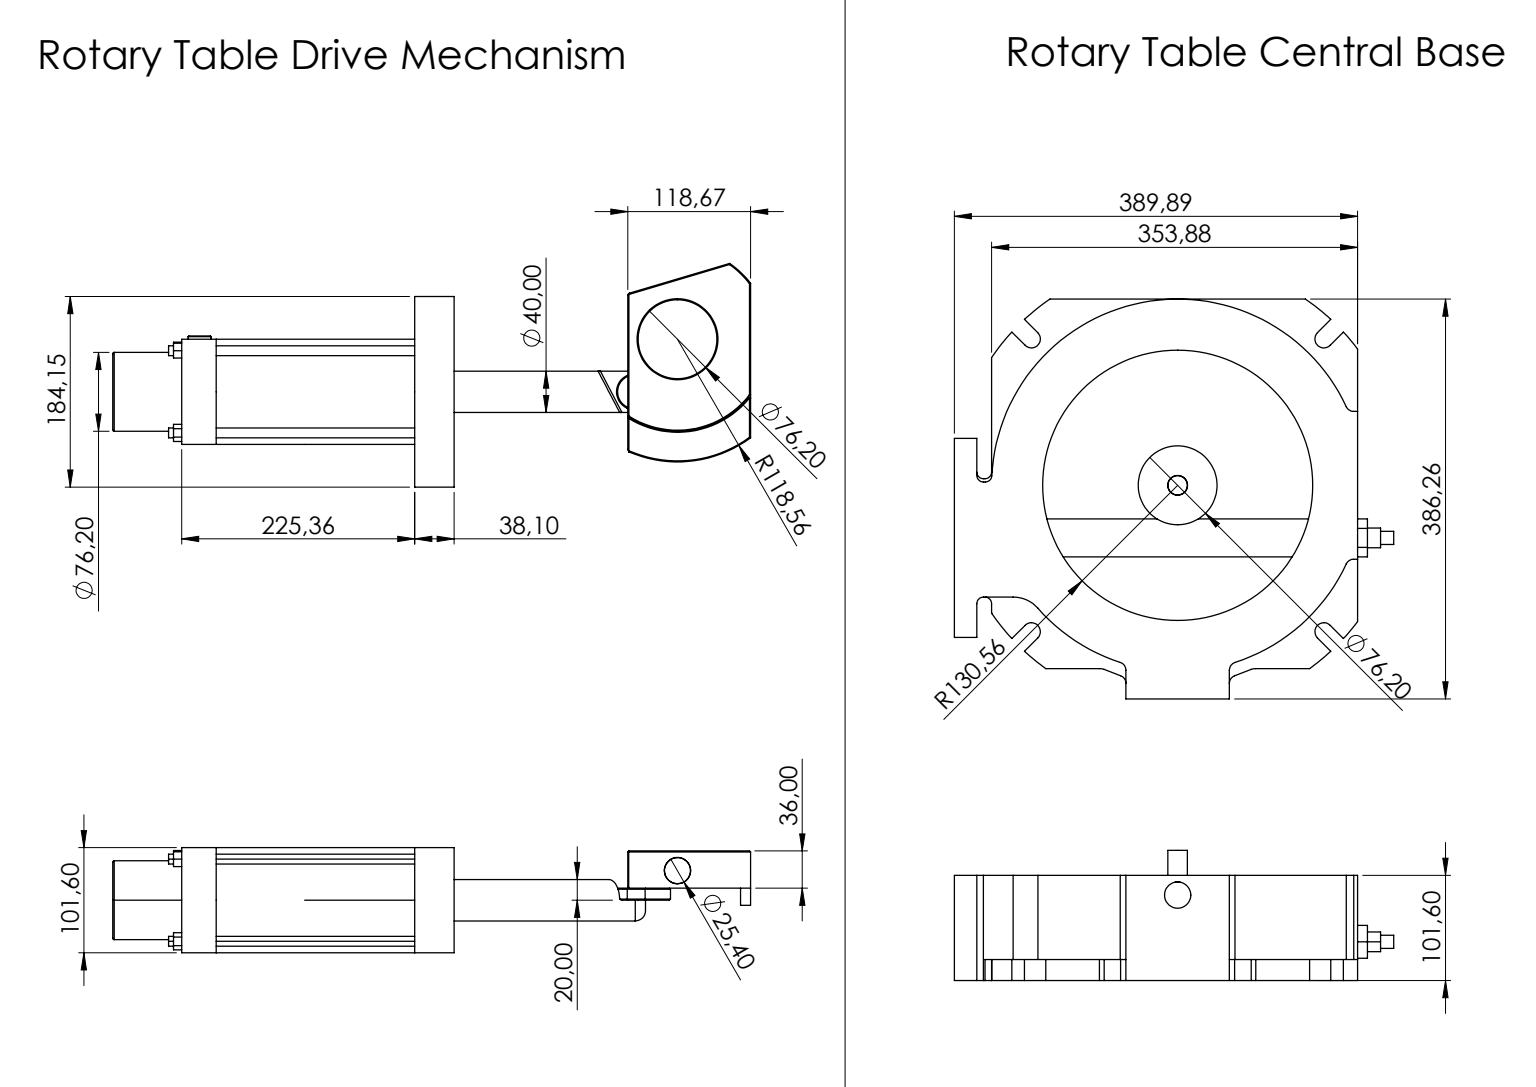
ISO-10303-21;
HEADER;
FILE_DESCRIPTION (('STEP AP214'),
    '1' );
FILE_NAME ('Rotary Table Central Base.step',
    '2026-10-07T11:37:37',
    ( '' ),
    ( '' ),
    'SwSTEP 2.0',
    'SolidWorks 2020',
    '' );
FILE_SCHEMA (( 'AUTOMOTIVE_DESIGN' ));
ENDSEC;

DATA;
#6=CARTESIAN_POINT ( 'NONE',  ( 55.11501535284990183, 101.5999999999999943, 183.9403141659174992 ) ) ;
#9=CARTESIAN_POINT ( 'NONE',  ( 9.168977498726896158, 73.76155057898466794, 130.2336791939843295 ) ) ;
#14=CARTESIAN_POINT ( 'NONE',  ( -194.1576000000000022, 0.000000000000000000, -12.69999999999999929 ) ) ;
#21=ORIENTED_EDGE ( 'NONE', *, *, #73612, .F. ) ;
#33=ORIENTED_EDGE ( 'NONE', *, *, #1736, .F. ) ;
#55=ORIENTED_EDGE ( 'NONE', *, *, #81296, .T. ) ;
#58=DIRECTION ( 'NONE',  ( 0.000000000000000000, -1.000000000000000000, 0.000000000000000000 ) ) ;
#67=DIRECTION ( 'NONE',  ( 0.000000000000000000, -1.000000000000000000, 0.000000000000000000 ) ) ;
#73=FACE_OUTER_BOUND ( 'NONE', #27829, .T. ) ;
#85=DIRECTION ( 'NONE',  ( 0.000000000000000000, 0.000000000000000000, -1.000000000000000000 ) ) ;
#88=CARTESIAN_POINT ( 'NONE',  ( 57.91199999999999903, 20.32000000000000028, 178.6098374884404905 ) ) ;
#95=ORIENTED_EDGE ( 'NONE', *, *, #27973, .F. ) ;
#121=VERTEX_POINT ( 'NONE', #20268 ) ;
#132=VECTOR ( 'NONE', #74907, 1000.000000000000000 ) ;
#135=DIRECTION ( 'NONE',  ( 0.000000000000000000, -1.000000000000000000, 0.000000000000000000 ) ) ;
#144=CARTESIAN_POINT ( 'NONE',  ( 1.925672578516905147E-22, 69.84999999999999432, 130.5560000000000116 ) ) ;
#191=EDGE_CURVE ( 'NONE', #23949, #76533, #47936, .T. ) ;
#205=FACE_OUTER_BOUND ( 'NONE', #10836, .T. ) ;
#234=CARTESIAN_POINT ( 'NONE',  ( -118.6305646578576045, 74.28520294732120988, 54.51736277023807986 ) ) ;
#242=EDGE_CURVE ( 'NONE', #42621, #19042, #11659, .T. ) ;
#255=EDGE_LOOP ( 'NONE', ( #36658, #16819, #37232, #21617 ) ) ;
#262=CARTESIAN_POINT ( 'NONE',  ( 50.03799999999999670, 101.5999999999999943, 206.3750000000000000 ) ) ;
#265=CARTESIAN_POINT ( 'NONE',  ( -6.586072245893089594, 71.69064597417980167, 130.3897833686264676 ) ) ;
#267=DIRECTION ( 'NONE',  ( 0.000000000000000000, 0.000000000000000000, 1.000000000000000000 ) ) ;
#269=LINE ( 'NONE', #28879, #27362 ) ;
#284=FACE_OUTER_BOUND ( 'NONE', #2553, .T. ) ;
#309=ORIENTED_EDGE ( 'NONE', *, *, #18028, .F. ) ;
#321=LINE ( 'NONE', #15311, #8132 ) ;
#341=CARTESIAN_POINT ( 'NONE',  ( -179.8898777604655095, 101.5999999999999943, 114.2999999999999972 ) ) ;
#345=ORIENTED_EDGE ( 'NONE', *, *, #9906, .F. ) ;
#365=EDGE_CURVE ( 'NONE', #79893, #74303, #7526, .T. ) ;
#369=DIRECTION ( 'NONE',  ( 0.000000000000000000, 0.000000000000000000, 1.000000000000000000 ) ) ;
#371=FACE_OUTER_BOUND ( 'NONE', #73680, .T. ) ;
#378=VERTEX_POINT ( 'NONE', #7971 ) ;
#402=CARTESIAN_POINT ( 'NONE',  ( 0.000000000000000000, 8.255000000000000782, 0.000000000000000000 ) ) ;
#409=ADVANCED_FACE ( 'NONE', ( #6043 ), #47786, .F. ) ;
#412=ORIENTED_EDGE ( 'NONE', *, *, #13605, .T. ) ;
#418=LINE ( 'NONE', #69017, #71892 ) ;
#419=VECTOR ( 'NONE', #36946, 1000.000000000000000 ) ;
#424=EDGE_CURVE ( 'NONE', #58432, #84394, #41641, .T. ) ;
#436=ORIENTED_EDGE ( 'NONE', *, *, #26526, .T. ) ;
#447=DIRECTION ( 'NONE',  ( 0.000000000000000000, 1.000000000000000000, 0.000000000000000000 ) ) ;
#456=CARTESIAN_POINT ( 'NONE',  ( 120.0602177517065314, 48.67389603571125178, -51.28856941560783866 ) ) ;
#459=ORIENTED_EDGE ( 'NONE', *, *, #13256, .F. ) ;
#461=EDGE_CURVE ( 'NONE', #89089, #79893, #19649, .T. ) ;
#493=ORIENTED_EDGE ( 'NONE', *, *, #28288, .T. ) ;
#509=PLANE ( 'NONE',  #44376 ) ;
#523=FACE_OUTER_BOUND ( 'NONE', #41384, .T. ) ;
#534=AXIS2_PLACEMENT_3D ( 'NONE', #54365, #54819, #13078 ) ;
#537=AXIS2_PLACEMENT_3D ( 'NONE', #14393, #82553, #62968 ) ;
#572=CARTESIAN_POINT ( 'NONE',  ( -187.8075999999999794, 20.32000000000000028, -12.69999999999999929 ) ) ;
#599=CARTESIAN_POINT ( 'NONE',  ( 11.42157353567683842, 76.98139724742750900, 130.0556313956597592 ) ) ;
#635=DIRECTION ( 'NONE',  ( 1.000000000000000000, 0.000000000000000000, 0.000000000000000000 ) ) ;
#639=ORIENTED_EDGE ( 'NONE', *, *, #3250, .F. ) ;
#656=LINE ( 'NONE', #28362, #8199 ) ;
#675=LINE ( 'NONE', #22483, #55023 ) ;
#679=ORIENTED_EDGE ( 'NONE', *, *, #28156, .T. ) ;
#681=CARTESIAN_POINT ( 'NONE',  ( -114.0590328520549832, 70.22562679785821160, 63.52550556333007137 ) ) ;
#684=CARTESIAN_POINT ( 'NONE',  ( -127.5252020268932114, 20.32000000000000028, 177.0380000000000109 ) ) ;
#710=DIRECTION ( 'NONE',  ( 0.000000000000000000, -1.000000000000000000, 0.000000000000000000 ) ) ;
#723=CARTESIAN_POINT ( 'NONE',  ( 0.000000000000000000, 101.5999999999999943, 0.000000000000000000 ) ) ;
#730=CARTESIAN_POINT ( 'NONE',  ( 0.000000000000000000, 0.000000000000000000, 0.000000000000000000 ) ) ;
#754=ORIENTED_EDGE ( 'NONE', *, *, #13256, .T. ) ;
#766=CARTESIAN_POINT ( 'NONE',  ( -11.74378193249606106, 87.38464304823123996, 130.0267385514075329 ) ) ;
#820=CARTESIAN_POINT ( 'NONE',  ( 23.04101804865160119, 56.72370184857491182, 30.34351131950213798 ) ) ;
#849=VERTEX_POINT ( 'NONE', #62748 ) ;
#879=VECTOR ( 'NONE', #87402, 1000.000000000000000 ) ;
#903=LINE ( 'NONE', #51260, #75514 ) ;
#910=CARTESIAN_POINT ( 'NONE',  ( 121.8078998857219375, 45.20015392834827850, -46.98888152329894297 ) ) ;
#924=DIRECTION ( 'NONE',  ( 1.000000000000000000, 0.000000000000000000, -7.340987889507870014E-14 ) ) ;
#940=CARTESIAN_POINT ( 'NONE',  ( 122.6197261538189593, 73.74150706513661646, 44.83011014023653473 ) ) ;
#969=EDGE_CURVE ( 'NONE', #72419, #64336, #76549, .T. ) ;
#991=EDGE_CURVE ( 'NONE', #50564, #38934, #59391, .T. ) ;
#1000=FACE_OUTER_BOUND ( 'NONE', #74644, .T. ) ;
#1051=CIRCLE ( 'NONE', #41678, 218.1859999999999786 ) ;
#1054=AXIS2_PLACEMENT_3D ( 'NONE', #30838, #23597, #85383 ) ;
#1058=PLANE ( 'NONE',  #80794 ) ;
#1080=ORIENTED_EDGE ( 'NONE', *, *, #12504, .T. ) ;
#1099=EDGE_LOOP ( 'NONE', ( #50497, #23649, #64387, #74455 ) ) ;
#1137=CIRCLE ( 'NONE', #51867, 218.1859999999999786 ) ;
#1144=CARTESIAN_POINT ( 'NONE',  ( -125.2622172144571522, 69.13895712999180887, 36.80031982249843026 ) ) ;
#1162=VERTEX_POINT ( 'NONE', #12156 ) ;
#1196=CARTESIAN_POINT ( 'NONE',  ( 0.000000000000000000, 0.000000000000000000, 0.000000000000000000 ) ) ;
#1214=AXIS2_PLACEMENT_3D ( 'NONE', #4908, #60752, #6253 ) ;
#1273=FACE_OUTER_BOUND ( 'NONE', #73997, .T. ) ;
#1274=CARTESIAN_POINT ( 'NONE',  ( 173.9900000000000091, 20.32000000000000028, 71.37400000000000944 ) ) ;
#1291=CYLINDRICAL_SURFACE ( 'NONE', #89725, 25.39999999999999858 ) ;
#1300=CARTESIAN_POINT ( 'NONE',  ( 141.3509999999999991, 0.000000000000000000, -141.3509999999999991 ) ) ;
#1331=ORIENTED_EDGE ( 'NONE', *, *, #52309, .T. ) ;
#1354=CARTESIAN_POINT ( 'NONE',  ( 131.3179999999999836, 53.97500000000000142, 50.79999999999999716 ) ) ;
#1365=CARTESIAN_POINT ( 'NONE',  ( 122.3663862029045504, 44.85577228901693303, -45.51497792402615516 ) ) ;
#1372=CARTESIAN_POINT ( 'NONE',  ( -186.2398777604655038, 20.32000000000000028, -6.349999999999999645 ) ) ;
#1374=DIRECTION ( 'NONE',  ( 0.000000000000000000, 1.000000000000000000, 0.000000000000000000 ) ) ;
#1384=VECTOR ( 'NONE', #24697, 1000.000000000000000 ) ;
#1393=CARTESIAN_POINT ( 'NONE',  ( 124.9987061611030299, 69.92834781287285750, 37.68974897191494478 ) ) ;
#1408=CIRCLE ( 'NONE', #11581, 7.937500000000000000 ) ;
#1428=LINE ( 'NONE', #77732, #37903 ) ;
#1476=ORIENTED_EDGE ( 'NONE', *, *, #57990, .F. ) ;
#1508=VECTOR ( 'NONE', #40924, 1000.000000000000000 ) ;
#1538=EDGE_CURVE ( 'NONE', #50564, #46362, #46531, .T. ) ;
#1547=DIRECTION ( 'NONE',  ( 0.000000000000000000, -1.000000000000000000, 0.000000000000000000 ) ) ;
#1579=VECTOR ( 'NONE', #24525, 1000.000000000000000 ) ;
#1593=LINE ( 'NONE', #33068, #83246 ) ;
#1603=EDGE_LOOP ( 'NONE', ( #84238, #42439, #85968, #88448, #51749, #46852, #88301, #60459, #68291, #59099, #73730, #61079, #86150, #31030, #81684, #69215, #63173, #39550, #87001, #53196, #28094, #73403, #88949, #30386 ) ) ;
#1625=TOROIDAL_SURFACE ( 'NONE', #36441, 154.1697486074984909, 6.349999999999999645 ) ;
#1662=ORIENTED_EDGE ( 'NONE', *, *, #34458, .T. ) ;
#1664=DIRECTION ( 'NONE',  ( 0.000000000000000000, -1.000000000000000000, 0.000000000000000000 ) ) ;
#1665=AXIS2_PLACEMENT_3D ( 'NONE', #30439, #29996, #84972 ) ;
#1728=CARTESIAN_POINT ( 'NONE',  ( 5.483693934069210130, 69.93014865207605624, 37.70952975325106848 ) ) ;
#1730=DIRECTION ( 'NONE',  ( 0.000000000000000000, -1.000000000000000000, 0.000000000000000000 ) ) ;
#1732=DIRECTION ( 'NONE',  ( -0.000000000000000000, 1.000000000000000000, -0.000000000000000000 ) ) ;
#1736=EDGE_CURVE ( 'NONE', #19136, #23399, #48323, .T. ) ;
#1772=AXIS2_PLACEMENT_3D ( 'NONE', #8531, #21718, #42565 ) ;
#1777=VECTOR ( 'NONE', #19377, 1000.000000000000000 ) ;
#1806=DIRECTION ( 'NONE',  ( 1.000000000000000000, 0.000000000000000000, 0.000000000000000000 ) ) ;
#1839=DIRECTION ( 'NONE',  ( 0.000000000000000000, 0.000000000000000000, 1.000000000000000000 ) ) ;
#1842=AXIS2_PLACEMENT_3D ( 'NONE', #41040, #67400, #66965 ) ;
#1844=CARTESIAN_POINT ( 'NONE',  ( 123.4547429832808945, 72.86362559908033631, 42.47335031276299588 ) ) ;
#1855=ORIENTED_EDGE ( 'NONE', *, *, #32760, .T. ) ;
#1900=CARTESIAN_POINT ( 'NONE',  ( 135.2444258376725941, 20.32000000000000028, 147.4575741623265799 ) ) ;
#1925=CARTESIAN_POINT ( 'NONE',  ( 50.03799999999999670, 20.32000000000000028, 178.6098374884404905 ) ) ;
#1957=CYLINDRICAL_SURFACE ( 'NONE', #84880, 6.349999999999994316 ) ;
#1960=CARTESIAN_POINT ( 'NONE',  ( 11.75171833347117811, 77.73468025497935230, 130.0260221836642813 ) ) ;
#1984=EDGE_LOOP ( 'NONE', ( #10043, #68745, #95, #71951, #82324, #55575 ) ) ;
#2041=CARTESIAN_POINT ( 'NONE',  ( -126.8825202696031198, 58.88652527941982129, 30.75229511181026609 ) ) ;
#2056=CYLINDRICAL_SURFACE ( 'NONE', #89128, 12.69999999999999929 ) ;
#2074=DIRECTION ( 'NONE',  ( 0.000000000000000000, -1.000000000000000000, 0.000000000000000000 ) ) ;
#2092=AXIS2_PLACEMENT_3D ( 'NONE', #19499, #34808, #8462 ) ;
#2178=CARTESIAN_POINT ( 'NONE',  ( 0.000000000000000000, 2.269999999999994245, 0.000000000000000000 ) ) ;
#2186=CARTESIAN_POINT ( 'NONE',  ( 173.9900000000000091, 21.46300000000000097, 41.63456447661474868 ) ) ;
#2198=DIRECTION ( 'NONE',  ( 0.000000000000000000, 0.000000000000000000, 1.000000000000000000 ) ) ;
#2213=VERTEX_POINT ( 'NONE', #41413 ) ;
#2238=DIRECTION ( 'NONE',  ( 0.000000000000000000, -1.000000000000000000, 0.000000000000000000 ) ) ;
#2241=VECTOR ( 'NONE', #42500, 1000.000000000000000 ) ;
#2242=EDGE_LOOP ( 'NONE', ( #82053, #59237, #69794, #15889 ) ) ;
#2281=CARTESIAN_POINT ( 'NONE',  ( -12.69999999999999929, 82.54999999999999716, 129.9368274816650057 ) ) ;
#2286=EDGE_CURVE ( 'NONE', #58230, #18059, #63217, .T. ) ;
#2292=CARTESIAN_POINT ( 'NONE',  ( 126.3208227659863638, 64.39779484612361671, 32.98409395337385064 ) ) ;
#2307=ORIENTED_EDGE ( 'NONE', *, *, #46424, .T. ) ;
#2310=AXIS2_PLACEMENT_3D ( 'NONE', #35040, #41840, #85017 ) ;
#2313=CIRCLE ( 'NONE', #50193, 8.636000000000004562 ) ;
#2395=ORIENTED_EDGE ( 'NONE', *, *, #26112, .F. ) ;
#2400=AXIS2_PLACEMENT_3D ( 'NONE', #64029, #1806, #29505 ) ;
#2401=DIRECTION ( 'NONE',  ( 0.000000000000000000, -1.000000000000000000, 0.000000000000000000 ) ) ;
#2458=DIRECTION ( 'NONE',  ( 0.000000000000000000, 1.000000000000000000, 0.000000000000000000 ) ) ;
#2468=EDGE_CURVE ( 'NONE', #11178, #18383, #21790, .T. ) ;
#2473=DIRECTION ( 'NONE',  ( -0.000000000000000000, 1.000000000000000000, 0.000000000000000000 ) ) ;
#2506=CARTESIAN_POINT ( 'NONE',  ( 71.09939861440099662, 20.32000000000000028, 177.8662485265279827 ) ) ;
#2508=ORIENTED_EDGE ( 'NONE', *, *, #15756, .F. ) ;
#2533=EDGE_CURVE ( 'NONE', #69150, #57574, #33384, .T. ) ;
#2541=LINE ( 'NONE', #8919, #2241 ) ;
#2550=ORIENTED_EDGE ( 'NONE', *, *, #83461, .F. ) ;
#2553=EDGE_LOOP ( 'NONE', ( #85925, #24242, #36675, #80564 ) ) ;
#2573=CARTESIAN_POINT ( 'NONE',  ( -6.676094946653681639, 93.36325093810603448, 130.3857439148796686 ) ) ;
#2617=CIRCLE ( 'NONE', #35929, 25.39999999999999858 ) ;
#2625=FACE_OUTER_BOUND ( 'NONE', #55968, .T. ) ;
#2688=CARTESIAN_POINT ( 'NONE',  ( 0.000000000000000000, 44.45000000000000284, 0.000000000000000000 ) ) ;
#2714=AXIS2_PLACEMENT_3D ( 'NONE', #31294, #58989, #11763 ) ;
#2739=CARTESIAN_POINT ( 'NONE',  ( 126.5345833325615104, 62.85051826981599987, 32.15513509386430258 ) ) ;
#2756=VERTEX_POINT ( 'NONE', #38518 ) ;
#2765=AXIS2_PLACEMENT_3D ( 'NONE', #7711, #28138, #27706 ) ;
#2785=CARTESIAN_POINT ( 'NONE',  ( 196.2150000000000034, 43.68799999999999528, 44.45000000000000284 ) ) ;
#2805=LINE ( 'NONE', #73162, #20065 ) ;
#2809=AXIS2_PLACEMENT_3D ( 'NONE', #64440, #50346, #78085 ) ;
#2810=FACE_OUTER_BOUND ( 'NONE', #61011, .T. ) ;
#2850=CARTESIAN_POINT ( 'NONE',  ( -135.2444258376732193, 101.5999999999999943, -147.4575741623275746 ) ) ;
#2904=LINE ( 'NONE', #44660, #11603 ) ;
#2914=AXIS2_PLACEMENT_3D ( 'NONE', #18645, #74054, #60409 ) ;
#2916=CARTESIAN_POINT ( 'NONE',  ( 3.174999999999879918, 17.78000000000000114, -33.98325472291465132 ) ) ;
#2945=DIRECTION ( 'NONE',  ( 0.000000000000000000, -1.000000000000000000, 0.000000000000000000 ) ) ;
#2957=LINE ( 'NONE', #11095, #63039 ) ;
#2965=ADVANCED_FACE ( 'NONE', ( #4242 ), #69374, .F. ) ;
#2975=PLANE ( 'NONE',  #30037 ) ;
#3011=EDGE_LOOP ( 'NONE', ( #54618, #26924, #77400, #78953 ) ) ;
#3013=CARTESIAN_POINT ( 'NONE',  ( 126.6062568295380260, 45.75147977268651545, 31.87055648571903532 ) ) ;
#3014=DIRECTION ( 'NONE',  ( 0.000000000000000000, 0.000000000000000000, 1.000000000000000000 ) ) ;
#3028=EDGE_CURVE ( 'NONE', #64725, #32634, #70806, .T. ) ;
#3039=AXIS2_PLACEMENT_3D ( 'NONE', #66814, #19562, #39106 ) ;
#3040=ORIENTED_EDGE ( 'NONE', *, *, #50901, .T. ) ;
#3070=LINE ( 'NONE', #30333, #46669 ) ;
#3088=FACE_OUTER_BOUND ( 'NONE', #30243, .T. ) ;
#3102=CARTESIAN_POINT ( 'NONE',  ( 173.9900000000000091, 20.32000000000000028, 71.37400000000000944 ) ) ;
#3105=ORIENTED_EDGE ( 'NONE', *, *, #42203, .F. ) ;
#3156=DIRECTION ( 'NONE',  ( 0.000000000000000000, -1.000000000000000000, 0.000000000000000000 ) ) ;
#3168=CIRCLE ( 'NONE', #78661, 12.69999999999999929 ) ;
#3173=DIRECTION ( 'NONE',  ( 0.000000000000000000, 0.000000000000000000, 1.000000000000000000 ) ) ;
#3181=CARTESIAN_POINT ( 'NONE',  ( 111.1294417335836044, 64.57244353077730636, 68.52200795564769464 ) ) ;
#3190=AXIS2_PLACEMENT_3D ( 'NONE', #44429, #24903, #23581 ) ;
#3191=EDGE_CURVE ( 'NONE', #23399, #67629, #41787, .T. ) ;
#3204=CARTESIAN_POINT ( 'NONE',  ( -55.48342271751670296, 20.32000000000000028, 171.1197181046785261 ) ) ;
#3209=LINE ( 'NONE', #30019, #61414 ) ;
#3210=VECTOR ( 'NONE', #26083, 1000.000000000000000 ) ;
#3216=EDGE_CURVE ( 'NONE', #74303, #21031, #48681, .T. ) ;
#3250=EDGE_CURVE ( 'NONE', #25538, #23113, #65902, .T. ) ;
#3256=DIRECTION ( 'NONE',  ( 0.000000000000000000, 1.000000000000000000, 0.000000000000000000 ) ) ;
#3265=CIRCLE ( 'NONE', #72887, 9.425000000000000711 ) ;
#3274=EDGE_LOOP ( 'NONE', ( #29356, #25141, #17679, #23241 ) ) ;
#3276=CARTESIAN_POINT ( 'NONE',  ( 0.000000000000000000, 114.2999999999999972, 0.000000000000000000 ) ) ;
#3279=ORIENTED_EDGE ( 'NONE', *, *, #89079, .T. ) ;
#3323=CARTESIAN_POINT ( 'NONE',  ( 6.966821914208871647, 93.16860575031896019, 130.3699860581843382 ) ) ;
#3393=EDGE_CURVE ( 'NONE', #60724, #64884, #18658, .T. ) ;
#3398=AXIS2_PLACEMENT_3D ( 'NONE', #24982, #52649, #18157 ) ;
#3424=DIRECTION ( 'NONE',  ( 0.000000000000000000, -1.000000000000000000, 0.000000000000000000 ) ) ;
#3442=AXIS2_PLACEMENT_3D ( 'NONE', #11677, #66625, #40255 ) ;
#3445=CARTESIAN_POINT ( 'NONE',  ( 196.2150000000000034, 37.33800000000000097, 50.79999999999999716 ) ) ;
#3446=AXIS2_PLACEMENT_3D ( 'NONE', #51287, #18570, #3173 ) ;
#3452=CARTESIAN_POINT ( 'NONE',  ( -7.303152832728717847, 92.94038696238578723, 130.3515497892399821 ) ) ;
#3454=ORIENTED_EDGE ( 'NONE', *, *, #53244, .F. ) ;
#3458=CARTESIAN_POINT ( 'NONE',  ( -158.9822249764580135, 20.32000000000000028, 107.9500000000000028 ) ) ;
#3493=AXIS2_PLACEMENT_3D ( 'NONE', #36604, #29780, #57471 ) ;
#3517=LINE ( 'NONE', #31217, #34566 ) ;
#3523=EDGE_CURVE ( 'NONE', #55364, #65449, #59232, .T. ) ;
#3534=DIRECTION ( 'NONE',  ( 0.000000000000000000, 1.000000000000000000, 0.000000000000000000 ) ) ;
#3554=CARTESIAN_POINT ( 'NONE',  ( 173.9900000000000091, 37.33800000000000097, 32.46912895322940074 ) ) ;
#3576=DIRECTION ( 'NONE',  ( 0.000000000000000000, -1.000000000000000000, 0.000000000000000000 ) ) ;
#3583=AXIS2_PLACEMENT_3D ( 'NONE', #26369, #33633, #89501 ) ;
#3603=FACE_OUTER_BOUND ( 'NONE', #9763, .T. ) ;
#3613=CARTESIAN_POINT ( 'NONE',  ( 117.1417030460440003, 73.45442465866868531, 57.64679522113551968 ) ) ;
#3636=EDGE_CURVE ( 'NONE', #45956, #11616, #5573, .T. ) ;
#3666=VERTEX_POINT ( 'NONE', #43106 ) ;
#3675=CARTESIAN_POINT ( 'NONE',  ( 183.5150000000000148, 21.46300000000000097, 59.96543552338529537 ) ) ;
#3676=CARTESIAN_POINT ( 'NONE',  ( 0.000000000000000000, 8.255000000000000782, 0.000000000000000000 ) ) ;
#3685=FILL_AREA_STYLE ('',( #37767 ) ) ;
#3686=DIRECTION ( 'NONE',  ( -1.000000000000000000, 0.000000000000000000, 0.000000000000000000 ) ) ;
#3692=LINE ( 'NONE', #31384, #19527 ) ;
#3707=EDGE_LOOP ( 'NONE', ( #12509, #31854, #37787, #38344 ) ) ;
#3714=ORIENTED_EDGE ( 'NONE', *, *, #48510, .F. ) ;
#3723=ORIENTED_EDGE ( 'NONE', *, *, #17531, .F. ) ;
#3743=CARTESIAN_POINT ( 'NONE',  ( -50.03799999999999670, 101.5999999999999943, 206.3750000000000000 ) ) ;
#3756=EDGE_CURVE ( 'NONE', #84589, #44354, #49476, .T. ) ;
#3763=CARTESIAN_POINT ( 'NONE',  ( 4.048368076483533251, 94.58941606601858609, 130.4932642680670654 ) ) ;
#3798=EDGE_CURVE ( 'NONE', #74769, #67371, #6811, .T. ) ;
#3841=CARTESIAN_POINT ( 'NONE',  ( -8.813809904571851206, 69.38616896394334788, 37.07268381226281662 ) ) ;
#3851=CARTESIAN_POINT ( 'NONE',  ( 0.000000000000000000, 17.78000000000000114, 0.000000000000000000 ) ) ;
#3859=EDGE_CURVE ( 'NONE', #24397, #60648, #74883, .T. ) ;
#3869=DIRECTION ( 'NONE',  ( 0.000000000000000000, 0.000000000000000000, 1.000000000000000000 ) ) ;
#3893=CARTESIAN_POINT ( 'NONE',  ( -10.40475206047886836, 89.83749360592842947, 130.1408237963791805 ) ) ;
#3902=EDGE_CURVE ( 'NONE', #43122, #1162, #15882, .T. ) ;
#3911=DIRECTION ( 'NONE',  ( 0.000000000000000000, 0.000000000000000000, 1.000000000000000000 ) ) ;
#3923=ADVANCED_FACE ( 'NONE', ( #86704 ), #10832, .F. ) ;
#3992=VECTOR ( 'NONE', #27514, 1000.000000000000000 ) ;
#4013=CARTESIAN_POINT ( 'NONE',  ( 119.5843592605237120, 53.27973259447988141, -52.38750000000000995 ) ) ;
#4030=AXIS2_PLACEMENT_3D ( 'NONE', #44635, #64216, #64650 ) ;
#4034=ORIENTED_EDGE ( 'NONE', *, *, #12569, .F. ) ;
#4035=CARTESIAN_POINT ( 'NONE',  ( -3.175000000000120171, 17.78000000000000114, -33.98325472291465132 ) ) ;
#4046=VECTOR ( 'NONE', #67580, 1000.000000000000000 ) ;
#4048=CYLINDRICAL_SURFACE ( 'NONE', #52014, 31.75000000000000000 ) ;
#4053=LINE ( 'NONE', #12215, #21138 ) ;
#4060=CARTESIAN_POINT ( 'NONE',  ( 112.1769819967410768, 67.02335788169725106, 66.79262069672253688 ) ) ;
#4065=DIRECTION ( 'NONE',  ( 1.000000000000000000, -0.000000000000000000, 2.108231265501709878E-16 ) ) ;
#4085=DIRECTION ( 'NONE',  ( 0.000000000000000000, 0.000000000000000000, 1.000000000000000000 ) ) ;
#4096=VECTOR ( 'NONE', #56793, 1000.000000000000000 ) ;
#4120=ORIENTED_EDGE ( 'NONE', *, *, #22845, .F. ) ;
#4151=EDGE_LOOP ( 'NONE', ( #9354, #88619 ) ) ;
#4177=VERTEX_POINT ( 'NONE', #89392 ) ;
#4196=DIRECTION ( 'NONE',  ( -1.000000000000000000, 0.000000000000000000, -1.840813417405305102E-14 ) ) ;
#4209=CARTESIAN_POINT ( 'NONE',  ( 7.283224538747764321, 92.95786475339244248, 130.3529002834609969 ) ) ;
#4239=DIRECTION ( 'NONE',  ( 0.7071067811865604513, 0.000000000000000000, -0.7071067811865344721 ) ) ;
#4242=FACE_OUTER_BOUND ( 'NONE', #42519, .T. ) ;
#4249=LINE ( 'NONE', #18318, #38584 ) ;
#4261=EDGE_LOOP ( 'NONE', ( #57389, #30712 ) ) ;
#4286=AXIS2_PLACEMENT_3D ( 'NONE', #3445, #51574, #78876 ) ;
#4293=CARTESIAN_POINT ( 'NONE',  ( -6.832456821293724225, 69.76561602091111070, 37.50674678103825244 ) ) ;
#4300=LINE ( 'NONE', #30664, #24978 ) ;
#4301=FACE_OUTER_BOUND ( 'NONE', #13829, .T. ) ;
#4318=DIRECTION ( 'NONE',  ( -1.514143847546114723E-15, -0.8660254037844387076, 0.4999999999999998890 ) ) ;
#4330=DIRECTION ( 'NONE',  ( -2.108231265501709878E-16, 0.000000000000000000, 1.000000000000000000 ) ) ;
#4338=ORIENTED_EDGE ( 'NONE', *, *, #33616, .F. ) ;
#4340=ADVANCED_FACE ( 'NONE', ( #64368 ), #37554, .F. ) ;
#4348=CARTESIAN_POINT ( 'NONE',  ( 173.9900000000000091, 0.000000000000000000, -131.6533725204182019 ) ) ;
#4360=ADVANCED_FACE ( 'NONE', ( #16659 ), #51160, .F. ) ;
#4368=ORIENTED_EDGE ( 'NONE', *, *, #69515, .F. ) ;
#4376=CARTESIAN_POINT ( 'NONE',  ( -109.3711719371063822, 56.43282072966933072, 71.29388279269264217 ) ) ;
#4442=ORIENTED_EDGE ( 'NONE', *, *, #82573, .T. ) ;
#4491=CARTESIAN_POINT ( 'NONE',  ( 173.9900000000000091, 101.5999999999999943, 71.37400000000000944 ) ) ;
#4513=CARTESIAN_POINT ( 'NONE',  ( 122.0810025972884034, 74.11507855671040090, 46.27428068823228813 ) ) ;
#4547=FACE_OUTER_BOUND ( 'NONE', #43550, .T. ) ;
#4549=ORIENTED_EDGE ( 'NONE', *, *, #3250, .T. ) ;
#4573=VERTEX_POINT ( 'NONE', #38874 ) ;
#4578=ORIENTED_EDGE ( 'NONE', *, *, #49606, .F. ) ;
#4634=FACE_OUTER_BOUND ( 'NONE', #56633, .T. ) ;
#4656=CARTESIAN_POINT ( 'NONE',  ( 7.043515244065597258, 93.11782407023925145, 130.3658622353028136 ) ) ;
#4664=AXIS2_PLACEMENT_3D ( 'NONE', #75186, #6153, #39312 ) ;
#4711=CARTESIAN_POINT ( 'NONE',  ( 147.4575741623270062, 101.5999999999999943, -135.2444258376734183 ) ) ;
#4719=CARTESIAN_POINT ( 'NONE',  ( -57.91199999999999903, 20.32000000000000028, 178.6098374884404905 ) ) ;
#4728=DIRECTION ( 'NONE',  ( 0.000000000000000000, -1.000000000000000000, 0.000000000000000000 ) ) ;
#4769=CARTESIAN_POINT ( 'NONE',  ( 21.73093249848547259, 47.21781368078172392, 31.29576654108570111 ) ) ;
#4778=CYLINDRICAL_SURFACE ( 'NONE', #24444, 9.524999999999998579 ) ;
#4786=PLANE ( 'NONE',  #18166 ) ;
#4800=CARTESIAN_POINT ( 'NONE',  ( 126.6659102797931808, 46.32248961978775981, 31.63262298343003920 ) ) ;
#4818=CARTESIAN_POINT ( 'NONE',  ( -109.4150722537221867, 56.95621006804009312, 71.22652974919590463 ) ) ;
#4822=ORIENTED_EDGE ( 'NONE', *, *, #21901, .F. ) ;
#4846=PLANE ( 'NONE',  #69282 ) ;
#4849=FACE_OUTER_BOUND ( 'NONE', #37716, .T. ) ;
#4853=EDGE_LOOP ( 'NONE', ( #37804, #41543, #10759, #75209 ) ) ;
#4875=ADVANCED_FACE ( 'NONE', ( #88308 ), #54626, .F. ) ;
#4888=CIRCLE ( 'NONE', #534, 24.63800000000000168 ) ;
#4898=PLANE ( 'NONE',  #8627 ) ;
#4908=CARTESIAN_POINT ( 'NONE',  ( 0.000000000000000000, 44.45000000000000284, 0.000000000000000000 ) ) ;
#4912=CARTESIAN_POINT ( 'NONE',  ( 125.2832873508473455, 54.59514987206014069, -36.72832927292047600 ) ) ;
#4938=DIRECTION ( 'NONE',  ( -1.000000000000000000, 0.000000000000000000, 3.491483361109380094E-15 ) ) ;
#4943=VERTEX_POINT ( 'NONE', #5171 ) ;
#4950=VECTOR ( 'NONE', #1730, 1000.000000000000000 ) ;
#4956=CARTESIAN_POINT ( 'NONE',  ( 120.5244058523157662, 74.60816462893807000, 50.18922276370457780 ) ) ;
#4962=AXIS2_PLACEMENT_3D ( 'NONE', #65180, #44719, #65621 ) ;
#4965=EDGE_LOOP ( 'NONE', ( #19056, #80784, #40633, #54726, #43123 ) ) ;
#4968=ORIENTED_EDGE ( 'NONE', *, *, #80762, .F. ) ;
#4980=EDGE_CURVE ( 'NONE', #64268, #63182, #88670, .T. ) ;
#4997=CARTESIAN_POINT ( 'NONE',  ( -71.09939861440099662, 101.5999999999999943, 177.8662485265279827 ) ) ;
#5009=CARTESIAN_POINT ( 'NONE',  ( 173.9900000000000091, 20.32000000000000028, 71.37400000000000944 ) ) ;
#5010=AXIS2_PLACEMENT_3D ( 'NONE', #56810, #14607, #41387 ) ;
#5042=CARTESIAN_POINT ( 'NONE',  ( -123.4696824136392053, 20.32000000000000028, -179.8898777604655095 ) ) ;
#5053=EDGE_CURVE ( 'NONE', #31466, #21936, #69233, .T. ) ;
#5058=VECTOR ( 'NONE', #74347, 1000.000000000000000 ) ;
#5070=CARTESIAN_POINT ( 'NONE',  ( 108.8673596973266058, 37.33800000000000097, 58.73749999999999716 ) ) ;
#5081=DIRECTION ( 'NONE',  ( -1.000000000000000000, 0.000000000000000000, 0.000000000000000000 ) ) ;
#5104=CARTESIAN_POINT ( 'NONE',  ( 11.71028986373773861, 87.46520591134841993, 130.0297596498208463 ) ) ;
#5105=ORIENTED_EDGE ( 'NONE', *, *, #8074, .T. ) ;
#5113=DIRECTION ( 'NONE',  ( 0.000000000000000000, -1.000000000000000000, 0.000000000000000000 ) ) ;
#5121=AXIS2_PLACEMENT_3D ( 'NONE', #8792, #57356, #48736 ) ;
#5126=CYLINDRICAL_SURFACE ( 'NONE', #69075, 9.425000000000000711 ) ;
#5154=EDGE_LOOP ( 'NONE', ( #63827, #17226, #55272, #36192 ) ) ;
#5171=CARTESIAN_POINT ( 'NONE',  ( -127.0239848601435995, 53.97500000000000142, 30.16249999999999787 ) ) ;
#5176=ADVANCED_FACE ( 'NONE', ( #41690 ), #53967, .F. ) ;
#5181=ORIENTED_EDGE ( 'NONE', *, *, #52435, .F. ) ;
#5185=CARTESIAN_POINT ( 'NONE',  ( -21.51128027773100015, 61.17290208904554305, 31.44902489669063073 ) ) ;
#5186=EDGE_CURVE ( 'NONE', #48446, #25704, #67627, .T. ) ;
#5209=CIRCLE ( 'NONE', #44293, 9.425000000000000711 ) ;
#5216=EDGE_CURVE ( 'NONE', #38814, #71713, #42213, .T. ) ;
#5232=VERTEX_POINT ( 'NONE', #48058 ) ;
#5236=VECTOR ( 'NONE', #48189, 1000.000000000000000 ) ;
#5268=ORIENTED_EDGE ( 'NONE', *, *, #31343, .F. ) ;
#5295=CARTESIAN_POINT ( 'NONE',  ( -10.54933103719152143, 75.47881567405516989, 130.1290928247797751 ) ) ;
#5300=DIRECTION ( 'NONE',  ( 0.000000000000000000, -1.000000000000000000, 0.000000000000000000 ) ) ;
#5303=CARTESIAN_POINT ( 'NONE',  ( -160.2664750769294812, 101.5999999999999943, -148.0533267522755807 ) ) ;
#5352=LINE ( 'NONE', #62548, #62068 ) ;
#5360=EDGE_LOOP ( 'NONE', ( #8884, #6285 ) ) ;
#5363=VERTEX_POINT ( 'NONE', #11673 ) ;
#5381=EDGE_CURVE ( 'NONE', #67371, #54555, #46157, .T. ) ;
#5395=DIRECTION ( 'NONE',  ( 0.000000000000000000, 1.000000000000000000, 0.000000000000000000 ) ) ;
#5414=LINE ( 'NONE', #89428, #45186 ) ;
#5450=LINE ( 'NONE', #4997, #48643 ) ;
#5454=FACE_OUTER_BOUND ( 'NONE', #53926, .T. ) ;
#5474=VERTEX_POINT ( 'NONE', #59793 ) ;
#5482=DIRECTION ( 'NONE',  ( 0.7071067811865344721, 0.000000000000000000, 0.7071067811865604513 ) ) ;
#5487=CARTESIAN_POINT ( 'NONE',  ( 10.40652293068787237, 75.26502159733162500, 130.1406823708988156 ) ) ;
#5514=ADVANCED_FACE ( 'NONE', ( #53410 ), #18923, .F. ) ;
#5534=DIRECTION ( 'NONE',  ( 1.000000000000000000, 0.000000000000000000, 2.108231265501709878E-16 ) ) ;
#5558=EDGE_CURVE ( 'NONE', #41931, #57180, #39366, .T. ) ;
#5573=CIRCLE ( 'NONE', #27343, 20.63750000000000284 ) ;
#5585=LINE ( 'NONE', #17859, #13035 ) ;
#5604=CIRCLE ( 'NONE', #2765, 31.75000000000000000 ) ;
#5642=DIRECTION ( 'NONE',  ( 1.000000000000000000, 0.000000000000000000, 0.000000000000000000 ) ) ;
#5648=DIRECTION ( 'NONE',  ( -1.000000000000000000, 0.000000000000000000, 4.277118011829300531E-15 ) ) ;
#5668=AXIS2_PLACEMENT_3D ( 'NONE', #25024, #11395, #24581 ) ;
#5702=DIRECTION ( 'NONE',  ( 0.000000000000000000, 0.000000000000000000, 1.000000000000000000 ) ) ;
#5715=CARTESIAN_POINT ( 'NONE',  ( 141.3509999999999991, 0.000000000000000000, 141.3509999999999991 ) ) ;
#5720=CARTESIAN_POINT ( 'NONE',  ( -109.4815320936060061, 57.56471201436704632, 71.12429803595952649 ) ) ;
#5721=AXIS2_PLACEMENT_3D ( 'NONE', #64400, #57570, #63953 ) ;
#5738=DIRECTION ( 'NONE',  ( 0.000000000000000000, 0.8660254037844387076, 0.4999999999999998890 ) ) ;
#5749=CARTESIAN_POINT ( 'NONE',  ( -10.52353995119061381, 75.44045292000316749, 130.1311838323437371 ) ) ;
#5810=DIRECTION ( 'NONE',  ( 0.000000000000000000, -1.000000000000000000, 0.000000000000000000 ) ) ;
#5834=VERTEX_POINT ( 'NONE', #50200 ) ;
#5837=ORIENTED_EDGE ( 'NONE', *, *, #86155, .T. ) ;
#5839=LINE ( 'NONE', #88950, #86209 ) ;
#5847=FACE_OUTER_BOUND ( 'NONE', #7286, .T. ) ;
#5960=VERTEX_POINT ( 'NONE', #45594 ) ;
#5984=DIRECTION ( 'NONE',  ( -0.7071067811865345831, 0.000000000000000000, -0.7071067811865604513 ) ) ;
#6014=CARTESIAN_POINT ( 'NONE',  ( 12.06576689403630454, 86.60966479152391173, 129.9976963971240025 ) ) ;
#6019=DIRECTION ( 'NONE',  ( 0.000000000000000000, 0.000000000000000000, 1.000000000000000000 ) ) ;
#6030=EDGE_CURVE ( 'NONE', #26732, #33670, #35078, .T. ) ;
#6039=DIRECTION ( 'NONE',  ( 0.000000000000000000, -1.000000000000000000, 0.000000000000000000 ) ) ;
#6043=FACE_OUTER_BOUND ( 'NONE', #3274, .T. ) ;
#6045=ORIENTED_EDGE ( 'NONE', *, *, #75444, .T. ) ;
#6085=EDGE_CURVE ( 'NONE', #30833, #66460, #68313, .T. ) ;
#6088=ORIENTED_EDGE ( 'NONE', *, *, #85066, .T. ) ;
#6119=CIRCLE ( 'NONE', #26402, 25.39999999999999858 ) ;
#6147=VERTEX_POINT ( 'NONE', #67399 ) ;
#6153=DIRECTION ( 'NONE',  ( 0.000000000000000000, -1.000000000000000000, 0.000000000000000000 ) ) ;
#6165=AXIS2_PLACEMENT_3D ( 'NONE', #29279, #27475, #76071 ) ;
#6169=CARTESIAN_POINT ( 'NONE',  ( -112.4269219824620478, 67.52370228190351042, 66.37105824381433195 ) ) ;
#6196=CARTESIAN_POINT ( 'NONE',  ( -7.057195792612153795, 71.99130726259811297, 130.3651223555374941 ) ) ;
#6197=CARTESIAN_POINT ( 'NONE',  ( -50.03799999999999670, 0.000000000000000000, 206.3750000000000000 ) ) ;
#6246=ADVANCED_FACE ( 'NONE', ( #69655 ), #43271, .F. ) ;
#6253=DIRECTION ( 'NONE',  ( 0.000000000000000000, 0.000000000000000000, 1.000000000000000000 ) ) ;
#6277=CARTESIAN_POINT ( 'NONE',  ( -123.4696824136392053, 20.32000000000000028, -179.8898777604655095 ) ) ;
#6285=ORIENTED_EDGE ( 'NONE', *, *, #3191, .F. ) ;
#6315=ORIENTED_EDGE ( 'NONE', *, *, #17305, .T. ) ;
#6334=LINE ( 'NONE', #83106, #44742 ) ;
#6339=CYLINDRICAL_SURFACE ( 'NONE', #73404, 12.69999999999999929 ) ;
#6343=VERTEX_POINT ( 'NONE', #86428 ) ;
#6370=VERTEX_POINT ( 'NONE', #71462 ) ;
#6374=CARTESIAN_POINT ( 'NONE',  ( 122.5505378705195909, 44.80423684447521993, -45.01691195935249112 ) ) ;
#6397=LINE ( 'NONE', #48160, #38253 ) ;
#6417=AXIS2_PLACEMENT_3D ( 'NONE', #81310, #67196, #73567 ) ;
#6423=CARTESIAN_POINT ( 'NONE',  ( 1.166476076187854022E-15, 114.2999999999999972, 9.525000000000000355 ) ) ;
#6428=CARTESIAN_POINT ( 'NONE',  ( 0.000000000000000000, 20.32000000000000028, 0.000000000000000000 ) ) ;
#6440=AXIS2_PLACEMENT_3D ( 'NONE', #77470, #710, #7979 ) ;
#6445=ORIENTED_EDGE ( 'NONE', *, *, #85042, .F. ) ;
#6465=CARTESIAN_POINT ( 'NONE',  ( 135.2444258376730204, 0.000000000000000000, -147.4575741623271767 ) ) ;
#6500=EDGE_LOOP ( 'NONE', ( #74205, #67199, #86606, #69951, #18273, #76747 ) ) ;
#6501=LINE ( 'NONE', #34200, #17892 ) ;
#6531=EDGE_CURVE ( 'NONE', #26221, #51337, #54095, .T. ) ;
#6554=CARTESIAN_POINT ( 'NONE',  ( 22.25283182517284075, 48.39572325881615456, 30.92657878646921432 ) ) ;
#6569=CARTESIAN_POINT ( 'NONE',  ( 31.75000000000000000, 24.56180297284579694, -3.174999999999999822 ) ) ;
#6605=CARTESIAN_POINT ( 'NONE',  ( -121.9014056762777329, 74.22174993621874250, 46.74836492626587159 ) ) ;
#6611=ORIENTED_EDGE ( 'NONE', *, *, #47315, .T. ) ;
#6630=AXIS2_PLACEMENT_3D ( 'NONE', #82779, #20540, #67779 ) ;
#6632=CARTESIAN_POINT ( 'NONE',  ( -12.69999999999999751, 81.76470274209911793, 129.9368274816649773 ) ) ;
#6657=DIRECTION ( 'NONE',  ( 3.491483361109380094E-15, 0.000000000000000000, 1.000000000000000000 ) ) ;
#6717=LINE ( 'NONE', #20361, #64420 ) ;
#6726=CYLINDRICAL_SURFACE ( 'NONE', #60956, 218.1859999999999786 ) ;
#6727=ORIENTED_EDGE ( 'NONE', *, *, #19121, .T. ) ;
#6737=DIRECTION ( 'NONE',  ( 2.505701470911820065E-15, 0.000000000000000000, 1.000000000000000000 ) ) ;
#6746=ORIENTED_EDGE ( 'NONE', *, *, #89384, .T. ) ;
#6787=ORIENTED_EDGE ( 'NONE', *, *, #71437, .T. ) ;
#6811=LINE ( 'NONE', #6, #53048 ) ;
#6814=CARTESIAN_POINT ( 'NONE',  ( 1.594823438788931513, 69.92315182778645521, 130.5484606227018958 ) ) ;
#6824=EDGE_CURVE ( 'NONE', #83969, #22713, #52381, .T. ) ;
#6845=VERTEX_POINT ( 'NONE', #3204 ) ;
#6943=VECTOR ( 'NONE', #50867, 1000.000000000000000 ) ;
#6945=VERTEX_POINT ( 'NONE', #26647 ) ;
#6965=AXIS2_PLACEMENT_3D ( 'NONE', #25339, #11726, #73948 ) ;
#6993=VECTOR ( 'NONE', #76413, 1000.000000000000000 ) ;
#7010=CARTESIAN_POINT ( 'NONE',  ( 148.0533267522749838, 20.32000000000000028, -160.2664750769289697 ) ) ;
#7033=ORIENTED_EDGE ( 'NONE', *, *, #68027, .T. ) ;
#7061=CARTESIAN_POINT ( 'NONE',  ( -114.5280640324896808, 70.85472008698103252, 62.67561285116475744 ) ) ;
#7087=CARTESIAN_POINT ( 'NONE',  ( -9.371942588247355488, 73.96144982415154345, 130.2197749970455050 ) ) ;
#7094=CARTESIAN_POINT ( 'NONE',  ( 0.000000000000000000, 12.27000000000000313, 0.000000000000000000 ) ) ;
#7095=VERTEX_POINT ( 'NONE', #14384 ) ;
#7104=VERTEX_POINT ( 'NONE', #56122 ) ;
#7110=VECTOR ( 'NONE', #49412, 1000.000000000000000 ) ;
#7143=CARTESIAN_POINT ( 'NONE',  ( -12.04016146640379148, 86.59615096602188089, 129.9997639365609245 ) ) ;
#7169=AXIS2_PLACEMENT_3D ( 'NONE', #46950, #81965, #75588 ) ;
#7187=DIRECTION ( 'NONE',  ( 0.000000000000000000, 0.000000000000000000, 1.000000000000000000 ) ) ;
#7192=PLANE ( 'NONE',  #14544 ) ;
#7221=EDGE_CURVE ( 'NONE', #43788, #6945, #30241, .T. ) ;
#7226=DIRECTION ( 'NONE',  ( 0.000000000000000000, 1.000000000000000000, 0.000000000000000000 ) ) ;
#7237=ORIENTED_EDGE ( 'NONE', *, *, #47452, .T. ) ;
#7263=CARTESIAN_POINT ( 'NONE',  ( -123.4696824136392053, 101.5999999999999943, -179.8898777604655095 ) ) ;
#7283=CARTESIAN_POINT ( 'NONE',  ( 119.5843592605237262, 52.19558960403061576, -52.38750000000002416 ) ) ;
#7286=EDGE_LOOP ( 'NONE', ( #82988, #76591, #25242, #57925 ) ) ;
#7306=ADVANCED_FACE ( 'NONE', ( #66074 ), #51548, .F. ) ;
#7348=FACE_OUTER_BOUND ( 'NONE', #61786, .T. ) ;
#7362=AXIS2_PLACEMENT_3D ( 'NONE', #20241, #35647, #69286 ) ;
#7387=LINE ( 'NONE', #27376, #23358 ) ;
#7407=CARTESIAN_POINT ( 'NONE',  ( -148.0533267522752112, 101.5999999999999943, 160.2664750769289697 ) ) ;
#7409=ORIENTED_EDGE ( 'NONE', *, *, #86155, .F. ) ;
#7420=CARTESIAN_POINT ( 'NONE',  ( 10.58784659601187350, 75.53659449424580430, 130.1259651751956312 ) ) ;
#7424=CARTESIAN_POINT ( 'NONE',  ( 170.2205283966864897, 20.32000000000000028, 79.24800000000000466 ) ) ;
#7446=CARTESIAN_POINT ( 'NONE',  ( -3.175000000000109956, 17.78000000000000114, -31.75000000000000000 ) ) ;
#7461=CARTESIAN_POINT ( 'NONE',  ( 196.2150000000000034, 43.68799999999999528, 57.14999999999999858 ) ) ;
#7465=ORIENTED_EDGE ( 'NONE', *, *, #78125, .F. ) ;
#7484=ORIENTED_EDGE ( 'NONE', *, *, #10397, .T. ) ;
#7501=DIRECTION ( 'NONE',  ( 0.000000000000000000, 1.000000000000000000, 0.000000000000000000 ) ) ;
#7507=CARTESIAN_POINT ( 'NONE',  ( -115.9581729443846143, 72.46394936478256454, 59.99146676500703990 ) ) ;
#7523=ORIENTED_EDGE ( 'NONE', *, *, #85177, .F. ) ;
#7526=LINE ( 'NONE', #34778, #3992 ) ;
#7543=CIRCLE ( 'NONE', #68429, 7.937500000000000000 ) ;
#7552=VERTEX_POINT ( 'NONE', #55111 ) ;
#7553=ADVANCED_FACE ( 'NONE', ( #88342 ), #75601, .T. ) ;
#7688=VERTEX_POINT ( 'NONE', #45070 ) ;
#7701=ORIENTED_EDGE ( 'NONE', *, *, #61457, .F. ) ;
#7711=CARTESIAN_POINT ( 'NONE',  ( -158.9822249764575020, 101.5999999999999943, 139.6999999999999886 ) ) ;
#7733=CARTESIAN_POINT ( 'NONE',  ( 33.98325472291465132, 24.56180297284579694, -3.174999999999999822 ) ) ;
#7737=ORIENTED_EDGE ( 'NONE', *, *, #34405, .F. ) ;
#7751=CARTESIAN_POINT ( 'NONE',  ( 126.0950369046984747, 65.73012104574902992, 33.83669062937374861 ) ) ;
#7756=AXIS2_PLACEMENT_3D ( 'NONE', #36514, #22891, #50567 ) ;
#7770=FILL_AREA_STYLE ('',( #49530 ) ) ;
#7779=CARTESIAN_POINT ( 'NONE',  ( -127.5252020268932114, 101.5999999999999943, 177.0380000000000109 ) ) ;
#7799=ORIENTED_EDGE ( 'NONE', *, *, #61457, .T. ) ;
#7811=CARTESIAN_POINT ( 'NONE',  ( 0.000000000000000000, 2.269999999999994245, -9.425000000000000711 ) ) ;
#7842=ORIENTED_EDGE ( 'NONE', *, *, #59061, .F. ) ;
#7873=CARTESIAN_POINT ( 'NONE',  ( 0.000000000000000000, 0.000000000000000000, 0.000000000000000000 ) ) ;
#7937=VERTEX_POINT ( 'NONE', #25533 ) ;
#7950=CARTESIAN_POINT ( 'NONE',  ( -112.9545031557597099, 68.49197848692702451, 65.46872494430569134 ) ) ;
#7971=CARTESIAN_POINT ( 'NONE',  ( 19.89663890320305839, 44.45000000000000284, 32.49205688096009936 ) ) ;
#7977=VECTOR ( 'NONE', #8445, 1000.000000000000000 ) ;
#7978=FACE_OUTER_BOUND ( 'NONE', #85148, .T. ) ;
#7979=DIRECTION ( 'NONE',  ( 0.000000000000000000, 0.000000000000000000, 1.000000000000000000 ) ) ;
#8014=ORIENTED_EDGE ( 'NONE', *, *, #64355, .T. ) ;
#8022=EDGE_LOOP ( 'NONE', ( #54716, #83488, #2307, #18096 ) ) ;
#8033=CARTESIAN_POINT ( 'NONE',  ( -11.02761275263880592, 88.85312730307458651, 130.0895250074965475 ) ) ;
#8043=ADVANCED_FACE ( 'NONE', ( #27774 ), #43180, .F. ) ;
#8067=ORIENTED_EDGE ( 'NONE', *, *, #57062, .T. ) ;
#8074=EDGE_CURVE ( 'NONE', #77506, #66460, #1428, .T. ) ;
#8077=AXIS2_PLACEMENT_3D ( 'NONE', #86892, #38283, #51019 ) ;
#8111=CARTESIAN_POINT ( 'NONE',  ( 196.2150000000000034, 37.33800000000000097, 50.79999999999999716 ) ) ;
#8116=ORIENTED_EDGE ( 'NONE', *, *, #43016, .F. ) ;
#8132=VECTOR ( 'NONE', #24237, 1000.000000000000000 ) ;
#8176=CARTESIAN_POINT ( 'NONE',  ( 119.9517054789250210, 49.13249813668914356, -51.54132924209260835 ) ) ;
#8199=VECTOR ( 'NONE', #4239, 1000.000000000000114 ) ;
#8212=DIRECTION ( 'NONE',  ( 0.000000000000000000, -1.000000000000000000, 0.000000000000000000 ) ) ;
#8256=PLANE ( 'NONE',  #64668 ) ;
#8289=LINE ( 'NONE', #22367, #55813 ) ;
#8321=VECTOR ( 'NONE', #21803, 1000.000000000000000 ) ;
#8337=CARTESIAN_POINT ( 'NONE',  ( 57.91199999999999903, 0.000000000000000000, 191.3008000794699797 ) ) ;
#8347=B_SPLINE_CURVE_WITH_KNOTS ( 'NONE', 3,
 ( #80272, #18015, #80712, #45698, #18461, #73880, #32528, #60234, #81620, #88868, #13010, #41137, #20713, #61579, #62486, #55198, #13896, #40697, #265, #68419, #27519, #67963, #67504, #76116, #89316, #41579, #6196, #27080, #82513, #54749, #21166, #75234, #69313, #7087, #47941, #75682, #33883, #62035, #20275, #13450, #48382, #5749, #82956, #5295, #83390, #76576, #47044, #55641, #68860, #88421, #89769, #12557, #47497, #19817, #27963, #32986, #34781, #60684, #26183, #26624, #48836, #6632, #53851 ),
 .UNSPECIFIED., .F., .F.,
 ( 4, 2, 2, 2, 1, 1, 1, 2, 2, 2, 2, 1, 1, 1, 1, 1, 2, 2, 2, 2, 2, 2, 2, 2, 1, 1, 1, 1, 2, 2, 2, 2, 1, 1, 1, 2, 2, 2, 4 ),
 ( 0.000000000000000000, 0.1249999999995831390, 0.1874999999993746669, 0.2187499999992704169, 0.2343749999992183475, 0.2421874999991923960, 0.2460937499991793231, 0.2480468749991724398, 0.2499999999991655286, 0.3124999999989367949, 0.3437499999988225530, 0.3593749999987653765, 0.3671874999987362886, 0.3710937499987211896, 0.3730468749987142507, 0.3740234374987106980, 0.3745117187487095323, 0.3749999999987083665, 0.4374999999987584376, 0.4687499999987840282, 0.4999999999988096189, 0.5624999999988609112, 0.5937499999988865573, 0.6093749999988995469, 0.6171874999989048760, 0.6210937499989086508, 0.6230468749989095389, 0.6240234374989099830, 0.6245117187489113153, 0.6249999999989126476, 0.6874999999990776267, 0.7187499999991611155, 0.7343749999992028599, 0.7421874999992246202, 0.7460937499992355004, 0.7480468749992409405, 0.7499999999992463806, 0.8749999999996231903, 1.000000000000000000 ),
 .UNSPECIFIED. ) ;
#8356=CARTESIAN_POINT ( 'NONE',  ( 123.4696824136382105, 101.5999999999999943, -179.8898777604649979 ) ) ;
#8398=ADVANCED_FACE ( 'NONE', ( #4547 ), #32235, .F. ) ;
#8416=DIRECTION ( 'NONE',  ( 8.503806984168930281E-16, 0.000000000000000000, -1.000000000000000000 ) ) ;
#8433=ORIENTED_EDGE ( 'NONE', *, *, #991, .F. ) ;
#8437=DIRECTION ( 'NONE',  ( 0.000000000000000000, -1.000000000000000000, 0.000000000000000000 ) ) ;
#8445=DIRECTION ( 'NONE',  ( 0.000000000000000000, -1.000000000000000000, 0.000000000000000000 ) ) ;
#8450=CARTESIAN_POINT ( 'NONE',  ( -3.175000000000109956, 24.56180297284579694, -31.75000000000000000 ) ) ;
#8462=DIRECTION ( 'NONE',  ( -1.000000000000000000, 3.651563665954189830E-16, 0.000000000000000000 ) ) ;
#8472=CYLINDRICAL_SURFACE ( 'NONE', #537, 38.10000000000000142 ) ;
#8475=EDGE_CURVE ( 'NONE', #36180, #15997, #60250, .T. ) ;
#8490=VECTOR ( 'NONE', #28169, 1000.000000000000000 ) ;
#8516=ORIENTED_EDGE ( 'NONE', *, *, #26265, .T. ) ;
#8531=CARTESIAN_POINT ( 'NONE',  ( -75.61066417432020614, 101.5999999999999943, 177.0380000000000109 ) ) ;
#8606=CARTESIAN_POINT ( 'NONE',  ( 196.2150000000000034, 37.33800000000000097, 50.79999999999999716 ) ) ;
#8612=ADVANCED_FACE ( 'NONE', ( #23999 ), #51225, .T. ) ;
#8619=ADVANCED_FACE ( 'NONE', ( #57148 ), #9464, .F. ) ;
#8627=AXIS2_PLACEMENT_3D ( 'NONE', #47101, #32586, #26674 ) ;
#8647=VECTOR ( 'NONE', #20300, 1000.000000000000000 ) ;
#8660=CARTESIAN_POINT ( 'NONE',  ( 124.1141232347067529, 71.87613260885804323, 40.50830340569535792 ) ) ;
#8662=ORIENTED_EDGE ( 'NONE', *, *, #2286, .T. ) ;
#8690=EDGE_CURVE ( 'NONE', #71713, #16666, #65326, .T. ) ;
#8709=CARTESIAN_POINT ( 'NONE',  ( 1.598849875094819542E-14, 44.45000000000000284, -130.5560000000000116 ) ) ;
#8719=DIRECTION ( 'NONE',  ( 1.000000000000000000, 0.000000000000000000, 0.000000000000000000 ) ) ;
#8748=DIRECTION ( 'NONE',  ( 0.000000000000000000, 0.000000000000000000, -1.000000000000000000 ) ) ;
#8760=ORIENTED_EDGE ( 'NONE', *, *, #24177, .F. ) ;
#8792=CARTESIAN_POINT ( 'NONE',  ( 0.000000000000000000, 20.32000000000000028, 0.000000000000000000 ) ) ;
#8813=ORIENTED_EDGE ( 'NONE', *, *, #25368, .T. ) ;
#8854=ORIENTED_EDGE ( 'NONE', *, *, #78387, .F. ) ;
#8884=ORIENTED_EDGE ( 'NONE', *, *, #74509, .F. ) ;
#8905=ADVANCED_FACE ( 'NONE', ( #17463 ), #2056, .F. ) ;
#8906=CARTESIAN_POINT ( 'NONE',  ( 0.000000000000000000, 2.269999999999994245, -9.525000000000000355 ) ) ;
#8919=CARTESIAN_POINT ( 'NONE',  ( 31.75000000000000000, 17.78000000000000114, 3.174999999999999822 ) ) ;
#8947=CARTESIAN_POINT ( 'NONE',  ( -11.93153746469517884, 86.90202483595902549, 130.0097012715444862 ) ) ;
#8962=EDGE_LOOP ( 'NONE', ( #82259, #47216, #39376, #70405 ) ) ;
#8973=VERTEX_POINT ( 'NONE', #51077 ) ;
#8980=CARTESIAN_POINT ( 'NONE',  ( 173.9900000000000091, 37.33800000000000097, 69.13087104677069306 ) ) ;
#9007=EDGE_CURVE ( 'NONE', #29697, #34694, #9759, .T. ) ;
#9009=DIRECTION ( 'NONE',  ( 0.000000000000000000, 1.000000000000000000, 0.000000000000000000 ) ) ;
#9034=DIRECTION ( 'NONE',  ( 0.000000000000000000, -1.000000000000000000, 0.000000000000000000 ) ) ;
#9049=CARTESIAN_POINT ( 'NONE',  ( 0.000000000000000000, 12.27000000000000313, 0.000000000000000000 ) ) ;
#9065=DIRECTION ( 'NONE',  ( -3.491483361109380094E-15, 0.000000000000000000, -1.000000000000000000 ) ) ;
#9067=CARTESIAN_POINT ( 'NONE',  ( -20.41604128349800007, 45.08960384674290367, 32.16949814425970544 ) ) ;
#9082=CARTESIAN_POINT ( 'NONE',  ( -55.48342271751670296, 101.5999999999999943, 171.1197181046785261 ) ) ;
#9095=ORIENTED_EDGE ( 'NONE', *, *, #23860, .T. ) ;
#9100=DIRECTION ( 'NONE',  ( -3.491483361109380094E-15, 0.000000000000000000, -1.000000000000000000 ) ) ;
#9120=DIRECTION ( 'NONE',  ( 0.000000000000000000, 0.000000000000000000, 1.000000000000000000 ) ) ;
#9126=FACE_OUTER_BOUND ( 'NONE', #79650, .T. ) ;
#9139=B_SPLINE_CURVE_WITH_KNOTS ( 'NONE', 3,
 ( #78753, #16506, #44185, #65971, #86007, #86448, #3763, #51881, #58707, #79195, #36510, #29683, #9246, #79636, #10134, #44633, #72804, #85120, #50563, #78305, #37842, #3323, #16067, #43748, #20085, #4656, #81432, #4209, #12828, #33705, #66873, #25537, #74146, #40512, #53212, #25094, #11921, #26884, #81871, #73697, #39609, #19622, #47758, #11012, #74587, #61396, #47309, #67314, #39171, #38717, #75041, #60494, #68233, #5104, #32799, #32341, #6014, #60043, #89125, #26442, #66420 ),
 .UNSPECIFIED., .F., .F.,
 ( 4, 2, 2, 2, 1, 1, 1, 2, 2, 2, 2, 1, 1, 1, 1, 1, 2, 2, 2, 2, 2, 2, 2, 1, 1, 1, 1, 2, 2, 2, 2, 1, 1, 1, 2, 2, 2, 4 ),
 ( 0.000000000000000000, 0.1249999999998101241, 0.1874999999997149780, 0.2187499999996670441, 0.2343749999996433686, 0.2421874999996319611, 0.2460937499996265487, 0.2480468749996235234, 0.2499999999996205258, 0.3124999999995198285, 0.3437499999994693689, 0.3593749999994442779, 0.3671874999994313438, 0.3710937499994253486, 0.3730468749994229061, 0.3740234374994215738, 0.3745117187494213518, 0.3749999999994211297, 0.4374999999993766098, 0.4999999999993320898, 0.5624999999992875699, 0.5937499999992651434, 0.6093749999992530419, 0.6171874999992470467, 0.6210937499992429389, 0.6230468749992407185, 0.6240234374992398303, 0.6245117187492407185, 0.6249999999992417177, 0.6874999999993813837, 0.7187499999994504396, 0.7343749999994850786, 0.7421874999995022870, 0.7460937499995110578, 0.7480468749995142774, 0.7499999999995174971, 0.8749999999997587485, 1.000000000000000000 ),
 .UNSPECIFIED. ) ;
#9188=FACE_OUTER_BOUND ( 'NONE', #53338, .T. ) ;
#9202=EDGE_LOOP ( 'NONE', ( #48581, #80882, #34303, #83240 ) ) ;
#9232=CARTESIAN_POINT ( 'NONE',  ( -179.8898777604649979, 0.000000000000000000, 122.9960808104842016 ) ) ;
#9236=EDGE_CURVE ( 'NONE', #32634, #45956, #85000, .T. ) ;
#9246=CARTESIAN_POINT ( 'NONE',  ( 4.836742537503020856, 94.29291739919693782, 130.4663756832428305 ) ) ;
#9346=CYLINDRICAL_SURFACE ( 'NONE', #54456, 1.523999999999053889 ) ;
#9354=ORIENTED_EDGE ( 'NONE', *, *, #3393, .F. ) ;
#9374=CIRCLE ( 'NONE', #6440, 6.349999999999994316 ) ;
#9394=EDGE_LOOP ( 'NONE', ( #14304, #65698 ) ) ;
#9464=PLANE ( 'NONE',  #57333 ) ;
#9502=AXIS2_PLACEMENT_3D ( 'NONE', #80863, #18616, #74030 ) ;
#9521=DIRECTION ( 'NONE',  ( 1.067350013832299363E-17, -0.9961946980917455452, 0.08715574274765836016 ) ) ;
#9542=CARTESIAN_POINT ( 'NONE',  ( 131.3179999999999836, 53.97500000000000142, 50.79999999999999716 ) ) ;
#9545=PLANE ( 'NONE',  #75107 ) ;
#9547=CARTESIAN_POINT ( 'NONE',  ( 122.8489780378840948, 73.53925275838706455, 44.19769267541737179 ) ) ;
#9552=CARTESIAN_POINT ( 'NONE',  ( -141.3509999999999991, 101.5999999999999943, 132.7150000000000034 ) ) ;
#9558=DIRECTION ( 'NONE',  ( 0.000000000000000000, 0.000000000000000000, 1.000000000000000000 ) ) ;
#9572=ORIENTED_EDGE ( 'NONE', *, *, #56651, .F. ) ;
#9613=DIRECTION ( 'NONE',  ( 0.000000000000000000, -1.000000000000000000, 0.000000000000000000 ) ) ;
#9622=EDGE_CURVE ( 'NONE', #84402, #10839, #85018, .T. ) ;
#9647=ORIENTED_EDGE ( 'NONE', *, *, #8475, .T. ) ;
#9651=AXIS2_PLACEMENT_3D ( 'NONE', #10395, #72631, #51707 ) ;
#9664=CYLINDRICAL_SURFACE ( 'NONE', #86922, 179.8898777604655095 ) ;
#9670=AXIS2_PLACEMENT_3D ( 'NONE', #79696, #24707, #73292 ) ;
#9679=ORIENTED_EDGE ( 'NONE', *, *, #64054, .F. ) ;
#9705=PLANE ( 'NONE',  #89314 ) ;
#9713=LINE ( 'NONE', #71508, #28976 ) ;
#9759=LINE ( 'NONE', #65161, #80438 ) ;
#9763=EDGE_LOOP ( 'NONE', ( #22885, #39877, #51909, #10660, #56595, #72729, #25972, #86063, #29563, #24401, #13494, #38447, #82801, #4822, #72600, #86296 ) ) ;
#9828=CARTESIAN_POINT ( 'NONE',  ( -7.057053722110693705, 93.10878806376580030, 130.3651300669557997 ) ) ;
#9857=ORIENTED_EDGE ( 'NONE', *, *, #64872, .T. ) ;
#9879=CARTESIAN_POINT ( 'NONE',  ( 6.836113969089879561, 69.74575608423708672, 37.48795912257015317 ) ) ;
#9888=CARTESIAN_POINT ( 'NONE',  ( 173.9900000000000091, 20.32000000000000028, -71.37400000000000944 ) ) ;
#9889=VECTOR ( 'NONE', #5482, 1000.000000000000114 ) ;
#9901=FACE_BOUND ( 'NONE', #72544, .T. ) ;
#9906=EDGE_CURVE ( 'NONE', #34082, #88226, #40411, .T. ) ;
#9917=ADVANCED_FACE ( 'NONE', ( #5454 ), #14411, .F. ) ;
#9923=ORIENTED_EDGE ( 'NONE', *, *, #82809, .T. ) ;
#9924=VECTOR ( 'NONE', #27448, 1000.000000000000000 ) ;
#9933=CARTESIAN_POINT ( 'NONE',  ( 3.175000000000334666, 17.78000000000000114, 31.75000000000000000 ) ) ;
#9943=CYLINDRICAL_SURFACE ( 'NONE', #33093, 9.525000000000000355 ) ;
#9951=ORIENTED_EDGE ( 'NONE', *, *, #21931, .F. ) ;
#9958=AXIS2_PLACEMENT_3D ( 'NONE', #22751, #57235, #22295 ) ;
#9993=CARTESIAN_POINT ( 'NONE',  ( 114.4819906290133247, 70.80449033172386919, 62.76244765184264907 ) ) ;
#10019=EDGE_CURVE ( 'NONE', #47532, #43122, #25894, .T. ) ;
#10030=ORIENTED_EDGE ( 'NONE', *, *, #36905, .T. ) ;
#10034=VECTOR ( 'NONE', #6737, 1000.000000000000000 ) ;
#10043=ORIENTED_EDGE ( 'NONE', *, *, #13403, .F. ) ;
#10078=( GEOMETRIC_REPRESENTATION_CONTEXT ( 3 ) GLOBAL_UNCERTAINTY_ASSIGNED_CONTEXT ( ( #71455 ) ) GLOBAL_UNIT_ASSIGNED_CONTEXT ( ( #87751, #12805, #53188 ) ) REPRESENTATION_CONTEXT ( 'NONE', 'WORKASPACE' ) );
#10134=CARTESIAN_POINT ( 'NONE',  ( 5.207367076801767247, 94.13935037115494708, 130.4525656815699790 ) ) ;
#10160=DIRECTION ( 'NONE',  ( 2.108231265501709878E-16, 0.000000000000000000, -1.000000000000000000 ) ) ;
#10173=DIRECTION ( 'NONE',  ( -0.7071067811865360264, 0.000000000000000000, 0.7071067811865588970 ) ) ;
#10183=DIRECTION ( 'NONE',  ( 1.514143847546114723E-15, -0.8660254037844387076, -0.4999999999999998890 ) ) ;
#10186=CARTESIAN_POINT ( 'NONE',  ( -127.0239848601435995, 53.97500000000000142, 30.16249999999999787 ) ) ;
#10267=CARTESIAN_POINT ( 'NONE',  ( -4.054936310288488777, 94.61721499974834160, 130.4955353351740257 ) ) ;
#10272=CARTESIAN_POINT ( 'NONE',  ( 126.6266614082200732, 45.94094662677520802, 31.78937376590539898 ) ) ;
#10280=CARTESIAN_POINT ( 'NONE',  ( -75.61066417432020614, 0.000000000000000000, 189.7379999999999995 ) ) ;
#10283=CIRCLE ( 'NONE', #61042, 161.5439999999999827 ) ;
#10303=LINE ( 'NONE', #24388, #14151 ) ;
#10311=ORIENTED_EDGE ( 'NONE', *, *, #9236, .F. ) ;
#10325=DIRECTION ( 'NONE',  ( -1.000000000000000000, 0.000000000000000000, 0.000000000000000000 ) ) ;
#10328=CARTESIAN_POINT ( 'NONE',  ( 55.11501535284990183, 20.32000000000000028, 183.9403141659174992 ) ) ;
#10330=AXIS2_PLACEMENT_3D ( 'NONE', #33971, #4938, #25831 ) ;
#10331=LINE ( 'NONE', #9888, #65740 ) ;
#10354=LINE ( 'NONE', #65320, #77448 ) ;
#10366=PLANE ( 'NONE',  #67370 ) ;
#10389=VERTEX_POINT ( 'NONE', #12956 ) ;
#10395=CARTESIAN_POINT ( 'NONE',  ( 183.5150000000000148, 37.33800000000000097, 50.79999999999999716 ) ) ;
#10397=EDGE_CURVE ( 'NONE', #66460, #80913, #70723, .T. ) ;
#10433=CARTESIAN_POINT ( 'NONE',  ( 109.6451729131657657, 58.77969955619902720, 70.87177885828612034 ) ) ;
#10435=ORIENTED_EDGE ( 'NONE', *, *, #61910, .F. ) ;
#10450=CARTESIAN_POINT ( 'NONE',  ( 131.3179999999999836, 34.75001145038169881, 58.30374716505330213 ) ) ;
#10454=CARTESIAN_POINT ( 'NONE',  ( 170.2205283966864897, 20.32000000000000028, 71.37400000000000944 ) ) ;
#10463=AXIS2_PLACEMENT_3D ( 'NONE', #54197, #40597, #32884 ) ;
#10546=ORIENTED_EDGE ( 'NONE', *, *, #10689, .T. ) ;
#10588=DIRECTION ( 'NONE',  ( 0.000000000000000000, 0.000000000000000000, -1.000000000000000000 ) ) ;
#10600=DIRECTION ( 'NONE',  ( 0.000000000000000000, 0.000000000000000000, -1.000000000000000000 ) ) ;
#10604=CARTESIAN_POINT ( 'NONE',  ( 0.000000000000000000, 101.5999999999999943, 0.000000000000000000 ) ) ;
#10610=ORIENTED_EDGE ( 'NONE', *, *, #27093, .T. ) ;
#10623=ORIENTED_EDGE ( 'NONE', *, *, #79318, .F. ) ;
#10624=ORIENTED_EDGE ( 'NONE', *, *, #30029, .F. ) ;
#10626=DIRECTION ( 'NONE',  ( 0.000000000000000000, 1.000000000000000000, 0.000000000000000000 ) ) ;
#10658=DIRECTION ( 'NONE',  ( 0.000000000000000000, -1.000000000000000000, 0.000000000000000000 ) ) ;
#10660=ORIENTED_EDGE ( 'NONE', *, *, #35021, .T. ) ;
#10689=EDGE_CURVE ( 'NONE', #28034, #25618, #28820, .T. ) ;
#10698=CARTESIAN_POINT ( 'NONE',  ( -4.878244184937265970, 94.27573757619954620, 130.4648306225670353 ) ) ;
#10724=CARTESIAN_POINT ( 'NONE',  ( -110.3511101689945093, 62.10781539098685045, 69.76748536262132916 ) ) ;
#10759=ORIENTED_EDGE ( 'NONE', *, *, #75212, .T. ) ;
#10832=CYLINDRICAL_SURFACE ( 'NONE', #2400, 7.937500000000000000 ) ;
#10836=EDGE_LOOP ( 'NONE', ( #78401, #77253, #65207, #69259, #65581, #48476, #23835, #25122, #31605, #28971, #23926, #82289, #62450, #36495, #14722, #29877, #4368, #34971 ) ) ;
#10839=VERTEX_POINT ( 'NONE', #25560 ) ;
#10847=DIRECTION ( 'NONE',  ( -1.000000000000000000, 0.000000000000000000, 0.000000000000000000 ) ) ;
#10850=ORIENTED_EDGE ( 'NONE', *, *, #51520, .T. ) ;
#10868=DIRECTION ( 'NONE',  ( -1.000000000000000000, 0.000000000000000000, -1.840813417405305102E-14 ) ) ;
#10873=CARTESIAN_POINT ( 'NONE',  ( 121.7044748306527424, 74.30620332398891037, 47.25378613605970202 ) ) ;
#10881=VERTEX_POINT ( 'NONE', #19205 ) ;
#10933=ORIENTED_EDGE ( 'NONE', *, *, #69248, .T. ) ;
#10967=EDGE_LOOP ( 'NONE', ( #87494, #40712, #87038, #72397 ) ) ;
#10986=FACE_BOUND ( 'NONE', #27944, .T. ) ;
#11003=CARTESIAN_POINT ( 'NONE',  ( 196.2150000000000034, 37.33800000000000097, 41.27499999999999858 ) ) ;
#11012=CARTESIAN_POINT ( 'NONE',  ( 10.54993534173505054, 89.62028068362222655, 130.1290436628989653 ) ) ;
#11013=VERTEX_POINT ( 'NONE', #77302 ) ;
#11043=DIRECTION ( 'NONE',  ( 0.000000000000000000, 0.000000000000000000, -1.000000000000000000 ) ) ;
#11095=CARTESIAN_POINT ( 'NONE',  ( 183.5150000000000148, 21.46300000000000097, 41.63456447661474868 ) ) ;
#11128=CARTESIAN_POINT ( 'NONE',  ( -215.9000000000000057, 101.5999999999999943, 146.9389999999999930 ) ) ;
#11161=ORIENTED_EDGE ( 'NONE', *, *, #81296, .F. ) ;
#11173=CARTESIAN_POINT ( 'NONE',  ( -111.0232030825078624, 64.26406744673955984, 68.69319255069000008 ) ) ;
#11178=VERTEX_POINT ( 'NONE', #3675 ) ;
#11263=DIRECTION ( 'NONE',  ( -0.7071067811865621167, 0.000000000000000000, 0.7071067811865330288 ) ) ;
#11271=CARTESIAN_POINT ( 'NONE',  ( 120.4547041627946840, 58.04868223456158915, -50.35440352988698010 ) ) ;
#11301=DIRECTION ( 'NONE',  ( 0.7071067811865835440, 0.000000000000000000, 0.7071067811865114905 ) ) ;
#11315=LINE ( 'NONE', #32650, #12742 ) ;
#11317=CARTESIAN_POINT ( 'NONE',  ( 114.8133063487188963, 71.21048122817593651, 62.15126537821431185 ) ) ;
#11332=EDGE_LOOP ( 'NONE', ( #81199, #10623, #23643, #83248 ) ) ;
#11355=CIRCLE ( 'NONE', #59190, 8.636000000000004562 ) ;
#11395=DIRECTION ( 'NONE',  ( 0.000000000000000000, -1.000000000000000000, 0.000000000000000000 ) ) ;
#11399=DIRECTION ( 'NONE',  ( 0.000000000000000000, 1.000000000000000000, 0.000000000000000000 ) ) ;
#11426=FACE_OUTER_BOUND ( 'NONE', #76945, .T. ) ;
#11435=CIRCLE ( 'NONE', #33223, 6.349999999999999645 ) ;
#11486=ORIENTED_EDGE ( 'NONE', *, *, #33703, .T. ) ;
#11489=CIRCLE ( 'NONE', #44925, 8.636000000000004562 ) ;
#11492=CARTESIAN_POINT ( 'NONE',  ( -186.2398777604655038, 0.000000000000000000, -12.69999999999999929 ) ) ;
#11531=DIRECTION ( 'NONE',  ( 0.000000000000000000, 0.000000000000000000, 1.000000000000000000 ) ) ;
#11539=AXIS2_PLACEMENT_3D ( 'NONE', #32473, #53345, #33380 ) ;
#11550=B_SPLINE_CURVE_WITH_KNOTS ( 'NONE', 3,
 ( #43432, #71178, #30715, #3013, #10272, #4800, #18414, #24354, #66115, #52463, #58411, #86139, #45651, #25230, #46102, #32045, #38412, #23915 ),
 .UNSPECIFIED., .F., .F.,
 ( 4, 2, 2, 2, 2, 2, 2, 2, 4 ),
 ( 0.000000000000000000, 0.1249999999999989175, 0.1874999999999970024, 0.2499999999999950595, 0.3749999999999940048, 0.4374999999999941158, 0.4999999999999942268, 0.7499999999999970024, 1.000000000000000000 ),
 .UNSPECIFIED. ) ;
#11552=ADVANCED_FACE ( 'NONE', ( #78102 ), #9943, .F. ) ;
#11565=DIRECTION ( 'NONE',  ( -4.277118011829300531E-15, 0.000000000000000000, -1.000000000000000000 ) ) ;
#11570=STYLED_ITEM ( 'NONE', ( #56798 ), #83525 ) ;
#11576=LINE ( 'NONE', #81968, #71284 ) ;
#11581=AXIS2_PLACEMENT_3D ( 'NONE', #12533, #71753, #79018 ) ;
#11603=VECTOR ( 'NONE', #86913, 1000.000000000000000 ) ;
#11606=DIRECTION ( 'NONE',  ( 0.000000000000000000, -1.000000000000000000, 0.000000000000000000 ) ) ;
#11616=VERTEX_POINT ( 'NONE', #51247 ) ;
#11657=EDGE_LOOP ( 'NONE', ( #15347, #20222 ) ) ;
#11659=LINE ( 'NONE', #39353, #43073 ) ;
#11660=CIRCLE ( 'NONE', #2914, 38.10000000000000142 ) ;
#11671=LINE ( 'NONE', #86188, #28805 ) ;
#11673=CARTESIAN_POINT ( 'NONE',  ( -3.174999999999664979, 17.78000000000000114, 31.75000000000000000 ) ) ;
#11675=EDGE_CURVE ( 'NONE', #66477, #63182, #33944, .T. ) ;
#11677=CARTESIAN_POINT ( 'NONE',  ( 173.9900000000000091, 52.73749999999999716, -44.45000000000000284 ) ) ;
#11703=ADVANCED_FACE ( 'NONE', ( #13073 ), #47113, .F. ) ;
#11712=DIRECTION ( 'NONE',  ( 0.000000000000000000, -1.000000000000000000, 0.000000000000000000 ) ) ;
#11724=ADVANCED_FACE ( 'NONE', ( #33503, #39420 ), #61642, .F. ) ;
#11726=DIRECTION ( 'NONE',  ( -0.7071067811865210384, 0.000000000000000000, 0.7071067811865739960 ) ) ;
#11730=CARTESIAN_POINT ( 'NONE',  ( 124.5534632449514589, 58.63620287803254882, -39.13237319201113706 ) ) ;
#11763=DIRECTION ( 'NONE',  ( 0.000000000000000000, 0.000000000000000000, 1.000000000000000000 ) ) ;
#11774=CARTESIAN_POINT ( 'NONE',  ( 113.5620303038072905, 69.49466463746259137, 64.41016170726432222 ) ) ;
#11789=CARTESIAN_POINT ( 'NONE',  ( 0.000000000000000000, 125.7300000000000040, 0.000000000000000000 ) ) ;
#11835=DIRECTION ( 'NONE',  ( 0.000000000000000000, 0.000000000000000000, 1.000000000000000000 ) ) ;
#11847=DIRECTION ( 'NONE',  ( -1.000000000000000000, 0.000000000000000000, 0.000000000000000000 ) ) ;
#11898=CARTESIAN_POINT ( 'NONE',  ( 0.000000000000000000, 17.78000000000000114, 0.000000000000000000 ) ) ;
#11921=CARTESIAN_POINT ( 'NONE',  ( 10.38443768554948932, 89.86159749365012317, 130.1424040926225132 ) ) ;
#11930=DIRECTION ( 'NONE',  ( 0.000000000000000000, 0.000000000000000000, 1.000000000000000000 ) ) ;
#11999=ADVANCED_FACE ( 'NONE', ( #15765 ), #81018, .F. ) ;
#12006=CARTESIAN_POINT ( 'NONE',  ( -23.05114358122109053, 56.73092669637083674, 30.33591271885418905 ) ) ;
#12028=CARTESIAN_POINT ( 'NONE',  ( 196.2150000000000034, 30.98800000000000310, 44.45000000000000284 ) ) ;
#12082=ORIENTED_EDGE ( 'NONE', *, *, #49250, .F. ) ;
#12088=CONICAL_SURFACE ( 'NONE', #41120, 25.39999999999999858, 0.7853981633974984611 ) ;
#12099=ORIENTED_EDGE ( 'NONE', *, *, #44068, .F. ) ;
#12110=CARTESIAN_POINT ( 'NONE',  ( -187.8075999999999794, 101.5999999999999943, -12.69999999999999929 ) ) ;
#12123=CARTESIAN_POINT ( 'NONE',  ( -179.6544565346565037, 20.32000000000000028, -9.200237383489920262 ) ) ;
#12149=VERTEX_POINT ( 'NONE', #47347 ) ;
#12156=CARTESIAN_POINT ( 'NONE',  ( 31.75000000000000000, 8.255000000000000782, -3.174999999999999822 ) ) ;
#12179=CARTESIAN_POINT ( 'NONE',  ( 123.6114559063626928, 60.30978874921765964, -42.01581149136940496 ) ) ;
#12215=CARTESIAN_POINT ( 'NONE',  ( -12.69999999999999929, 82.54999999999999716, -179.8908777604655143 ) ) ;
#12226=VERTEX_POINT ( 'NONE', #19217 ) ;
#12239=VERTEX_POINT ( 'NONE', #34170 ) ;
#12294=CARTESIAN_POINT ( 'NONE',  ( 160.2664750769289697, 0.000000000000000000, 148.0533267522752112 ) ) ;
#12336=DIRECTION ( 'NONE',  ( -0.7071067811865604513, 0.000000000000000000, 0.7071067811865345831 ) ) ;
#12358=CARTESIAN_POINT ( 'NONE',  ( 163.0822201311030142, 20.32000000000000028, -75.92468371870729982 ) ) ;
#12361=VECTOR ( 'NONE', #82323, 1000.000000000000000 ) ;
#12378=EDGE_LOOP ( 'NONE', ( #345, #76654, #83196, #65193 ) ) ;
#12388=DIRECTION ( 'NONE',  ( 0.000000000000000000, 1.000000000000000000, 0.000000000000000000 ) ) ;
#12438=VECTOR ( 'NONE', #70391, 1000.000000000000000 ) ;
#12439=VECTOR ( 'NONE', #24947, 1000.000000000000000 ) ;
#12476=EDGE_CURVE ( 'NONE', #7688, #45185, #26782, .T. ) ;
#12483=CARTESIAN_POINT ( 'NONE',  ( 21.53388387833662065, 46.83799769796173251, 31.43192935164580604 ) ) ;
#12504=EDGE_CURVE ( 'NONE', #85180, #13373, #47072, .T. ) ;
#12509=ORIENTED_EDGE ( 'NONE', *, *, #29743, .F. ) ;
#12514=ADVANCED_FACE ( 'NONE', ( #2810 ), #16882, .F. ) ;
#12528=CARTESIAN_POINT ( 'NONE',  ( -111.5512539134624888, 65.62907064895924236, 67.83205493406804010 ) ) ;
#12531=VECTOR ( 'NONE', #5534, 1000.000000000000000 ) ;
#12533=CARTESIAN_POINT ( 'NONE',  ( 173.9900000000000091, 52.73749999999999716, -44.45000000000000284 ) ) ;
#12551=CIRCLE ( 'NONE', #14043, 179.8898777604655095 ) ;
#12557=CARTESIAN_POINT ( 'NONE',  ( -11.54220284826591758, 77.25119473389790414, 130.0448154359650630 ) ) ;
#12569=EDGE_CURVE ( 'NONE', #47365, #46362, #3692, .T. ) ;
#12577=DIRECTION ( 'NONE',  ( 0.000000000000000000, 1.000000000000000000, 0.000000000000000000 ) ) ;
#12587=ADVANCED_FACE ( 'NONE', ( #33185 ), #27262, .F. ) ;
#12630=ORIENTED_EDGE ( 'NONE', *, *, #76388, .T. ) ;
#12656=CIRCLE ( 'NONE', #44534, 218.1859999999999786 ) ;
#12662=VECTOR ( 'NONE', #40626, 1000.000000000000000 ) ;
#12692=AXIS2_PLACEMENT_3D ( 'NONE', #46707, #74436, #39901 ) ;
#12694=CARTESIAN_POINT ( 'NONE',  ( 0.000000000000000000, 101.5999999999999943, 130.5560000000000116 ) ) ;
#12735=CARTESIAN_POINT ( 'NONE',  ( -12.69999999999999929, 82.54999999999999716, 206.3750000000000000 ) ) ;
#12740=EDGE_LOOP ( 'NONE', ( #37958, #5268, #57873, #66298 ) ) ;
#12742=VECTOR ( 'NONE', #88084, 1000.000000000000000 ) ;
#12761=DIRECTION ( 'NONE',  ( 0.000000000000000000, 1.000000000000000000, 0.000000000000000000 ) ) ;
#12781=CYLINDRICAL_SURFACE ( 'NONE', #17131, 8.636000000000004562 ) ;
#12805=( NAMED_UNIT ( * ) PLANE_ANGLE_UNIT ( ) SI_UNIT ( $, .RADIAN. ) );
#12827=AXIS2_PLACEMENT_3D ( 'NONE', #28627, #50403, #72209 ) ;
#12828=CARTESIAN_POINT ( 'NONE',  ( 7.568530249623516504, 92.75688873515042587, 130.3366983285493461 ) ) ;
#12840=EDGE_LOOP ( 'NONE', ( #86570, #72475, #26590, #31340 ) ) ;
#12846=CARTESIAN_POINT ( 'NONE',  ( -215.9010000000000105, 52.73749999999999716, -44.45000000000000284 ) ) ;
#12898=DIRECTION ( 'NONE',  ( 0.000000000000000000, 0.000000000000000000, -1.000000000000000000 ) ) ;
#12903=CARTESIAN_POINT ( 'NONE',  ( -23.27731929905159802, 54.32390312253606623, 30.16249999999998366 ) ) ;
#12930=CIRCLE ( 'NONE', #76785, 7.874000000000005883 ) ;
#12939=PLANE ( 'NONE',  #75829 ) ;
#12956=CARTESIAN_POINT ( 'NONE',  ( 173.9900000000000091, 53.21300000000000097, 41.63456447661469895 ) ) ;
#12972=ORIENTED_EDGE ( 'NONE', *, *, #9622, .F. ) ;
#12984=CARTESIAN_POINT ( 'NONE',  ( -122.8759924518541169, 73.50212837636460961, 44.11811403647472929 ) ) ;
#13010=CARTESIAN_POINT ( 'NONE',  ( -4.771202963297667132, 70.78025357177421029, 130.4687910435467018 ) ) ;
#13014=FACE_OUTER_BOUND ( 'NONE', #73364, .T. ) ;
#13035=VECTOR ( 'NONE', #6039, 1000.000000000000000 ) ;
#13073=FACE_OUTER_BOUND ( 'NONE', #35394, .T. ) ;
#13078=DIRECTION ( 'NONE',  ( 0.000000000000000000, 0.000000000000000000, 1.000000000000000000 ) ) ;
#13119=CARTESIAN_POINT ( 'NONE',  ( -179.8898777604655095, 0.000000000000000000, -12.69999999999999929 ) ) ;
#13120=PLANE ( 'NONE',  #48994 ) ;
#13144=ORIENTED_EDGE ( 'NONE', *, *, #78014, .F. ) ;
#13182=FACE_OUTER_BOUND ( 'NONE', #45910, .T. ) ;
#13195=CARTESIAN_POINT ( 'NONE',  ( 5.011961811782480680, 70.88063028345509053, 130.4597710397083858 ) ) ;
#13201=CARTESIAN_POINT ( 'NONE',  ( 121.2668985255015031, 45.81534544650252627, -48.36754857886660375 ) ) ;
#13204=VERTEX_POINT ( 'NONE', #25545 ) ;
#13236=ORIENTED_EDGE ( 'NONE', *, *, #6085, .F. ) ;
#13256=EDGE_CURVE ( 'NONE', #5960, #51180, #24661, .T. ) ;
#13265=CARTESIAN_POINT ( 'NONE',  ( 1.154229608196380665E-15, 12.27000000000000313, 9.425000000000000711 ) ) ;
#13301=CARTESIAN_POINT ( 'NONE',  ( -179.6544565346565037, 20.32000000000000028, -9.200237383489920262 ) ) ;
#13370=CARTESIAN_POINT ( 'NONE',  ( 147.4575741623270062, 0.000000000000000000, -135.2444258376734183 ) ) ;
#13373=VERTEX_POINT ( 'NONE', #55017 ) ;
#13377=CARTESIAN_POINT ( 'NONE',  ( 19.89663890320305839, 44.45000000000000284, 32.49205688096009936 ) ) ;
#13403=EDGE_CURVE ( 'NONE', #23728, #39686, #40965, .T. ) ;
#13409=AXIS2_PLACEMENT_3D ( 'NONE', #85776, #23985, #40721 ) ;
#13410=DIRECTION ( 'NONE',  ( 0.000000000000000000, 0.000000000000000000, 1.000000000000000000 ) ) ;
#13412=CIRCLE ( 'NONE', #59811, 9.525000000000000355 ) ;
#13422=FACE_OUTER_BOUND ( 'NONE', #84147, .T. ) ;
#13426=CARTESIAN_POINT ( 'NONE',  ( -114.2735689154193750, 70.52307754910606263, 63.13935773474766222 ) ) ;
#13440=CARTESIAN_POINT ( 'NONE',  ( 183.5150000000000148, 37.33800000000000097, 32.46912895322940074 ) ) ;
#13450=CARTESIAN_POINT ( 'NONE',  ( -10.45593524471656721, 75.34132956249517576, 130.1366506729525554 ) ) ;
#13451=EDGE_CURVE ( 'NONE', #59655, #72639, #78658, .T. ) ;
#13462=CARTESIAN_POINT ( 'NONE',  ( -3.174999999999664979, 8.255000000000000782, 31.75000000000000000 ) ) ;
#13471=CARTESIAN_POINT ( 'NONE',  ( 3.174999999999879918, 8.255000000000000782, -33.98325472291465132 ) ) ;
#13473=DIRECTION ( 'NONE',  ( 1.000000000000000000, 0.000000000000000000, 0.000000000000000000 ) ) ;
#13483=EDGE_LOOP ( 'NONE', ( #10610, #59710, #31499, #63498 ) ) ;
#13484=CARTESIAN_POINT ( 'NONE',  ( -127.0239848601436563, 53.14309343562469934, 30.16249999999989839 ) ) ;
#13494=ORIENTED_EDGE ( 'NONE', *, *, #27474, .F. ) ;
#13498=CIRCLE ( 'NONE', #86065, 7.873999999999991672 ) ;
#13532=VERTEX_POINT ( 'NONE', #70481 ) ;
#13576=AXIS2_PLACEMENT_3D ( 'NONE', #20317, #27116, #47542 ) ;
#13582=VERTEX_POINT ( 'NONE', #38624 ) ;
#13598=DIRECTION ( 'NONE',  ( -1.000000000000000000, 0.000000000000000000, 6.982966722218760189E-15 ) ) ;
#13605=EDGE_CURVE ( 'NONE', #53038, #87166, #31362, .T. ) ;
#13619=DIRECTION ( 'NONE',  ( 0.000000000000000000, 0.000000000000000000, -1.000000000000000000 ) ) ;
#13634=CARTESIAN_POINT ( 'NONE',  ( 7.082822281873440318, 72.00847419435602603, 130.3637323515569904 ) ) ;
#13641=CARTESIAN_POINT ( 'NONE',  ( 121.9957511497836578, 45.05269096688547137, -46.49927299628500776 ) ) ;
#13650=LINE ( 'NONE', #7733, #59612 ) ;
#13651=CYLINDRICAL_SURFACE ( 'NONE', #41727, 8.636000000000004562 ) ;
#13659=ORIENTED_EDGE ( 'NONE', *, *, #32760, .F. ) ;
#13693=EDGE_CURVE ( 'NONE', #12149, #40524, #28339, .T. ) ;
#13713=CARTESIAN_POINT ( 'NONE',  ( 0.000000000000000000, 2.031999999999865025, 0.000000000000000000 ) ) ;
#13782=ORIENTED_EDGE ( 'NONE', *, *, #85177, .T. ) ;
#13794=CARTESIAN_POINT ( 'NONE',  ( 0.000000000000000000, 101.5999999999999943, 0.000000000000000000 ) ) ;
#13803=CARTESIAN_POINT ( 'NONE',  ( 12.69999999999999929, 82.54999999999999716, 206.3750000000000000 ) ) ;
#13829=EDGE_LOOP ( 'NONE', ( #60495, #25691, #51213, #8760 ) ) ;
#13869=CARTESIAN_POINT ( 'NONE',  ( -124.2531446105977011, 71.60797102361802047, 40.07553659477990493 ) ) ;
#13888=ORIENTED_EDGE ( 'NONE', *, *, #20174, .T. ) ;
#13889=ORIENTED_EDGE ( 'NONE', *, *, #59013, .F. ) ;
#13896=CARTESIAN_POINT ( 'NONE',  ( -6.118449702233622389, 71.41905655665884467, 130.4126312001327221 ) ) ;
#13914=VERTEX_POINT ( 'NONE', #21782 ) ;
#13916=LINE ( 'NONE', #41595, #82893 ) ;
#13952=ORIENTED_EDGE ( 'NONE', *, *, #80198, .T. ) ;
#13955=CARTESIAN_POINT ( 'NONE',  ( 75.61066417432020614, 0.000000000000000000, 177.0380000000000109 ) ) ;
#13974=AXIS2_PLACEMENT_3D ( 'NONE', #33329, #87852, #12898 ) ;
#13980=VERTEX_POINT ( 'NONE', #59293 ) ;
#13993=EDGE_CURVE ( 'NONE', #76533, #83920, #5209, .T. ) ;
#14028=MECHANICAL_DESIGN_GEOMETRIC_PRESENTATION_REPRESENTATION('',(#72065),#32875);
#14037=DIRECTION ( 'NONE',  ( 0.000000000000000000, -1.000000000000000000, 0.000000000000000000 ) ) ;
#14043=AXIS2_PLACEMENT_3D ( 'NONE', #17452, #80583, #11531 ) ;
#14056=DIRECTION ( 'NONE',  ( 0.000000000000000000, -1.000000000000000000, 0.000000000000000000 ) ) ;
#14057=ORIENTED_EDGE ( 'NONE', *, *, #71275, .F. ) ;
#14078=DIRECTION ( 'NONE',  ( 0.000000000000000000, -1.000000000000000000, 0.000000000000000000 ) ) ;
#14080=CARTESIAN_POINT ( 'NONE',  ( 8.223282282254929854, 72.86292289192388694, 130.2970040361317103 ) ) ;
#14108=AXIS2_PLACEMENT_3D ( 'NONE', #20217, #34273, #61087 ) ;
#14123=LINE ( 'NONE', #47722, #61152 ) ;
#14148=EDGE_LOOP ( 'NONE', ( #14951, #87998, #56877, #40889 ) ) ;
#14151=VECTOR ( 'NONE', #31179, 1000.000000000000000 ) ;
#14152=LINE ( 'NONE', #41386, #37746 ) ;
#14209=EDGE_CURVE ( 'NONE', #13373, #85180, #53078, .T. ) ;
#14244=CARTESIAN_POINT ( 'NONE',  ( 11.87295884493951625, 78.03960220850400731, 130.0150426351353588 ) ) ;
#14269=DIRECTION ( 'NONE',  ( 0.000000000000000000, 0.000000000000000000, 1.000000000000000000 ) ) ;
#14291=VECTOR ( 'NONE', #60704, 1000.000000000000000 ) ;
#14299=DIRECTION ( 'NONE',  ( 0.000000000000000000, 0.000000000000000000, 1.000000000000000000 ) ) ;
#14304=ORIENTED_EDGE ( 'NONE', *, *, #89055, .T. ) ;
#14321=ORIENTED_EDGE ( 'NONE', *, *, #16459, .T. ) ;
#14327=CARTESIAN_POINT ( 'NONE',  ( 3.174999999999889688, 8.255000000000000782, -31.75000000000000000 ) ) ;
#14329=CARTESIAN_POINT ( 'NONE',  ( -114.7490242460955159, 71.13177641138574359, 62.26986715482768631 ) ) ;
#14332=EDGE_CURVE ( 'NONE', #47179, #87166, #31477, .T. ) ;
#14358=DIRECTION ( 'NONE',  ( 0.000000000000000000, -1.000000000000000000, 0.000000000000000000 ) ) ;
#14368=CIRCLE ( 'NONE', #86848, 20.63750000000000284 ) ;
#14384=CARTESIAN_POINT ( 'NONE',  ( 4.665904304751416087E-15, 44.45000000000000284, -38.10000000000000142 ) ) ;
#14393=CARTESIAN_POINT ( 'NONE',  ( 0.000000000000000000, 44.45000000000000284, 0.000000000000000000 ) ) ;
#14402=ADVANCED_FACE ( 'NONE', ( #39194 ), #5126, .T. ) ;
#14411=CYLINDRICAL_SURFACE ( 'NONE', #52885, 6.350000000000659561 ) ;
#14459=DIRECTION ( 'NONE',  ( 0.000000000000000000, 0.000000000000000000, 1.000000000000000000 ) ) ;
#14462=CARTESIAN_POINT ( 'NONE',  ( 0.000000000000000000, 101.5999999999999943, 0.000000000000000000 ) ) ;
#14471=VECTOR ( 'NONE', #70948, 1000.000000000000000 ) ;
#14485=CIRCLE ( 'NONE', #5721, 7.874000000000005883 ) ;
#14488=VECTOR ( 'NONE', #65141, 1000.000000000000000 ) ;
#14538=EDGE_CURVE ( 'NONE', #7104, #54166, #75065, .T. ) ;
#14541=CARTESIAN_POINT ( 'NONE',  ( 5.567800219335068412, 71.13383842984607952, 130.4373048777247561 ) ) ;
#14544=AXIS2_PLACEMENT_3D ( 'NONE', #1274, #62590, #28979 ) ;
#14545=ORIENTED_EDGE ( 'NONE', *, *, #57221, .T. ) ;
#14549=CARTESIAN_POINT ( 'NONE',  ( 120.2492451804830011, 48.02562542861102202, -50.84303487544575262 ) ) ;
#14569=LINE ( 'NONE', #42242, #8490 ) ;
#14570=EDGE_LOOP ( 'NONE', ( #54012, #5837, #6315 ) ) ;
#14587=CARTESIAN_POINT ( 'NONE',  ( -75.61066417432020614, 0.000000000000000000, 177.0380000000000109 ) ) ;
#14607=DIRECTION ( 'NONE',  ( 0.000000000000000000, 1.000000000000000000, 0.000000000000000000 ) ) ;
#14630=CARTESIAN_POINT ( 'NONE',  ( 71.09939861440099662, 101.5999999999999943, 177.8662485265279827 ) ) ;
#14637=AXIS2_PLACEMENT_3D ( 'NONE', #44738, #38824, #3869 ) ;
#14657=ADVANCED_FACE ( 'NONE', ( #82347 ), #35964, .F. ) ;
#14661=CARTESIAN_POINT ( 'NONE',  ( 31.75000000000000000, 17.78000000000000114, 3.174999999999999822 ) ) ;
#14686=FACE_OUTER_BOUND ( 'NONE', #23476, .T. ) ;
#14722=ORIENTED_EDGE ( 'NONE', *, *, #62400, .F. ) ;
#14773=VERTEX_POINT ( 'NONE', #1900 ) ;
#14783=DIRECTION ( 'NONE',  ( 0.000000000000000000, 3.785359618865284342E-16, 1.000000000000000000 ) ) ;
#14784=CARTESIAN_POINT ( 'NONE',  ( -123.0153672541236176, 73.36296953743759275, 43.72751329226351658 ) ) ;
#14805=VECTOR ( 'NONE', #86173, 1000.000000000000000 ) ;
#14825=CARTESIAN_POINT ( 'NONE',  ( 208.9149999999999920, 30.98800000000000310, 44.45000000000000284 ) ) ;
#14863=EDGE_CURVE ( 'NONE', #45672, #66449, #53137, .T. ) ;
#14921=CARTESIAN_POINT ( 'NONE',  ( 109.6604454188727402, 49.07786898089018734, 70.84811965973803183 ) ) ;
#14951=ORIENTED_EDGE ( 'NONE', *, *, #84885, .F. ) ;
#14964=DIRECTION ( 'NONE',  ( 0.000000000000000000, 0.000000000000000000, -1.000000000000000000 ) ) ;
#14989=VERTEX_POINT ( 'NONE', #81784 ) ;
#15019=CARTESIAN_POINT ( 'NONE',  ( 125.1553824804045547, 69.48256747448400006, 37.16550212950143361 ) ) ;
#15023=ORIENTED_EDGE ( 'NONE', *, *, #59717, .T. ) ;
#15045=CARTESIAN_POINT ( 'NONE',  ( 170.2205283966864897, 101.5999999999999943, -71.37400000000000944 ) ) ;
#15047=CARTESIAN_POINT ( 'NONE',  ( -31.75000000000000000, 24.56180297284579694, 3.175000000000219647 ) ) ;
#15050=DIRECTION ( 'NONE',  ( 0.9347835805883503157, 0.000000000000000000, -0.3552177606235690788 ) ) ;
#15095=LINE ( 'NONE', #53814, #58334 ) ;
#15110=EDGE_CURVE ( 'NONE', #56957, #60012, #49009, .T. ) ;
#15246=AXIS2_PLACEMENT_3D ( 'NONE', #20633, #83761, #14269 ) ;
#15252=CARTESIAN_POINT ( 'NONE',  ( 147.4575741623265799, 101.5999999999999943, 135.2444258376725941 ) ) ;
#15281=ORIENTED_EDGE ( 'NONE', *, *, #68593, .F. ) ;
#15298=ORIENTED_EDGE ( 'NONE', *, *, #51185, .F. ) ;
#15309=CARTESIAN_POINT ( 'NONE',  ( -12.69999999999999929, 82.54999999999999716, 129.9368274816650057 ) ) ;
#15311=CARTESIAN_POINT ( 'NONE',  ( 148.0533267522752112, 20.32000000000000028, 160.2664750769284865 ) ) ;
#15324=ORIENTED_EDGE ( 'NONE', *, *, #24595, .T. ) ;
#15347=ORIENTED_EDGE ( 'NONE', *, *, #16459, .F. ) ;
#15360=CARTESIAN_POINT ( 'NONE',  ( 21.94694372886773337, 60.27287744939596337, 31.14430251170410457 ) ) ;
#15364=PLANE ( 'NONE',  #17972 ) ;
#15372=CARTESIAN_POINT ( 'NONE',  ( -18.25522102001837155, 65.15566424648996247, 33.44615533302457777 ) ) ;
#15398=EDGE_CURVE ( 'NONE', #47018, #31056, #72313, .T. ) ;
#15448=CARTESIAN_POINT ( 'NONE',  ( 125.0134529257903893, 48.65659782722526217, -37.63673439681842581 ) ) ;
#15464=EDGE_CURVE ( 'NONE', #43342, #41931, #4888, .T. ) ;
#15480=CARTESIAN_POINT ( 'NONE',  ( 126.4548149396404710, 63.48030817387711977, 32.46806497751565956 ) ) ;
#15508=AXIS2_PLACEMENT_3D ( 'NONE', #64861, #44396, #65309 ) ;
#15522=VERTEX_POINT ( 'NONE', #78455 ) ;
#15564=EDGE_LOOP ( 'NONE', ( #40992, #83711, #76749, #66777 ) ) ;
#15569=ORIENTED_EDGE ( 'NONE', *, *, #68094, .F. ) ;
#15604=CIRCLE ( 'NONE', #47469, 20.63750000000000284 ) ;
#15664=EDGE_LOOP ( 'NONE', ( #38777, #45392, #61313, #4338 ) ) ;
#15670=AXIS2_PLACEMENT_3D ( 'NONE', #20750, #48422, #76160 ) ;
#15683=ORIENTED_EDGE ( 'NONE', *, *, #22398, .T. ) ;
#15708=DIRECTION ( 'NONE',  ( 0.000000000000000000, 0.000000000000000000, 1.000000000000000000 ) ) ;
#15709=FACE_OUTER_BOUND ( 'NONE', #84617, .T. ) ;
#15725=VERTEX_POINT ( 'NONE', #87483 ) ;
#15734=ORIENTED_EDGE ( 'NONE', *, *, #3028, .T. ) ;
#15756=EDGE_CURVE ( 'NONE', #51663, #21659, #13412, .T. ) ;
#15765=FACE_OUTER_BOUND ( 'NONE', #19033, .T. ) ;
#15771=EDGE_CURVE ( 'NONE', #28030, #11013, #46706, .T. ) ;
#15805=CARTESIAN_POINT ( 'NONE',  ( 23.27731929905161223, 53.97500000000000142, 30.16249999999999076 ) ) ;
#15821=LINE ( 'NONE', #43496, #23380 ) ;
#15838=CARTESIAN_POINT ( 'NONE',  ( 3.110602869834275287E-15, 2.031999999999865025, -25.39999999999999858 ) ) ;
#15856=ORIENTED_EDGE ( 'NONE', *, *, #54472, .F. ) ;
#15868=CARTESIAN_POINT ( 'NONE',  ( 0.000000000000000000, 114.2999999999999972, 0.000000000000000000 ) ) ;
#15881=CARTESIAN_POINT ( 'NONE',  ( -21.12245462538188079, 46.12462447032474699, 31.70988376339461112 ) ) ;
#15882=LINE ( 'NONE', #79458, #82231 ) ;
#15889=ORIENTED_EDGE ( 'NONE', *, *, #242, .F. ) ;
#15892=ORIENTED_EDGE ( 'NONE', *, *, #87439, .F. ) ;
#15897=LINE ( 'NONE', #23617, #32693 ) ;
#15920=CARTESIAN_POINT ( 'NONE',  ( 125.9597867034675573, 66.44223047789067493, 34.33911078552125673 ) ) ;
#15941=PLANE ( 'NONE',  #18010 ) ;
#15950=VECTOR ( 'NONE', #21904, 1000.000000000000000 ) ;
#15951=EDGE_CURVE ( 'NONE', #64336, #42621, #15095, .T. ) ;
#15957=CARTESIAN_POINT ( 'NONE',  ( -147.4575741623270062, 0.000000000000000000, 135.2444258376732193 ) ) ;
#15984=DIRECTION ( 'NONE',  ( -1.514143847546114723E-15, -0.8660254037844387076, 0.4999999999999998890 ) ) ;
#15997=VERTEX_POINT ( 'NONE', #64144 ) ;
#16001=VERTEX_POINT ( 'NONE', #58214 ) ;
#16032=VECTOR ( 'NONE', #32667, 1000.000000000000000 ) ;
#16041=CARTESIAN_POINT ( 'NONE',  ( 11.80314539778289529, 77.86161004085525406, 130.0213727849707368 ) ) ;
#16048=AXIS2_PLACEMENT_3D ( 'NONE', #52262, #65486, #80028 ) ;
#16061=ADVANCED_FACE ( 'NONE', ( #79571 ), #65474, .F. ) ;
#16067=CARTESIAN_POINT ( 'NONE',  ( 7.008108505301582802, 93.14135335536794003, 130.3677710664748020 ) ) ;
#16077=CARTESIAN_POINT ( 'NONE',  ( 0.000000000000000000, 1.270000000000000018, 0.000000000000000000 ) ) ;
#16177=ORIENTED_EDGE ( 'NONE', *, *, #76388, .F. ) ;
#16196=CARTESIAN_POINT ( 'NONE',  ( 173.9900000000000091, 20.32000000000000028, 131.6533725204182019 ) ) ;
#16204=CARTESIAN_POINT ( 'NONE',  ( -7.061405134937971617, 93.10587809510549562, 130.3648943659824795 ) ) ;
#16221=DIRECTION ( 'NONE',  ( 0.000000000000000000, 0.000000000000000000, 1.000000000000000000 ) ) ;
#16225=CIRCLE ( 'NONE', #78622, 7.873999999999991672 ) ;
#16250=CARTESIAN_POINT ( 'NONE',  ( -160.2664750769294812, 20.32000000000000028, -148.0533267522755807 ) ) ;
#16267=ORIENTED_EDGE ( 'NONE', *, *, #37185, .T. ) ;
#16271=DIRECTION ( 'NONE',  ( 1.000000000000000000, 0.000000000000000000, -1.047445008332813989E-14 ) ) ;
#16314=DIRECTION ( 'NONE',  ( 0.000000000000000000, 1.000000000000000000, 0.000000000000000000 ) ) ;
#16331=ORIENTED_EDGE ( 'NONE', *, *, #87439, .T. ) ;
#16339=CARTESIAN_POINT ( 'NONE',  ( -179.8898777604655095, 0.000000000000000000, 114.2999999999999972 ) ) ;
#16350=ORIENTED_EDGE ( 'NONE', *, *, #46365, .F. ) ;
#16364=CARTESIAN_POINT ( 'NONE',  ( 127.0154160123110927, 55.38930970734350723, 30.19865483100764791 ) ) ;
#16378=CYLINDRICAL_SURFACE ( 'NONE', #37506, 20.63750000000000284 ) ;
#16387=CARTESIAN_POINT ( 'NONE',  ( -141.3509999999999991, 0.000000000000000000, 141.3509999999999991 ) ) ;
#16414=ORIENTED_EDGE ( 'NONE', *, *, #40552, .F. ) ;
#16435=DIRECTION ( 'NONE',  ( 0.000000000000000000, 0.000000000000000000, 1.000000000000000000 ) ) ;
#16442=AXIS2_PLACEMENT_3D ( 'NONE', #48205, #35038, #55462 ) ;
#16459=EDGE_CURVE ( 'NONE', #31056, #47018, #53695, .T. ) ;
#16506=CARTESIAN_POINT ( 'NONE',  ( 0.7862675091416512219, 95.25000000000004263, 130.5560000000000684 ) ) ;
#16520=ORIENTED_EDGE ( 'NONE', *, *, #12476, .F. ) ;
#16585=ORIENTED_EDGE ( 'NONE', *, *, #63824, .T. ) ;
#16634=LINE ( 'NONE', #72045, #78114 ) ;
#16643=CARTESIAN_POINT ( 'NONE',  ( -5.570957693668114885, 93.96460761459663047, 130.4371699319834761 ) ) ;
#16659=FACE_OUTER_BOUND ( 'NONE', #42642, .T. ) ;
#16666=VERTEX_POINT ( 'NONE', #27159 ) ;
#16712=DIRECTION ( 'NONE',  ( 1.514143847546114723E-15, -0.8660254037844387076, -0.4999999999999998890 ) ) ;
#16730=CARTESIAN_POINT ( 'NONE',  ( 183.5150000000000148, 53.21300000000000097, 41.63456447661469895 ) ) ;
#16771=DIRECTION ( 'NONE',  ( 0.000000000000000000, -1.000000000000000000, 0.000000000000000000 ) ) ;
#16798=CARTESIAN_POINT ( 'NONE',  ( 0.000000000000000000, 8.255000000000000782, 0.000000000000000000 ) ) ;
#16808=CARTESIAN_POINT ( 'NONE',  ( 113.3231070055411323, 69.11259796942169942, 64.82881333974782478 ) ) ;
#16819=ORIENTED_EDGE ( 'NONE', *, *, #14209, .T. ) ;
#16820=DIRECTION ( 'NONE',  ( 0.000000000000000000, 1.000000000000000000, 0.000000000000000000 ) ) ;
#16882=CYLINDRICAL_SURFACE ( 'NONE', #18098, 12.69999999999998863 ) ;
#16965=VERTEX_POINT ( 'NONE', #89698 ) ;
#16968=ADVANCED_FACE ( 'NONE', ( #62859, #47876 ), #42407, .T. ) ;
#17005=CIRCLE ( 'NONE', #40192, 9.425000000000000711 ) ;
#17010=EDGE_LOOP ( 'NONE', ( #66539, #87674, #88983, #65753 ) ) ;
#17070=CARTESIAN_POINT ( 'NONE',  ( 0.000000000000000000, 1.270000000000000018, 24.63800000000000168 ) ) ;
#17084=DIRECTION ( 'NONE',  ( -0.7071067811865360264, 0.000000000000000000, 0.7071067811865588970 ) ) ;
#17088=CARTESIAN_POINT ( 'NONE',  ( -7.079787210858614621, 93.09356445001880331, 130.3638972052411589 ) ) ;
#17098=DIRECTION ( 'NONE',  ( 1.000000000000000000, 0.000000000000000000, 0.000000000000000000 ) ) ;
#17104=ORIENTED_EDGE ( 'NONE', *, *, #75206, .T. ) ;
#17108=ORIENTED_EDGE ( 'NONE', *, *, #17802, .T. ) ;
#17128=DIRECTION ( 'NONE',  ( -0.7071067811865580088, 0.000000000000000000, -0.7071067811865370256 ) ) ;
#17131=AXIS2_PLACEMENT_3D ( 'NONE', #40473, #68636, #26838 ) ;
#17193=EDGE_CURVE ( 'NONE', #35428, #83920, #1593, .T. ) ;
#17226=ORIENTED_EDGE ( 'NONE', *, *, #64872, .F. ) ;
#17233=DIRECTION ( 'NONE',  ( 0.000000000000000000, 0.000000000000000000, -1.000000000000000000 ) ) ;
#17256=CARTESIAN_POINT ( 'NONE',  ( 111.6005515524849017, 65.74677178836266478, 67.75091760821770492 ) ) ;
#17284=DIRECTION ( 'NONE',  ( 1.000000000000000000, 0.000000000000000000, 0.000000000000000000 ) ) ;
#17305=EDGE_CURVE ( 'NONE', #69846, #59397, #61429, .T. ) ;
#17335=ORIENTED_EDGE ( 'NONE', *, *, #62400, .T. ) ;
#17362=CARTESIAN_POINT ( 'NONE',  ( -194.1576000000000022, 101.5999999999999943, 114.2999999999999972 ) ) ;
#17431=FACE_OUTER_BOUND ( 'NONE', #59777, .T. ) ;
#17452=CARTESIAN_POINT ( 'NONE',  ( 0.000000000000000000, 20.32000000000000028, 0.000000000000000000 ) ) ;
#17463=FACE_OUTER_BOUND ( 'NONE', #69926, .T. ) ;
#17481=DIRECTION ( 'NONE',  ( 1.000000000000000000, 0.000000000000000000, 2.108231265501709878E-16 ) ) ;
#17490=VERTEX_POINT ( 'NONE', #17878 ) ;
#17502=EDGE_CURVE ( 'NONE', #52020, #36552, #83255, .T. ) ;
#17515=AXIS2_PLACEMENT_3D ( 'NONE', #63644, #56809, #84557 ) ;
#17521=AXIS2_PLACEMENT_3D ( 'NONE', #36817, #16820, #18592 ) ;
#17529=AXIS2_PLACEMENT_3D ( 'NONE', #19359, #39346, #67052 ) ;
#17531=EDGE_CURVE ( 'NONE', #28246, #72639, #7387, .T. ) ;
#17548=VERTEX_POINT ( 'NONE', #14661 ) ;
#17559=ORIENTED_EDGE ( 'NONE', *, *, #83652, .T. ) ;
#17582=CARTESIAN_POINT ( 'NONE',  ( -123.4696824136392053, 101.5999999999999943, -179.8898777604655095 ) ) ;
#17626=EDGE_CURVE ( 'NONE', #121, #39820, #58646, .T. ) ;
#17639=DIRECTION ( 'NONE',  ( 0.000000000000000000, 0.8660254037844387076, 0.4999999999999998890 ) ) ;
#17651=CARTESIAN_POINT ( 'NONE',  ( 119.9576544348878713, 56.34114634768905461, -51.52716989460228802 ) ) ;
#17659=ADVANCED_FACE ( 'NONE', ( #9188 ), #1625, .F. ) ;
#17672=LINE ( 'NONE', #65803, #68180 ) ;
#17679=ORIENTED_EDGE ( 'NONE', *, *, #64355, .F. ) ;
#17696=CARTESIAN_POINT ( 'NONE',  ( 109.5717151936057689, 58.27256190523081614, 70.98527193250401979 ) ) ;
#17711=CARTESIAN_POINT ( 'NONE',  ( 0.000000000000000000, 1.270000000000000018, 0.000000000000000000 ) ) ;
#17712=CARTESIAN_POINT ( 'NONE',  ( 131.3179999999999836, 53.97500000000000142, 50.79999999999999716 ) ) ;
#17717=AXIS2_PLACEMENT_3D ( 'NONE', #38892, #80701, #87506 ) ;
#17761=CIRCLE ( 'NONE', #6165, 9.425000000000000711 ) ;
#17802=EDGE_CURVE ( 'NONE', #34850, #58230, #30593, .T. ) ;
#17846=EDGE_LOOP ( 'NONE', ( #40483, #39610, #4578, #48191, #88738, #81816, #59550, #36097 ) ) ;
#17859=CARTESIAN_POINT ( 'NONE',  ( 173.9900000000000091, 101.5999999999999943, 131.6533725204182019 ) ) ;
#17872=LINE ( 'NONE', #81024, #22663 ) ;
#17878=CARTESIAN_POINT ( 'NONE',  ( 23.27731929905161223, 53.97500000000000142, 30.16249999999999076 ) ) ;
#17883=DIRECTION ( 'NONE',  ( 0.000000000000000000, 0.000000000000000000, -1.000000000000000000 ) ) ;
#17885=VERTEX_POINT ( 'NONE', #20022 ) ;
#17888=DIRECTION ( 'NONE',  ( 0.000000000000000000, 0.000000000000000000, 1.000000000000000000 ) ) ;
#17892=VECTOR ( 'NONE', #61903, 1000.000000000000000 ) ;
#17917=FACE_OUTER_BOUND ( 'NONE', #32518, .T. ) ;
#17972=AXIS2_PLACEMENT_3D ( 'NONE', #51190, #37587, #85312 ) ;
#17975=ORIENTED_EDGE ( 'NONE', *, *, #50001, .T. ) ;
#17988=CARTESIAN_POINT ( 'NONE',  ( -111.4783850760235566, 65.45264025789361995, 67.95177877341511419 ) ) ;
#18001=EDGE_CURVE ( 'NONE', #69846, #22712, #62237, .T. ) ;
#18010=AXIS2_PLACEMENT_3D ( 'NONE', #36826, #50891, #56802 ) ;
#18015=CARTESIAN_POINT ( 'NONE',  ( -0.7859308033515303160, 69.84999999999996589, 130.5560000000000684 ) ) ;
#18028=EDGE_CURVE ( 'NONE', #47532, #51892, #13650, .T. ) ;
#18059=VERTEX_POINT ( 'NONE', #28618 ) ;
#18070=ORIENTED_EDGE ( 'NONE', *, *, #22845, .T. ) ;
#18082=CARTESIAN_POINT ( 'NONE',  ( 119.5843592605237120, 52.73749999999999716, -52.38749999999991758 ) ) ;
#18090=EDGE_CURVE ( 'NONE', #3666, #52538, #23618, .T. ) ;
#18096=ORIENTED_EDGE ( 'NONE', *, *, #28357, .F. ) ;
#18097=DIRECTION ( 'NONE',  ( -0.000000000000000000, 1.000000000000000000, 0.000000000000000000 ) ) ;
#18098=AXIS2_PLACEMENT_3D ( 'NONE', #51817, #9613, #66349 ) ;
#18101=VECTOR ( 'NONE', #71700, 1000.000000000000000 ) ;
#18130=CARTESIAN_POINT ( 'NONE',  ( 109.2774118001977541, 55.39176648947218240, 71.43749999999998579 ) ) ;
#18157=DIRECTION ( 'NONE',  ( 0.000000000000000000, 0.000000000000000000, 1.000000000000000000 ) ) ;
#18158=DIRECTION ( 'NONE',  ( 0.000000000000000000, 0.000000000000000000, 1.000000000000000000 ) ) ;
#18166=AXIS2_PLACEMENT_3D ( 'NONE', #6569, #67443, #11606 ) ;
#18208=DIRECTION ( 'NONE',  ( 0.000000000000000000, 1.000000000000000000, 0.000000000000000000 ) ) ;
#18248=LINE ( 'NONE', #17362, #77773 ) ;
#18252=ORIENTED_EDGE ( 'NONE', *, *, #30569, .T. ) ;
#18273=ORIENTED_EDGE ( 'NONE', *, *, #27630, .T. ) ;
#18291=AXIS2_PLACEMENT_3D ( 'NONE', #76739, #48107, #62205 ) ;
#18318=CARTESIAN_POINT ( 'NONE',  ( 160.2664750769284865, 0.000000000000000000, -148.0533267522753818 ) ) ;
#18319=VERTEX_POINT ( 'NONE', #6277 ) ;
#18354=CARTESIAN_POINT ( 'NONE',  ( -0.6929090906571917508, 70.24203434096085630, 38.09999999999997300 ) ) ;
#18366=CARTESIAN_POINT ( 'NONE',  ( 55.48342271751659638, 20.32000000000000028, 171.1197181046785261 ) ) ;
#18383=VERTEX_POINT ( 'NONE', #37123 ) ;
#18395=ORIENTED_EDGE ( 'NONE', *, *, #32327, .F. ) ;
#18414=CARTESIAN_POINT ( 'NONE',  ( 126.6848757172646884, 46.51586155035142411, 31.55656739648512854 ) ) ;
#18422=VERTEX_POINT ( 'NONE', #8980 ) ;
#18423=VERTEX_POINT ( 'NONE', #85736 ) ;
#18448=FACE_BOUND ( 'NONE', #51598, .T. ) ;
#18461=CARTESIAN_POINT ( 'NONE',  ( -3.228675327066591105, 70.25984576160145423, 130.5164141216791904 ) ) ;
#18491=VERTEX_POINT ( 'NONE', #22164 ) ;
#18495=DIRECTION ( 'NONE',  ( 0.000000000000000000, -1.000000000000000000, 0.000000000000000000 ) ) ;
#18498=AXIS2_PLACEMENT_3D ( 'NONE', #33982, #76225, #369 ) ;
#18527=EDGE_LOOP ( 'NONE', ( #57992, #55530, #54668, #76475 ) ) ;
#18530=CARTESIAN_POINT ( 'NONE',  ( 122.5474368815848578, 60.65832587247668783, -45.02295694080569888 ) ) ;
#18549=VECTOR ( 'NONE', #85535, 1000.000000000000000 ) ;
#18555=ORIENTED_EDGE ( 'NONE', *, *, #67638, .F. ) ;
#18569=DIRECTION ( 'NONE',  ( 0.000000000000000000, 0.000000000000000000, -1.000000000000000000 ) ) ;
#18570=DIRECTION ( 'NONE',  ( 0.000000000000000000, 1.000000000000000000, 0.000000000000000000 ) ) ;
#18579=CARTESIAN_POINT ( 'NONE',  ( 111.6427491051048122, 65.84630886252570292, 67.68135981035700866 ) ) ;
#18592=DIRECTION ( 'NONE',  ( 0.000000000000000000, 0.000000000000000000, 1.000000000000000000 ) ) ;
#18616=DIRECTION ( 'NONE',  ( 1.825781832977094175E-16, -0.4999999999999998890, -0.8660254037844387076 ) ) ;
#18628=FACE_OUTER_BOUND ( 'NONE', #82184, .T. ) ;
#18645=CARTESIAN_POINT ( 'NONE',  ( 0.000000000000000000, 44.45000000000000284, 0.000000000000000000 ) ) ;
#18658=CIRCLE ( 'NONE', #86815, 20.63750000000000284 ) ;
#18673=ORIENTED_EDGE ( 'NONE', *, *, #39658, .F. ) ;
#18690=VECTOR ( 'NONE', #54930, 1000.000000000000000 ) ;
#18700=DIRECTION ( 'NONE',  ( 0.000000000000000000, -1.000000000000000000, 0.000000000000000000 ) ) ;
#18729=LINE ( 'NONE', #54557, #12361 ) ;
#18749=DIRECTION ( 'NONE',  ( -1.000000000000000000, 0.000000000000000000, -7.867884063170659983E-16 ) ) ;
#18756=CARTESIAN_POINT ( 'NONE',  ( 0.000000000000000000, 0.000000000000000000, 0.000000000000000000 ) ) ;
#18790=EDGE_LOOP ( 'NONE', ( #29323, #29305, #83369, #77542 ) ) ;
#18817=LINE ( 'NONE', #33340, #83094 ) ;
#18855=AXIS2_PLACEMENT_3D ( 'NONE', #19089, #26355, #11835 ) ;
#18923=PLANE ( 'NONE',  #53868 ) ;
#18926=ORIENTED_EDGE ( 'NONE', *, *, #75353, .F. ) ;
#18930=CARTESIAN_POINT ( 'NONE',  ( -185.9961463128564958, 101.5999999999999943, -3.174999999999514877 ) ) ;
#18941=CARTESIAN_POINT ( 'NONE',  ( 0.000000000000000000, 114.2999999999999972, -9.525000000000000355 ) ) ;
#18986=CARTESIAN_POINT ( 'NONE',  ( 1.154229608196380665E-15, 125.7300000000000040, 9.425000000000000711 ) ) ;
#18989=CARTESIAN_POINT ( 'NONE',  ( 124.3618578197163771, 59.12976082637415942, -39.73717948323967164 ) ) ;
#19016=ORIENTED_EDGE ( 'NONE', *, *, #82429, .F. ) ;
#19033=EDGE_LOOP ( 'NONE', ( #81166, #85326, #20636, #41377 ) ) ;
#19042=VERTEX_POINT ( 'NONE', #44253 ) ;
#19056=ORIENTED_EDGE ( 'NONE', *, *, #4980, .T. ) ;
#19069=AXIS2_PLACEMENT_3D ( 'NONE', #60919, #68194, #27743 ) ;
#19089=CARTESIAN_POINT ( 'NONE',  ( -215.9000000000000057, 53.97500000000000142, 50.79999999999999716 ) ) ;
#19098=CARTESIAN_POINT ( 'NONE',  ( 196.2150000000000034, 30.98800000000000310, 57.14999999999999858 ) ) ;
#19121=EDGE_CURVE ( 'NONE', #13980, #48446, #47271, .T. ) ;
#19136=VERTEX_POINT ( 'NONE', #28175 ) ;
#19171=ORIENTED_EDGE ( 'NONE', *, *, #15398, .T. ) ;
#19190=DIRECTION ( 'NONE',  ( 0.000000000000000000, -1.000000000000000000, 0.000000000000000000 ) ) ;
#19202=DIRECTION ( 'NONE',  ( 1.000000000000000000, 0.000000000000000000, 0.000000000000000000 ) ) ;
#19205=CARTESIAN_POINT ( 'NONE',  ( 1.166476076187854022E-15, 1.270000000000000018, 9.525000000000000355 ) ) ;
#19217=CARTESIAN_POINT ( 'NONE',  ( -179.8898777604659927, 20.32000000000000028, -123.4696824136383952 ) ) ;
#19256=EDGE_CURVE ( 'NONE', #18423, #39686, #55421, .T. ) ;
#19265=DIRECTION ( 'NONE',  ( 0.000000000000000000, 0.000000000000000000, 1.000000000000000000 ) ) ;
#19276=FACE_OUTER_BOUND ( 'NONE', #65541, .T. ) ;
#19277=ADVANCED_FACE ( 'NONE', ( #44931 ), #44485, .T. ) ;
#19297=CARTESIAN_POINT ( 'NONE',  ( -187.8075999999999794, 0.000000000000000000, 107.9500000000000028 ) ) ;
#19304=VERTEX_POINT ( 'NONE', #71331 ) ;
#19342=CARTESIAN_POINT ( 'NONE',  ( -111.1819842745013460, 64.70253472953531571, 68.43619979767439077 ) ) ;
#19346=CYLINDRICAL_SURFACE ( 'NONE', #24601, 8.636000000000004562 ) ;
#19350=EDGE_CURVE ( 'NONE', #47179, #72757, #46254, .T. ) ;
#19359=CARTESIAN_POINT ( 'NONE',  ( 0.000000000000000000, 2.270000000000000462, 0.000000000000000000 ) ) ;
#19377=DIRECTION ( 'NONE',  ( 1.000000000000000000, 0.000000000000000000, 0.000000000000000000 ) ) ;
#19395=ORIENTED_EDGE ( 'NONE', *, *, #53557, .F. ) ;
#19428=ADVANCED_FACE ( 'NONE', ( #87183 ), #80825, .T. ) ;
#19459=CARTESIAN_POINT ( 'NONE',  ( 0.000000000000000000, 20.32000000000000028, 0.000000000000000000 ) ) ;
#19463=CARTESIAN_POINT ( 'NONE',  ( -148.0533267522759786, 0.000000000000000000, -160.2664750769289697 ) ) ;
#19485=DIRECTION ( 'NONE',  ( 1.000000000000000000, 0.000000000000000000, 0.000000000000000000 ) ) ;
#19499=CARTESIAN_POINT ( 'NONE',  ( 183.5150000000000148, 37.33800000000000097, 32.46912895322940074 ) ) ;
#19507=CARTESIAN_POINT ( 'NONE',  ( -186.2398777604655038, 101.5999999999999943, -6.349999999999999645 ) ) ;
#19517=ORIENTED_EDGE ( 'NONE', *, *, #28654, .F. ) ;
#19527=VECTOR ( 'NONE', #11399, 1000.000000000000000 ) ;
#19543=( NAMED_UNIT ( * ) SI_UNIT ( $, .STERADIAN. ) SOLID_ANGLE_UNIT ( ) );
#19547=CYLINDRICAL_SURFACE ( 'NONE', #5668, 9.425000000000000711 ) ;
#19548=CARTESIAN_POINT ( 'NONE',  ( 7.069959413120197489, 71.99984796920048780, 130.3644307161663107 ) ) ;
#19557=VERTEX_POINT ( 'NONE', #38130 ) ;
#19558=EDGE_CURVE ( 'NONE', #57167, #31769, #30335, .T. ) ;
#19562=DIRECTION ( 'NONE',  ( 0.000000000000000000, 1.000000000000000000, 0.000000000000000000 ) ) ;
#19622=CARTESIAN_POINT ( 'NONE',  ( 10.54391646024738627, 89.62925550596948199, 130.1295316605823871 ) ) ;
#19627=CARTESIAN_POINT ( 'NONE',  ( -186.2398777604655038, 0.000000000000000000, 114.2999999999999972 ) ) ;
#19649=LINE ( 'NONE', #69149, #83762 ) ;
#19661=CARTESIAN_POINT ( 'NONE',  ( -158.9822249764580135, 20.32000000000000028, 107.9500000000000028 ) ) ;
#19670=EDGE_CURVE ( 'NONE', #84394, #25618, #35328, .T. ) ;
#19672=ADVANCED_FACE ( 'NONE', ( #371 ), #42139, .T. ) ;
#19709=PLANE ( 'NONE',  #71483 ) ;
#19724=CARTESIAN_POINT ( 'NONE',  ( 0.000000000000000000, 0.000000000000000000, 0.000000000000000000 ) ) ;
#19788=CARTESIAN_POINT ( 'NONE',  ( -109.6498392670675628, 58.85328883199191097, 70.86473263594878347 ) ) ;
#19817=CARTESIAN_POINT ( 'NONE',  ( -11.66942133526382008, 77.53815898108125282, 130.0334386654385526 ) ) ;
#19823=DIRECTION ( 'NONE',  ( -0.7071067811865480168, 0.000000000000000000, 0.7071067811865470176 ) ) ;
#19824=LINE ( 'NONE', #67073, #1777 ) ;
#19842=ORIENTED_EDGE ( 'NONE', *, *, #73612, .T. ) ;
#19889=ORIENTED_EDGE ( 'NONE', *, *, #1736, .T. ) ;
#19927=FACE_OUTER_BOUND ( 'NONE', #89247, .T. ) ;
#19937=CARTESIAN_POINT ( 'NONE',  ( 110.7653435595065901, 44.45000000000000284, 69.10794311903988785 ) ) ;
#19938=CARTESIAN_POINT ( 'NONE',  ( -186.2398777604659870, 0.000000000000000000, 107.9500000000000028 ) ) ;
#19951=AXIS2_PLACEMENT_3D ( 'NONE', #18756, #33283, #82350 ) ;
#19975=VERTEX_POINT ( 'NONE', #72554 ) ;
#20006=CARTESIAN_POINT ( 'NONE',  ( 50.03799999999999670, 20.32000000000000028, 191.3008000794699797 ) ) ;
#20022=CARTESIAN_POINT ( 'NONE',  ( 0.000000000000000000, 11.98343896644750117, -160.4955849403809793 ) ) ;
#20029=AXIS2_PLACEMENT_3D ( 'NONE', #41424, #21005, #83688 ) ;
#20041=CARTESIAN_POINT ( 'NONE',  ( -50.03799999999999670, 101.5999999999999943, 178.6098374884404905 ) ) ;
#20052=FACE_OUTER_BOUND ( 'NONE', #85822, .T. ) ;
#20065=VECTOR ( 'NONE', #3686, 1000.000000000000000 ) ;
#20080=CARTESIAN_POINT ( 'NONE',  ( 131.3179999999999836, 53.97500000000000142, 50.79999999999999716 ) ) ;
#20085=CARTESIAN_POINT ( 'NONE',  ( 7.037613089623343754, 93.12175551049465128, 130.3661809698470506 ) ) ;
#20156=VECTOR ( 'NONE', #56938, 1000.000000000000000 ) ;
#20174=EDGE_CURVE ( 'NONE', #31769, #76607, #36218, .T. ) ;
#20196=CARTESIAN_POINT ( 'NONE',  ( 23.12708505997960629, 51.75119301488568624, 30.27798919810780731 ) ) ;
#20202=EDGE_CURVE ( 'NONE', #78334, #73595, #73949, .T. ) ;
#20213=DIRECTION ( 'NONE',  ( 0.000000000000000000, 1.000000000000000000, 0.000000000000000000 ) ) ;
#20216=AXIS2_PLACEMENT_3D ( 'NONE', #24508, #38566, #31754 ) ;
#20217=CARTESIAN_POINT ( 'NONE',  ( 0.000000000000000000, 0.000000000000000000, 0.000000000000000000 ) ) ;
#20222=ORIENTED_EDGE ( 'NONE', *, *, #15398, .F. ) ;
#20224=LINE ( 'NONE', #34734, #54574 ) ;
#20235=ORIENTED_EDGE ( 'NONE', *, *, #5558, .F. ) ;
#20241=CARTESIAN_POINT ( 'NONE',  ( 0.000000000000000000, 125.7300000000000040, 0.000000000000000000 ) ) ;
#20242=CARTESIAN_POINT ( 'NONE',  ( -115.0751651833283233, 71.53075230113380201, 61.66802841283988101 ) ) ;
#20259=COLOUR_RGB ( '', 0.72549020, 0.75294118, 0.79215686) ;
#20261=CARTESIAN_POINT ( 'NONE',  ( -50.03799999999999670, 20.32000000000000028, 191.3008000794699797 ) ) ;
#20262=VERTEX_POINT ( 'NONE', #6197 ) ;
#20268=CARTESIAN_POINT ( 'NONE',  ( 50.03799999999999670, 20.32000000000000028, 178.6098374884404905 ) ) ;
#20271=EDGE_CURVE ( 'NONE', #6343, #5474, #29330, .T. ) ;
#20275=CARTESIAN_POINT ( 'NONE',  ( -10.38944306109878646, 75.24551383372960345, 130.1420047866670870 ) ) ;
#20279=CARTESIAN_POINT ( 'NONE',  ( -179.6544565346565037, 101.5999999999999943, -9.200237383489920262 ) ) ;
#20286=CARTESIAN_POINT ( 'NONE',  ( -55.11501535285000131, 20.32000000000000028, 183.9403141659174992 ) ) ;
#20300=DIRECTION ( 'NONE',  ( -1.000000000000000000, 0.000000000000000000, 0.000000000000000000 ) ) ;
#20313=ADVANCED_FACE ( 'NONE', ( #7978 ), #56100, .F. ) ;
#20317=CARTESIAN_POINT ( 'NONE',  ( 141.3509999999999991, 20.32000000000000028, 141.3509999999999991 ) ) ;
#20318=EDGE_CURVE ( 'NONE', #10839, #46235, #20340, .T. ) ;
#20330=VECTOR ( 'NONE', #32389, 1000.000000000000000 ) ;
#20334=VERTEX_POINT ( 'NONE', #83848 ) ;
#20340=CIRCLE ( 'NONE', #85652, 130.5560000000000116 ) ;
#20342=EDGE_LOOP ( 'NONE', ( #63834, #25274, #83668, #29038 ) ) ;
#20361=CARTESIAN_POINT ( 'NONE',  ( 148.0533267522749838, 101.5999999999999943, -160.2664750769289697 ) ) ;
#20419=AXIS2_PLACEMENT_3D ( 'NONE', #2688, #16314, #58083 ) ;
#20431=ORIENTED_EDGE ( 'NONE', *, *, #75245, .F. ) ;
#20433=CARTESIAN_POINT ( 'NONE',  ( -186.2398777604655038, 20.32000000000000028, 114.2999999999999972 ) ) ;
#20451=AXIS2_PLACEMENT_3D ( 'NONE', #34890, #60803, #47612 ) ;
#20456=LINE ( 'NONE', #34057, #34692 ) ;
#20458=CARTESIAN_POINT ( 'NONE',  ( 5.749594899366220702, 71.22412605658588802, 130.4294147092975606 ) ) ;
#20483=CARTESIAN_POINT ( 'NONE',  ( 126.4481529151155996, 44.45000000000000284, 32.49205688096009936 ) ) ;
#20515=( LENGTH_UNIT ( ) NAMED_UNIT ( * ) SI_UNIT ( .MILLI., .METRE. ) );
#20522=DIRECTION ( 'NONE',  ( 0.000000000000000000, 1.000000000000000000, 0.000000000000000000 ) ) ;
#20540=DIRECTION ( 'NONE',  ( 0.000000000000000000, 1.000000000000000000, 0.000000000000000000 ) ) ;
#20545=EDGE_LOOP ( 'NONE', ( #75381, #81751, #26586, #50981 ) ) ;
#20586=DIRECTION ( 'NONE',  ( 1.000000000000000000, 0.000000000000000000, -1.047445008332813989E-14 ) ) ;
#20618=CARTESIAN_POINT ( 'NONE',  ( -215.9000000000000057, 53.97500000000000142, 71.43750000000000000 ) ) ;
#20633=CARTESIAN_POINT ( 'NONE',  ( 131.3179999999999836, 53.97500000000000142, 50.79999999999999716 ) ) ;
#20636=ORIENTED_EDGE ( 'NONE', *, *, #5186, .T. ) ;
#20643=ORIENTED_EDGE ( 'NONE', *, *, #59816, .T. ) ;
#20679=CARTESIAN_POINT ( 'NONE',  ( -19.89663890320305839, 44.45000000000000284, 32.49205688096009936 ) ) ;
#20688=CARTESIAN_POINT ( 'NONE',  ( -126.0120328259609863, 66.16239491992259047, 34.14452143064587375 ) ) ;
#20701=EDGE_CURVE ( 'NONE', #40497, #22712, #51016, .T. ) ;
#20711=CARTESIAN_POINT ( 'NONE',  ( 0.000000000000000000, 101.5999999999999943, 0.000000000000000000 ) ) ;
#20713=CARTESIAN_POINT ( 'NONE',  ( -4.834503460661677465, 70.80616061483986812, 130.4664586724606750 ) ) ;
#20719=DIRECTION ( 'NONE',  ( 0.000000000000000000, 1.000000000000000000, 0.000000000000000000 ) ) ;
#20722=CARTESIAN_POINT ( 'NONE',  ( -141.3509999999999991, 20.32000000000000028, -141.3509999999999991 ) ) ;
#20750=CARTESIAN_POINT ( 'NONE',  ( -187.8075999999999794, 0.000000000000000000, 114.2999999999999972 ) ) ;
#20793=CARTESIAN_POINT ( 'NONE',  ( -147.4575741623271767, 20.32000000000000028, -135.2444258376735888 ) ) ;
#20798=EDGE_CURVE ( 'NONE', #7104, #65312, #903, .T. ) ;
#20849=CARTESIAN_POINT ( 'NONE',  ( -50.03799999999999670, 101.5999999999999943, 206.3750000000000000 ) ) ;
#20866=EDGE_CURVE ( 'NONE', #46484, #13532, #84495, .T. ) ;
#20887=DIRECTION ( 'NONE',  ( 0.000000000000000000, -1.000000000000000000, 0.000000000000000000 ) ) ;
#20899=CARTESIAN_POINT ( 'NONE',  ( 4.935589585849590399, 70.84825094496120812, 130.4626753348074999 ) ) ;
#20907=CARTESIAN_POINT ( 'NONE',  ( 121.4441796687513744, 45.58144993709862547, -47.92108811332148832 ) ) ;
#20916=CARTESIAN_POINT ( 'NONE',  ( 0.000000000000000000, 44.45000000000000284, 130.5560000000000116 ) ) ;
#20923=DIRECTION ( 'NONE',  ( 0.000000000000000000, -1.000000000000000000, 0.000000000000000000 ) ) ;
#20927=ORIENTED_EDGE ( 'NONE', *, *, #51395, .F. ) ;
#20945=EDGE_CURVE ( 'NONE', #20334, #56957, #48355, .T. ) ;
#20957=CARTESIAN_POINT ( 'NONE',  ( -194.1576000000000022, 0.000000000000000000, 146.9389999999999930 ) ) ;
#20971=EDGE_CURVE ( 'NONE', #35428, #23949, #39258, .T. ) ;
#21005=DIRECTION ( 'NONE',  ( 0.000000000000000000, -1.000000000000000000, 0.000000000000000000 ) ) ;
#21031=VERTEX_POINT ( 'NONE', #14327 ) ;
#21042=EDGE_CURVE ( 'NONE', #46235, #10839, #76942, .T. ) ;
#21107=DIRECTION ( 'NONE',  ( 0.000000000000000000, -1.000000000000000000, 0.000000000000000000 ) ) ;
#21138=VECTOR ( 'NONE', #52170, 1000.000000000000000 ) ;
#21139=CARTESIAN_POINT ( 'NONE',  ( -120.0114297908194203, 74.60389011813707327, 51.40169094214619605 ) ) ;
#21141=EDGE_LOOP ( 'NONE', ( #37884, #6611, #89541, #30408 ) ) ;
#21166=CARTESIAN_POINT ( 'NONE',  ( -8.235690233012341821, 72.87934159340741758, 130.2959689530747767 ) ) ;
#21174=DIRECTION ( 'NONE',  ( 0.000000000000000000, -1.000000000000000000, 0.000000000000000000 ) ) ;
#21205=ADVANCED_FACE ( 'NONE', ( #74203 ), #67825, .F. ) ;
#21300=FACE_OUTER_BOUND ( 'NONE', #61229, .T. ) ;
#21347=CARTESIAN_POINT ( 'NONE',  ( 4.902965529469843986, 70.83457992324913732, 130.4639032678012995 ) ) ;
#21412=ADVANCED_FACE ( 'NONE', ( #75548 ), #68725, .F. ) ;
#21425=LINE ( 'NONE', #78648, #62182 ) ;
#21452=DIRECTION ( 'NONE',  ( 0.000000000000000000, 1.000000000000000000, 0.000000000000000000 ) ) ;
#21511=CARTESIAN_POINT ( 'NONE',  ( -186.2398777604655038, 101.5999999999999943, 114.2999999999999972 ) ) ;
#21536=ORIENTED_EDGE ( 'NONE', *, *, #27567, .F. ) ;
#21595=CARTESIAN_POINT ( 'NONE',  ( -112.6202530838359479, 67.89471438008003190, 66.04292222482025920 ) ) ;
#21599=ORIENTED_EDGE ( 'NONE', *, *, #63956, .F. ) ;
#21617=ORIENTED_EDGE ( 'NONE', *, *, #79360, .T. ) ;
#21631=CARTESIAN_POINT ( 'NONE',  ( 0.000000000000000000, 2.269999999999994245, 0.000000000000000000 ) ) ;
#21632=ADVANCED_FACE ( 'NONE', ( #39115 ), #80468, .F. ) ;
#21638=AXIS2_PLACEMENT_3D ( 'NONE', #12846, #19202, #46431 ) ;
#21655=ORIENTED_EDGE ( 'NONE', *, *, #83654, .F. ) ;
#21656=VERTEX_POINT ( 'NONE', #25488 ) ;
#21659=VERTEX_POINT ( 'NONE', #46356 ) ;
#21675=DIRECTION ( 'NONE',  ( -1.000000000000000000, 0.000000000000000000, -2.108231265501709878E-16 ) ) ;
#21690=ORIENTED_EDGE ( 'NONE', *, *, #66596, .T. ) ;
#21691=ORIENTED_EDGE ( 'NONE', *, *, #15756, .T. ) ;
#21718=DIRECTION ( 'NONE',  ( 4.811757763307910244E-15, 0.000000000000000000, -1.000000000000000000 ) ) ;
#21726=CARTESIAN_POINT ( 'NONE',  ( 16.74114328162335141, 66.32651888666420348, 34.24720710913430821 ) ) ;
#21743=CARTESIAN_POINT ( 'NONE',  ( 0.000000000000000000, -71.84204896855320044, 0.000000000000000000 ) ) ;
#21770=VERTEX_POINT ( 'NONE', #20483 ) ;
#21782=CARTESIAN_POINT ( 'NONE',  ( 208.9149999999999920, 43.68799999999999528, 57.14999999999999858 ) ) ;
#21790=LINE ( 'NONE', #49458, #23304 ) ;
#21803=DIRECTION ( 'NONE',  ( -1.000000000000000000, 0.000000000000000000, 1.047445008332813989E-14 ) ) ;
#21805=CARTESIAN_POINT ( 'NONE',  ( -160.2664750769294812, 101.5999999999999943, -148.0533267522755807 ) ) ;
#21807=CARTESIAN_POINT ( 'NONE',  ( 170.2205283966864897, 20.32000000000000028, -79.24800000000000466 ) ) ;
#21816=CARTESIAN_POINT ( 'NONE',  ( 124.8806136228746482, 48.00086824241649452, -38.07526654068476546 ) ) ;
#21822=DIRECTION ( 'NONE',  ( 0.000000000000000000, 1.000000000000000000, 0.000000000000000000 ) ) ;
#21839=FACE_OUTER_BOUND ( 'NONE', #27528, .T. ) ;
#21901=EDGE_CURVE ( 'NONE', #5232, #1162, #14569, .T. ) ;
#21904=DIRECTION ( 'NONE',  ( 1.000000000000000000, 0.000000000000000000, 0.000000000000000000 ) ) ;
#21931=EDGE_CURVE ( 'NONE', #37741, #6343, #76629, .T. ) ;
#21936=VERTEX_POINT ( 'NONE', #78147 ) ;
#21951=CARTESIAN_POINT ( 'NONE',  ( 127.5252020268926003, 20.32000000000000028, 177.0380000000000109 ) ) ;
#22006=EDGE_LOOP ( 'NONE', ( #63708, #40111 ) ) ;
#22012=CYLINDRICAL_SURFACE ( 'NONE', #79600, 20.63750000000000284 ) ;
#22050=CARTESIAN_POINT ( 'NONE',  ( 183.5150000000000148, 53.21300000000000097, 41.63456447661469895 ) ) ;
#22052=CARTESIAN_POINT ( 'NONE',  ( -121.1982028425885858, 74.49303996718552412, 48.53946104397632411 ) ) ;
#22069=ORIENTED_EDGE ( 'NONE', *, *, #87865, .F. ) ;
#22098=CARTESIAN_POINT ( 'NONE',  ( 0.000000000000000000, 1.270000000000000018, 0.000000000000000000 ) ) ;
#22158=ORIENTED_EDGE ( 'NONE', *, *, #34080, .T. ) ;
#22160=DIRECTION ( 'NONE',  ( 0.000000000000000000, -1.000000000000000000, 0.000000000000000000 ) ) ;
#22164=CARTESIAN_POINT ( 'NONE',  ( 160.2664750769284865, 20.32000000000000028, -148.0533267522753818 ) ) ;
#22174=ORIENTED_EDGE ( 'NONE', *, *, #34695, .F. ) ;
#22176=CYLINDRICAL_SURFACE ( 'NONE', #88167, 34.13125000000000142 ) ;
#22220=EDGE_CURVE ( 'NONE', #378, #7095, #57811, .T. ) ;
#22240=ADVANCED_FACE ( 'NONE', ( #66254 ), #4048, .F. ) ;
#22243=CYLINDRICAL_SURFACE ( 'NONE', #20419, 38.10000000000000142 ) ;
#22274=DIRECTION ( 'NONE',  ( -7.340987889507870014E-14, 0.000000000000000000, -1.000000000000000000 ) ) ;
#22276=EDGE_CURVE ( 'NONE', #6343, #38814, #55740, .T. ) ;
#22280=LINE ( 'NONE', #50409, #55601 ) ;
#22284=LINE ( 'NONE', #36354, #6943 ) ;
#22295=DIRECTION ( 'NONE',  ( 0.000000000000000000, -3.785359618865284342E-16, -1.000000000000000000 ) ) ;
#22305=LINE ( 'NONE', #34569, #52101 ) ;
#22316=DIRECTION ( 'NONE',  ( -1.000000000000000000, 0.000000000000000000, 0.000000000000000000 ) ) ;
#22367=CARTESIAN_POINT ( 'NONE',  ( -50.03799999999999670, 20.32000000000000028, 178.6098374884404905 ) ) ;
#22375=ORIENTED_EDGE ( 'NONE', *, *, #30199, .T. ) ;
#22398=EDGE_CURVE ( 'NONE', #61274, #50564, #68516, .T. ) ;
#22461=ORIENTED_EDGE ( 'NONE', *, *, #83654, .T. ) ;
#22475=ORIENTED_EDGE ( 'NONE', *, *, #6085, .T. ) ;
#22481=ORIENTED_EDGE ( 'NONE', *, *, #66840, .T. ) ;
#22483=CARTESIAN_POINT ( 'NONE',  ( -50.03799999999999670, 0.000000000000000000, 206.3750000000000000 ) ) ;
#22517=DIRECTION ( 'NONE',  ( 0.000000000000000000, -1.000000000000000000, 0.000000000000000000 ) ) ;
#22521=DIRECTION ( 'NONE',  ( 0.000000000000000000, 0.000000000000000000, -1.000000000000000000 ) ) ;
#22530=ADVANCED_FACE ( 'NONE', ( #29874 ), #65078, .T. ) ;
#22538=CARTESIAN_POINT ( 'NONE',  ( -3.175000000000109956, 8.255000000000000782, -31.75000000000000000 ) ) ;
#22599=ORIENTED_EDGE ( 'NONE', *, *, #44306, .T. ) ;
#22612=CARTESIAN_POINT ( 'NONE',  ( -215.9000000000000057, 101.5999999999999943, -45.33899999999999864 ) ) ;
#22625=CARTESIAN_POINT ( 'NONE',  ( 3.175000000000355094, 24.56180297284579694, 33.98325472291460159 ) ) ;
#22639=FACE_OUTER_BOUND ( 'NONE', #39621, .T. ) ;
#22648=CYLINDRICAL_SURFACE ( 'NONE', #43799, 9.425000000000000711 ) ;
#22654=ORIENTED_EDGE ( 'NONE', *, *, #57070, .F. ) ;
#22663=VECTOR ( 'NONE', #31490, 1000.000000000000000 ) ;
#22673=FACE_OUTER_BOUND ( 'NONE', #33573, .T. ) ;
#22681=ORIENTED_EDGE ( 'NONE', *, *, #65167, .F. ) ;
#22712=VERTEX_POINT ( 'NONE', #144 ) ;
#22713=VERTEX_POINT ( 'NONE', #75565 ) ;
#22751=CARTESIAN_POINT ( 'NONE',  ( 183.5150000000000148, 21.46300000000000097, 59.96543552338529537 ) ) ;
#22758=ORIENTED_EDGE ( 'NONE', *, *, #85346, .F. ) ;
#22763=DIRECTION ( 'NONE',  ( 0.000000000000000000, 0.000000000000000000, 1.000000000000000000 ) ) ;
#22779=EDGE_LOOP ( 'NONE', ( #8433, #64175, #79498, #45475, #60713, #21536 ) ) ;
#22845=EDGE_CURVE ( 'NONE', #66449, #45792, #70080, .T. ) ;
#22861=DIRECTION ( 'NONE',  ( 2.301579500234999682E-14, 0.000000000000000000, -1.000000000000000000 ) ) ;
#22885=ORIENTED_EDGE ( 'NONE', *, *, #44306, .F. ) ;
#22891=DIRECTION ( 'NONE',  ( 0.000000000000000000, 1.000000000000000000, 0.000000000000000000 ) ) ;
#22919=CARTESIAN_POINT ( 'NONE',  ( 131.3179999999999836, 34.75001145038165618, 43.29625283494679877 ) ) ;
#22973=CARTESIAN_POINT ( 'NONE',  ( 0.000000000000000000, 11.98343896644750117, 0.000000000000000000 ) ) ;
#23026=CARTESIAN_POINT ( 'NONE',  ( -7.158941453477376982, 93.04008847735218524, 130.3595723459966962 ) ) ;
#23068=CARTESIAN_POINT ( 'NONE',  ( -109.2774118001975836, 52.30007095126370587, 71.43750000000027001 ) ) ;
#23081=LINE ( 'NONE', #16250, #87033 ) ;
#23083=CARTESIAN_POINT ( 'NONE',  ( 21.50062301572775780, 61.16842642911653627, 31.45420966082828329 ) ) ;
#23096=ADVANCED_FACE ( 'NONE', ( #25058 ), #66837, .F. ) ;
#23106=DIRECTION ( 'NONE',  ( 0.000000000000000000, -1.000000000000000000, 0.000000000000000000 ) ) ;
#23113=VERTEX_POINT ( 'NONE', #28642 ) ;
#23134=CARTESIAN_POINT ( 'NONE',  ( 141.3509999999999991, 20.32000000000000028, 132.7150000000000034 ) ) ;
#23142=DIRECTION ( 'NONE',  ( 1.000000000000000000, 0.000000000000000000, 0.000000000000000000 ) ) ;
#23192=EDGE_CURVE ( 'NONE', #42800, #89089, #57173, .T. ) ;
#23218=CYLINDRICAL_SURFACE ( 'NONE', #27307, 34.13125000000000142 ) ;
#23223=LINE ( 'NONE', #10454, #69523 ) ;
#23238=CARTESIAN_POINT ( 'NONE',  ( -160.2664750769284865, 0.000000000000000000, 148.0533267522753818 ) ) ;
#23241=ORIENTED_EDGE ( 'NONE', *, *, #39871, .T. ) ;
#23251=ORIENTED_EDGE ( 'NONE', *, *, #84781, .T. ) ;
#23269=VERTEX_POINT ( 'NONE', #33114 ) ;
#23282=DIRECTION ( 'NONE',  ( 2.108231265501709878E-16, 0.000000000000000000, -1.000000000000000000 ) ) ;
#23304=VECTOR ( 'NONE', #42638, 1000.000000000000000 ) ;
#23312=LINE ( 'NONE', #87301, #18549 ) ;
#23327=FACE_OUTER_BOUND ( 'NONE', #73708, .T. ) ;
#23358=VECTOR ( 'NONE', #61437, 1000.000000000000000 ) ;
#23361=DIRECTION ( 'NONE',  ( 0.000000000000000000, -1.000000000000000000, 0.000000000000000000 ) ) ;
#23380=VECTOR ( 'NONE', #16712, 1000.000000000000000 ) ;
#23385=ORIENTED_EDGE ( 'NONE', *, *, #50273, .T. ) ;
#23399=VERTEX_POINT ( 'NONE', #31768 ) ;
#23401=CARTESIAN_POINT ( 'NONE',  ( -194.1576000000000022, 0.000000000000000000, -45.33899999999999864 ) ) ;
#23406=AXIS2_PLACEMENT_3D ( 'NONE', #48196, #22316, #70921 ) ;
#23441=CARTESIAN_POINT ( 'NONE',  ( -187.8075999999999794, 20.32000000000000028, -9.525000000000000355 ) ) ;
#23462=ORIENTED_EDGE ( 'NONE', *, *, #62623, .T. ) ;
#23464=VERTEX_POINT ( 'NONE', #19938 ) ;
#23476=EDGE_LOOP ( 'NONE', ( #11486, #56170, #22375, #89635, #436, #39513, #34399, #24286, #72619, #41340, #34078, #68723, #23251, #28253, #13888 ) ) ;
#23493=VECTOR ( 'NONE', #18749, 1000.000000000000000 ) ;
#23503=ORIENTED_EDGE ( 'NONE', *, *, #26301, .F. ) ;
#23535=DIRECTION ( 'NONE',  ( 1.000000000000000000, 0.000000000000000000, 2.108231265501709878E-16 ) ) ;
#23558=CIRCLE ( 'NONE', #74305, 160.4955849403809793 ) ;
#23581=DIRECTION ( 'NONE',  ( 0.000000000000000000, 0.000000000000000000, -1.000000000000000000 ) ) ;
#23587=FACE_OUTER_BOUND ( 'NONE', #83343, .T. ) ;
#23597=DIRECTION ( 'NONE',  ( 0.000000000000000000, -1.000000000000000000, 0.000000000000000000 ) ) ;
#23617=CARTESIAN_POINT ( 'NONE',  ( -55.11501535285000131, 101.5999999999999943, 183.9403141659174992 ) ) ;
#23618=LINE ( 'NONE', #63594, #53827 ) ;
#23643=ORIENTED_EDGE ( 'NONE', *, *, #31210, .T. ) ;
#23649=ORIENTED_EDGE ( 'NONE', *, *, #13451, .F. ) ;
#23704=PRESENTATION_STYLE_ASSIGNMENT (( #80007 ) ) ;
#23717=AXIS2_PLACEMENT_3D ( 'NONE', #55912, #49104, #85 ) ;
#23728=VERTEX_POINT ( 'NONE', #2186 ) ;
#23745=CIRCLE ( 'NONE', #32395, 8.636000000000004562 ) ;
#23828=CARTESIAN_POINT ( 'NONE',  ( -127.0239848601436847, 55.39831567219715680, 30.16249999999990195 ) ) ;
#23835=ORIENTED_EDGE ( 'NONE', *, *, #44132, .T. ) ;
#23860=EDGE_CURVE ( 'NONE', #46362, #13204, #81182, .T. ) ;
#23878=CARTESIAN_POINT ( 'NONE',  ( 0.000000000000000000, 152.3879256507328250, -9.425000000000000711 ) ) ;
#23879=CARTESIAN_POINT ( 'NONE',  ( 125.3463460965257070, 52.73749999999999716, -36.51249999999992468 ) ) ;
#23911=CARTESIAN_POINT ( 'NONE',  ( -7.582671002870624122, 92.73938028448795023, 130.3355715079545689 ) ) ;
#23915=CARTESIAN_POINT ( 'NONE',  ( 127.0239848601435995, 53.97500000000000142, 30.16249999999999787 ) ) ;
#23926=ORIENTED_EDGE ( 'NONE', *, *, #89710, .F. ) ;
#23941=DIRECTION ( 'NONE',  ( 0.000000000000000000, -1.000000000000000000, 0.000000000000000000 ) ) ;
#23949=VERTEX_POINT ( 'NONE', #26193 ) ;
#23952=ORIENTED_EDGE ( 'NONE', *, *, #18001, .F. ) ;
#23953=VECTOR ( 'NONE', #69582, 1000.000000000000000 ) ;
#23985=DIRECTION ( 'NONE',  ( -2.108231265501709878E-16, 0.000000000000000000, 1.000000000000000000 ) ) ;
#23986=VERTEX_POINT ( 'NONE', #13462 ) ;
#23997=CARTESIAN_POINT ( 'NONE',  ( 55.11501535284990183, 0.000000000000000000, 183.9403141659174992 ) ) ;
#23999=FACE_OUTER_BOUND ( 'NONE', #89762, .T. ) ;
#24014=ORIENTED_EDGE ( 'NONE', *, *, #80736, .T. ) ;
#24018=AXIS2_PLACEMENT_3D ( 'NONE', #72810, #30584, #58713 ) ;
#24033=VECTOR ( 'NONE', #37173, 1000.000000000000000 ) ;
#24062=ORIENTED_EDGE ( 'NONE', *, *, #63006, .T. ) ;
#24074=CARTESIAN_POINT ( 'NONE',  ( 110.4401826102544533, 62.42991204253968363, 69.62641815663941713 ) ) ;
#24157=DIRECTION ( 'NONE',  ( 0.000000000000000000, -1.000000000000000000, 0.000000000000000000 ) ) ;
#24177=EDGE_CURVE ( 'NONE', #38814, #33479, #56575, .T. ) ;
#24191=CARTESIAN_POINT ( 'NONE',  ( 131.3179999999999836, 53.97500000000000142, 30.16249999999999787 ) ) ;
#24213=ORIENTED_EDGE ( 'NONE', *, *, #32645, .F. ) ;
#24225=VECTOR ( 'NONE', #72756, 1000.000000000000114 ) ;
#24237=DIRECTION ( 'NONE',  ( -0.7071067811865739960, 0.000000000000000000, -0.7071067811865210384 ) ) ;
#24239=CARTESIAN_POINT ( 'NONE',  ( 173.9900000000000091, 101.5999999999999943, 131.6533725204182019 ) ) ;
#24242=ORIENTED_EDGE ( 'NONE', *, *, #24177, .T. ) ;
#24259=DIRECTION ( 'NONE',  ( 0.000000000000000000, 1.000000000000000000, 0.000000000000000000 ) ) ;
#24286=ORIENTED_EDGE ( 'NONE', *, *, #56022, .T. ) ;
#24314=FACE_OUTER_BOUND ( 'NONE', #72331, .T. ) ;
#24348=CARTESIAN_POINT ( 'NONE',  ( -10.58606582829696308, 89.56609333295101294, 130.1261100651620950 ) ) ;
#24354=CARTESIAN_POINT ( 'NONE',  ( 126.7387501644084722, 47.09211651945648924, 31.33975947824927388 ) ) ;
#24372=AXIS2_PLACEMENT_3D ( 'NONE', #60526, #60990, #88274 ) ;
#24388=CARTESIAN_POINT ( 'NONE',  ( -179.8898777604659927, 101.5999999999999943, -123.4696824136383952 ) ) ;
#24390=PLANE ( 'NONE',  #46547 ) ;
#24397=VERTEX_POINT ( 'NONE', #47848 ) ;
#24401=ORIENTED_EDGE ( 'NONE', *, *, #46424, .F. ) ;
#24404=CARTESIAN_POINT ( 'NONE',  ( 131.3179999999999836, 53.97500000000000142, 50.79999999999999716 ) ) ;
#24428=DIRECTION ( 'NONE',  ( -0.000000000000000000, 1.000000000000000000, 0.000000000000000000 ) ) ;
#24444=AXIS2_PLACEMENT_3D ( 'NONE', #60160, #25209, #39291 ) ;
#24454=DIRECTION ( 'NONE',  ( 1.000000000000000000, 0.000000000000000000, 0.000000000000000000 ) ) ;
#24470=CARTESIAN_POINT ( 'NONE',  ( 120.9217020216711234, 59.09882332812808414, -49.22416681939083816 ) ) ;
#24493=DIRECTION ( 'NONE',  ( 0.000000000000000000, 0.000000000000000000, 1.000000000000000000 ) ) ;
#24508=CARTESIAN_POINT ( 'NONE',  ( 0.000000000000000000, 1.270000000000000018, 0.000000000000000000 ) ) ;
#24513=CARTESIAN_POINT ( 'NONE',  ( 114.9214557239245096, 71.34069570408355787, 61.95106117944241930 ) ) ;
#24525=DIRECTION ( 'NONE',  ( 0.000000000000000000, -1.000000000000000000, 0.000000000000000000 ) ) ;
#24531=VECTOR ( 'NONE', #32272, 1000.000000000000000 ) ;
#24562=ORIENTED_EDGE ( 'NONE', *, *, #74411, .F. ) ;
#24581=DIRECTION ( 'NONE',  ( 0.000000000000000000, 0.000000000000000000, -1.000000000000000000 ) ) ;
#24595=EDGE_CURVE ( 'NONE', #5363, #4177, #84648, .T. ) ;
#24599=PLANE ( 'NONE',  #16048 ) ;
#24601=AXIS2_PLACEMENT_3D ( 'NONE', #85842, #3156, #17233 ) ;
#24605=CYLINDRICAL_SURFACE ( 'NONE', #80770, 9.525000000000000355 ) ;
#24627=LINE ( 'NONE', #24191, #57267 ) ;
#24661=LINE ( 'NONE', #67324, #70372 ) ;
#24676=CARTESIAN_POINT ( 'NONE',  ( -141.3509999999999991, 0.000000000000000000, 141.3509999999999991 ) ) ;
#24681=ADVANCED_FACE ( 'NONE', ( #69659 ), #77824, .T. ) ;
#24697=DIRECTION ( 'NONE',  ( 0.000000000000000000, -1.000000000000000000, 0.000000000000000000 ) ) ;
#24703=LINE ( 'NONE', #80130, #85565 ) ;
#24707=DIRECTION ( 'NONE',  ( 1.000000000000000000, 0.000000000000000000, 0.000000000000000000 ) ) ;
#24711=CARTESIAN_POINT ( 'NONE',  ( 0.000000000000000000, 95.00619999999999266, -9.525000000000000355 ) ) ;
#24740=DIRECTION ( 'NONE',  ( 0.000000000000000000, -1.000000000000000000, 0.000000000000000000 ) ) ;
#24766=CARTESIAN_POINT ( 'NONE',  ( 208.9149999999999920, 37.33800000000000097, 50.79999999999999716 ) ) ;
#24788=CARTESIAN_POINT ( 'NONE',  ( -3.230781895526043890, 94.86034579432060809, 130.5182095844837704 ) ) ;
#24830=PLANE ( 'NONE',  #17717 ) ;
#24836=VECTOR ( 'NONE', #12577, 1000.000000000000000 ) ;
#24866=DIRECTION ( 'NONE',  ( -1.000000000000000000, 0.000000000000000000, 3.491483361109380094E-15 ) ) ;
#24869=ORIENTED_EDGE ( 'NONE', *, *, #28654, .T. ) ;
#24897=VECTOR ( 'NONE', #51243, 1000.000000000000000 ) ;
#24903=DIRECTION ( 'NONE',  ( 0.000000000000000000, -1.000000000000000000, 0.000000000000000000 ) ) ;
#24912=CARTESIAN_POINT ( 'NONE',  ( 125.0187123012608481, 56.81681257766939552, -37.62034114384582750 ) ) ;
#24917=CARTESIAN_POINT ( 'NONE',  ( 183.5150000000000148, 37.33800000000000097, 50.79999999999999716 ) ) ;
#24938=ORIENTED_EDGE ( 'NONE', *, *, #51395, .T. ) ;
#24947=DIRECTION ( 'NONE',  ( 0.000000000000000000, -1.000000000000000000, 0.000000000000000000 ) ) ;
#24953=CARTESIAN_POINT ( 'NONE',  ( 111.9933789837352833, 66.64000986900705925, 67.10026523892989303 ) ) ;
#24978=VECTOR ( 'NONE', #17481, 1000.000000000000000 ) ;
#24982=CARTESIAN_POINT ( 'NONE',  ( 170.2205283966864897, 101.5999999999999943, 79.24800000000000466 ) ) ;
#25024=CARTESIAN_POINT ( 'NONE',  ( 0.000000000000000000, 152.3879256507328250, 0.000000000000000000 ) ) ;
#25027=CARTESIAN_POINT ( 'NONE',  ( -158.9822249764575020, 20.32000000000000028, 139.6999999999999886 ) ) ;
#25033=ORIENTED_EDGE ( 'NONE', *, *, #80061, .T. ) ;
#25048=DIRECTION ( 'NONE',  ( 0.000000000000000000, 0.000000000000000000, -1.000000000000000000 ) ) ;
#25058=FACE_OUTER_BOUND ( 'NONE', #33938, .T. ) ;
#25094=CARTESIAN_POINT ( 'NONE',  ( 10.33715916136909563, 89.92838495571164970, 130.1461902906857802 ) ) ;
#25112=VECTOR ( 'NONE', #73120, 1000.000000000000000 ) ;
#25122=ORIENTED_EDGE ( 'NONE', *, *, #39119, .F. ) ;
#25141=ORIENTED_EDGE ( 'NONE', *, *, #19256, .F. ) ;
#25169=CARTESIAN_POINT ( 'NONE',  ( -16.71522554099469815, 66.30250908626825890, 34.24257953154918965 ) ) ;
#25209=DIRECTION ( 'NONE',  ( -1.000000000000000000, 0.000000000000000000, 0.000000000000000000 ) ) ;
#25230=CARTESIAN_POINT ( 'NONE',  ( 126.9292520036857894, 49.86282737081235439, 30.55937423833577071 ) ) ;
#25242=ORIENTED_EDGE ( 'NONE', *, *, #80592, .T. ) ;
#25243=DIRECTION ( 'NONE',  ( 0.000000000000000000, 0.000000000000000000, -1.000000000000000000 ) ) ;
#25274=ORIENTED_EDGE ( 'NONE', *, *, #89065, .T. ) ;
#25278=DIRECTION ( 'NONE',  ( -0.000000000000000000, 1.000000000000000000, 0.000000000000000000 ) ) ;
#25286=CARTESIAN_POINT ( 'NONE',  ( 71.09939861440099662, 0.000000000000000000, 177.8662485265279827 ) ) ;
#25339=CARTESIAN_POINT ( 'NONE',  ( 148.0533267522752112, 101.5999999999999943, 160.2664750769284865 ) ) ;
#25343=CARTESIAN_POINT ( 'NONE',  ( 125.0952692105185804, 56.35416992947224912, -37.36429652679031221 ) ) ;
#25367=VECTOR ( 'NONE', #44321, 1000.000000000000000 ) ;
#25368=EDGE_CURVE ( 'NONE', #13204, #64268, #70094, .T. ) ;
#25394=CARTESIAN_POINT ( 'NONE',  ( 112.8147779832228963, 68.25761352872008558, 65.71143442840111959 ) ) ;
#25426=EDGE_CURVE ( 'NONE', #38579, #88991, #13498, .T. ) ;
#25431=CIRCLE ( 'NONE', #71876, 12.69999999999999929 ) ;
#25449=EDGE_CURVE ( 'NONE', #45185, #12149, #6501, .T. ) ;
#25466=CARTESIAN_POINT ( 'NONE',  ( 131.3179999999999836, 53.97500000000000142, 50.79999999999999716 ) ) ;
#25468=VECTOR ( 'NONE', #9100, 1000.000000000000000 ) ;
#25488=CARTESIAN_POINT ( 'NONE',  ( 163.0822201311030142, 20.32000000000000028, 75.92468371870748456 ) ) ;
#25493=LINE ( 'NONE', #45911, #24225 ) ;
#25533=CARTESIAN_POINT ( 'NONE',  ( 0.000000000000000000, 1.270000000000000018, -9.525000000000000355 ) ) ;
#25537=CARTESIAN_POINT ( 'NONE',  ( 9.368522474371046016, 91.14223545714233410, 130.2200199954151856 ) ) ;
#25538=VERTEX_POINT ( 'NONE', #78708 ) ;
#25545=CARTESIAN_POINT ( 'NONE',  ( -185.9961463128564958, 101.5999999999999943, -3.174999999999349676 ) ) ;
#25554=AXIS2_PLACEMENT_3D ( 'NONE', #59185, #30609, #10600 ) ;
#25560=CARTESIAN_POINT ( 'NONE',  ( 1.598849875094819542E-14, 101.5999999999999943, -130.5560000000000116 ) ) ;
#25570=LINE ( 'NONE', #82803, #89506 ) ;
#25574=CIRCLE ( 'NONE', #63320, 7.873999999999991672 ) ;
#25614=AXIS2_PLACEMENT_3D ( 'NONE', #58197, #51362, #44547 ) ;
#25618=VERTEX_POINT ( 'NONE', #70988 ) ;
#25647=CLOSED_SHELL ( 'NONE', ( #83457, #68665, #52093, #44530, #85605, #32245, #409, #8619, #29620, #87279, #59302, #8398, #79614, #42162, #56510, #40564, #46499, #31121, #7553, #79243, #54276, #77534, #31515, #46271, #39161, #50183, #44450, #22530, #54886, #42390, #43831, #87678, #11552, #86133, #44573, #21412, #85155, #72637, #86398, #82595, #11999, #48899, #52028, #73148, #65476, #50903, #57362, #48513, #88574, #47849, #28943, #53858, #79866, #19277, #45406, #36879, #78568, #42945, #3923, #4360, #32638, #68874, #52692, #63643, #31358, #17659, #2965, #59538, #39004, #49875, #11724, #26532, #6246, #88875, #38482, #24681, #22240, #7306, #23096, #9917, #58601, #55693, #54884, #45083, #4340, #81295, #11703, #38694, #21632, #78645, #28205, #19672, #40446, #66732, #59836, #8612, #81274, #73070, #14657, #89109, #5514, #32548, #53118, #86962, #32116, #64263, #5176, #76863, #40236, #49656, #8043, #4875, #78684, #81803, #80012, #57175, #63102, #73430, #69270, #41572, #20313, #30515, #76573, #12587, #61572, #44339, #67976, #36266, #21205, #49141, #12514, #75431, #75652, #75731, #57409, #56845, #8905, #16968, #19428, #14402, #73575, #16061 ) ) ;
#25691=ORIENTED_EDGE ( 'NONE', *, *, #20271, .T. ) ;
#25694=CARTESIAN_POINT ( 'NONE',  ( 173.9900000000000091, 37.33800000000000097, 50.79999999999999716 ) ) ;
#25704=VERTEX_POINT ( 'NONE', #65496 ) ;
#25723=CARTESIAN_POINT ( 'NONE',  ( 0.000000000000000000, 152.3879256507328250, -9.425000000000000711 ) ) ;
#25817=ORIENTED_EDGE ( 'NONE', *, *, #25449, .T. ) ;
#25831=DIRECTION ( 'NONE',  ( 0.000000000000000000, 1.000000000000000000, 0.000000000000000000 ) ) ;
#25868=PRODUCT_CONTEXT ( 'NONE', #37076, 'mechanical' ) ;
#25870=CARTESIAN_POINT ( 'NONE',  ( 0.000000000000000000, 12.27000000000000313, 0.000000000000000000 ) ) ;
#25877=AXIS2_PLACEMENT_3D ( 'NONE', #22973, #36597, #42478 ) ;
#25884=EDGE_CURVE ( 'NONE', #66001, #26221, #6397, .T. ) ;
#25894=LINE ( 'NONE', #78440, #25367 ) ;
#25972=ORIENTED_EDGE ( 'NONE', *, *, #19121, .F. ) ;
#25992=DIRECTION ( 'NONE',  ( -1.000000000000000000, 0.000000000000000000, 0.000000000000000000 ) ) ;
#25993=ORIENTED_EDGE ( 'NONE', *, *, #25884, .F. ) ;
#26002=DIRECTION ( 'NONE',  ( 0.000000000000000000, 1.000000000000000000, 0.000000000000000000 ) ) ;
#26030=DIRECTION ( 'NONE',  ( 0.000000000000000000, -1.000000000000000000, 0.000000000000000000 ) ) ;
#26034=LINE ( 'NONE', #60527, #62751 ) ;
#26078=CARTESIAN_POINT ( 'NONE',  ( -21.00265438680891705, 62.01110210563430769, 31.78899330339352858 ) ) ;
#26083=DIRECTION ( 'NONE',  ( 1.000000000000000000, 0.000000000000000000, -4.277118011829300531E-15 ) ) ;
#26085=CARTESIAN_POINT ( 'NONE',  ( 160.2664750769289697, 101.5999999999999943, 148.0533267522752112 ) ) ;
#26089=CARTESIAN_POINT ( 'NONE',  ( 183.5150000000000148, 37.33800000000000097, 60.32499999999999574 ) ) ;
#26090=PLANE ( 'NONE',  #7169 ) ;
#26109=CARTESIAN_POINT ( 'NONE',  ( 22.68560957326527472, 49.60990628430907634, 30.61209429277630534 ) ) ;
#26112=EDGE_CURVE ( 'NONE', #77555, #43158, #22280, .T. ) ;
#26177=AXIS2_PLACEMENT_3D ( 'NONE', #77648, #29948, #36758 ) ;
#26183=CARTESIAN_POINT ( 'NONE',  ( -12.06903998855693061, 78.50064190147526233, 129.9973879043436398 ) ) ;
#26187=DIRECTION ( 'NONE',  ( 0.000000000000000000, 0.000000000000000000, 1.000000000000000000 ) ) ;
#26193=CARTESIAN_POINT ( 'NONE',  ( 0.000000000000000000, 125.7300000000000040, -9.425000000000000711 ) ) ;
#26221=VERTEX_POINT ( 'NONE', #67164 ) ;
#26227=AXIS2_PLACEMENT_3D ( 'NONE', #34192, #20586, #61895 ) ;
#26247=CARTESIAN_POINT ( 'NONE',  ( 121.5330498715421896, 59.98657059693208282, -47.69329234032820608 ) ) ;
#26265=EDGE_CURVE ( 'NONE', #65449, #55364, #42575, .T. ) ;
#26286=LINE ( 'NONE', #84413, #60037 ) ;
#26301=EDGE_CURVE ( 'NONE', #65247, #78334, #58557, .T. ) ;
#26316=PLANE ( 'NONE',  #2092 ) ;
#26324=CIRCLE ( 'NONE', #64003, 12.69999999999998863 ) ;
#26355=DIRECTION ( 'NONE',  ( -1.000000000000000000, 0.000000000000000000, 0.000000000000000000 ) ) ;
#26365=CARTESIAN_POINT ( 'NONE',  ( 0.000000000000000000, 95.00619999999999266, 0.000000000000000000 ) ) ;
#26366=LINE ( 'NONE', #54035, #24531 ) ;
#26369=CARTESIAN_POINT ( 'NONE',  ( -75.61066417432020614, 101.5999999999999943, 189.7379999999999995 ) ) ;
#26402=AXIS2_PLACEMENT_3D ( 'NONE', #34443, #62152, #35784 ) ;
#26414=EDGE_LOOP ( 'NONE', ( #37221, #35047, #42547, #49840 ) ) ;
#26415=LINE ( 'NONE', #14587, #87101 ) ;
#26425=CARTESIAN_POINT ( 'NONE',  ( 208.9149999999999920, 37.33800000000000097, 50.79999999999999716 ) ) ;
#26429=EDGE_CURVE ( 'NONE', #21656, #88388, #36265, .T. ) ;
#26442=CARTESIAN_POINT ( 'NONE',  ( 12.69999999999999751, 83.33714971666560700, 129.9368274816649773 ) ) ;
#26461=DIRECTION ( 'NONE',  ( 0.000000000000000000, 0.000000000000000000, 1.000000000000000000 ) ) ;
#26526=EDGE_CURVE ( 'NONE', #36938, #13582, #23081, .T. ) ;
#26532=ADVANCED_FACE ( 'NONE', ( #63488 ), #7192, .F. ) ;
#26580=AXIS2_PLACEMENT_3D ( 'NONE', #44495, #4065, #72227 ) ;
#26586=ORIENTED_EDGE ( 'NONE', *, *, #19670, .T. ) ;
#26590=ORIENTED_EDGE ( 'NONE', *, *, #43224, .T. ) ;
#26594=CARTESIAN_POINT ( 'NONE',  ( -109.2774118001975836, 54.68092463569039552, 71.43750000000027001 ) ) ;
#26624=CARTESIAN_POINT ( 'NONE',  ( -12.31154164839621146, 79.32405795620842071, 129.9746777458391591 ) ) ;
#26647=CARTESIAN_POINT ( 'NONE',  ( 0.000000000000000000, 1.270000000000000018, -9.425000000000000711 ) ) ;
#26674=DIRECTION ( 'NONE',  ( 1.000000000000000000, 0.000000000000000000, 0.000000000000000000 ) ) ;
#26703=DIRECTION ( 'NONE',  ( 0.000000000000000000, -1.000000000000000000, 0.000000000000000000 ) ) ;
#26717=AXIS2_PLACEMENT_3D ( 'NONE', #30721, #71181, #39645 ) ;
#26732=VERTEX_POINT ( 'NONE', #54297 ) ;
#26753=ORIENTED_EDGE ( 'NONE', *, *, #12569, .T. ) ;
#26782=CIRCLE ( 'NONE', #61606, 31.75000000000000000 ) ;
#26786=CIRCLE ( 'NONE', #61608, 8.636000000000004562 ) ;
#26793=LINE ( 'NONE', #28583, #29039 ) ;
#26824=DIRECTION ( 'NONE',  ( 0.000000000000000000, -1.000000000000000000, 0.000000000000000000 ) ) ;
#26834=DIRECTION ( 'NONE',  ( 0.000000000000000000, -1.000000000000000000, 0.000000000000000000 ) ) ;
#26838=DIRECTION ( 'NONE',  ( 0.000000000000000000, 0.000000000000000000, -1.000000000000000000 ) ) ;
#26849=CARTESIAN_POINT ( 'NONE',  ( 173.9900000000000091, 21.46300000000000097, 59.96543552338529537 ) ) ;
#26884=CARTESIAN_POINT ( 'NONE',  ( 10.45076961392105908, 89.76615655770415003, 130.1370655302031025 ) ) ;
#26924=ORIENTED_EDGE ( 'NONE', *, *, #62520, .T. ) ;
#26978=CARTESIAN_POINT ( 'NONE',  ( 75.61066417432020614, 0.000000000000000000, 177.0380000000000109 ) ) ;
#26997=VECTOR ( 'NONE', #40082, 1000.000000000000000 ) ;
#27011=VECTOR ( 'NONE', #76628, 1000.000000000000000 ) ;
#27023=EDGE_CURVE ( 'NONE', #1162, #51892, #53178, .T. ) ;
#27053=CARTESIAN_POINT ( 'NONE',  ( -114.6380061954168923, 70.99355617351733372, 62.47401523881796948 ) ) ;
#27080=CARTESIAN_POINT ( 'NONE',  ( -7.291605166176498010, 72.14803965971481148, 130.3524295837840725 ) ) ;
#27083=CARTESIAN_POINT ( 'NONE',  ( 33.98325472291465132, 8.255000000000000782, 3.174999999999999822 ) ) ;
#27093=EDGE_CURVE ( 'NONE', #18383, #23728, #82294, .T. ) ;
#27116=DIRECTION ( 'NONE',  ( 0.000000000000000000, -1.000000000000000000, 0.000000000000000000 ) ) ;
#27130=EDGE_CURVE ( 'NONE', #2756, #28030, #26415, .T. ) ;
#27134=ORIENTED_EDGE ( 'NONE', *, *, #29119, .F. ) ;
#27154=DIRECTION ( 'NONE',  ( 0.000000000000000000, -1.000000000000000000, 0.000000000000000000 ) ) ;
#27159=CARTESIAN_POINT ( 'NONE',  ( 173.9900000000000091, 20.32000000000000028, 71.37400000000000944 ) ) ;
#27185=DIRECTION ( 'NONE',  ( -1.047445008332813989E-14, 0.000000000000000000, -1.000000000000000000 ) ) ;
#27197=ORIENTED_EDGE ( 'NONE', *, *, #64870, .F. ) ;
#27226=DIRECTION ( 'NONE',  ( 1.000000000000000000, 0.000000000000000000, 0.000000000000000000 ) ) ;
#27262=CYLINDRICAL_SURFACE ( 'NONE', #3583, 12.69999999999998863 ) ;
#27305=DIRECTION ( 'NONE',  ( 0.000000000000000000, -1.000000000000000000, 0.000000000000000000 ) ) ;
#27307=AXIS2_PLACEMENT_3D ( 'NONE', #51758, #38585, #9120 ) ;
#27343=AXIS2_PLACEMENT_3D ( 'NONE', #25466, #11847, #39541 ) ;
#27345=ORIENTED_EDGE ( 'NONE', *, *, #62623, .F. ) ;
#27348=FACE_OUTER_BOUND ( 'NONE', #34104, .T. ) ;
#27362=VECTOR ( 'NONE', #22517, 1000.000000000000000 ) ;
#27376=CARTESIAN_POINT ( 'NONE',  ( 208.9149999999999920, 30.98800000000000310, 44.45000000000000284 ) ) ;
#27399=AXIS2_PLACEMENT_3D ( 'NONE', #74154, #39178, #11930 ) ;
#27435=EDGE_CURVE ( 'NONE', #18059, #51056, #47898, .T. ) ;
#27448=DIRECTION ( 'NONE',  ( 1.000000000000000000, 0.000000000000000000, 2.108231265501709878E-16 ) ) ;
#27465=DIRECTION ( 'NONE',  ( 0.000000000000000000, 0.000000000000000000, 1.000000000000000000 ) ) ;
#27474=EDGE_CURVE ( 'NONE', #52538, #21031, #86308, .T. ) ;
#27475=DIRECTION ( 'NONE',  ( -0.000000000000000000, 1.000000000000000000, -0.000000000000000000 ) ) ;
#27486=DIRECTION ( 'NONE',  ( 2.761895400282000234E-15, 0.000000000000000000, 1.000000000000000000 ) ) ;
#27491=CARTESIAN_POINT ( 'NONE',  ( -119.8041702335904546, 74.58518942925769579, 51.88336617615348700 ) ) ;
#27511=EDGE_LOOP ( 'NONE', ( #46612, #6746, #1662, #84747 ) ) ;
#27514=DIRECTION ( 'NONE',  ( 1.000000000000000000, 0.000000000000000000, -3.491483361109380094E-15 ) ) ;
#27519=CARTESIAN_POINT ( 'NONE',  ( -6.892982596720425015, 71.88311738247121241, 130.3739197406787582 ) ) ;
#27528=EDGE_LOOP ( 'NONE', ( #22681, #32052, #80260, #87141 ) ) ;
#27560=EDGE_CURVE ( 'NONE', #23949, #35428, #77056, .T. ) ;
#27567=EDGE_CURVE ( 'NONE', #38934, #57278, #86756, .T. ) ;
#27585=EDGE_CURVE ( 'NONE', #7937, #10881, #75551, .T. ) ;
#27630=EDGE_CURVE ( 'NONE', #5834, #55364, #82641, .T. ) ;
#27634=CARTESIAN_POINT ( 'NONE',  ( -31.75000000000000000, 8.255000000000000782, -3.174999999999779998 ) ) ;
#27661=ORIENTED_EDGE ( 'NONE', *, *, #969, .T. ) ;
#27670=DIRECTION ( 'NONE',  ( -1.224646799147355426E-16, 0.000000000000000000, -1.000000000000000000 ) ) ;
#27680=VECTOR ( 'NONE', #63786, 1000.000000000000000 ) ;
#27696=CARTESIAN_POINT ( 'NONE',  ( -57.91199999999999903, 101.5999999999999943, 191.3008000794699797 ) ) ;
#27706=DIRECTION ( 'NONE',  ( 0.000000000000000000, 0.000000000000000000, 1.000000000000000000 ) ) ;
#27707=DIRECTION ( 'NONE',  ( 0.000000000000000000, -1.000000000000000000, 0.000000000000000000 ) ) ;
#27709=CARTESIAN_POINT ( 'NONE',  ( 7.373078322898753534, 72.20904964896763545, 130.3475976157996570 ) ) ;
#27717=CARTESIAN_POINT ( 'NONE',  ( 122.8247853069674136, 44.79825420117990120, -44.26074039117278147 ) ) ;
#27743=DIRECTION ( 'NONE',  ( 0.000000000000000000, 0.000000000000000000, -1.000000000000000000 ) ) ;
#27770=ORIENTED_EDGE ( 'NONE', *, *, #88763, .T. ) ;
#27774=FACE_OUTER_BOUND ( 'NONE', #86592, .T. ) ;
#27782=PLANE ( 'NONE',  #16442 ) ;
#27791=VERTEX_POINT ( 'NONE', #89896 ) ;
#27801=CARTESIAN_POINT ( 'NONE',  ( 50.03799999999999670, 101.5999999999999943, 206.3750000000000000 ) ) ;
#27807=VECTOR ( 'NONE', #11263, 999.9999999999998863 ) ;
#27829=EDGE_LOOP ( 'NONE', ( #79370, #51516, #55460, #32755 ) ) ;
#27836=CARTESIAN_POINT ( 'NONE',  ( -185.9961463128564958, 101.5999999999999943, -9.525000000000000355 ) ) ;
#27905=CARTESIAN_POINT ( 'NONE',  ( 131.3179999999999836, 53.97500000000000142, 50.79999999999999716 ) ) ;
#27921=AXIS2_PLACEMENT_3D ( 'NONE', #10280, #86594, #3911 ) ;
#27938=CARTESIAN_POINT ( 'NONE',  ( -114.7114918133012793, 71.08538102460907737, 62.33898210981162435 ) ) ;
#27944=EDGE_LOOP ( 'NONE', ( #30026, #48253, #22654, #55762, #18926, #49708, #81144, #31688, #50839, #78482, #15298, #639, #58394, #88238, #68552, #68838 ) ) ;
#27963=CARTESIAN_POINT ( 'NONE',  ( -11.70177394069033383, 77.61446958840116395, 130.0305271391580675 ) ) ;
#27973=EDGE_CURVE ( 'NONE', #18422, #18383, #15821, .T. ) ;
#27982=DIRECTION ( 'NONE',  ( 0.000000000000000000, -1.000000000000000000, 0.000000000000000000 ) ) ;
#28005=ORIENTED_EDGE ( 'NONE', *, *, #31210, .F. ) ;
#28014=CARTESIAN_POINT ( 'NONE',  ( 183.5150000000000148, 37.33800000000000097, 69.13087104677069306 ) ) ;
#28021=DIRECTION ( 'NONE',  ( 0.000000000000000000, -1.000000000000000000, 0.000000000000000000 ) ) ;
#28029=ORIENTED_EDGE ( 'NONE', *, *, #68926, .F. ) ;
#28030=VERTEX_POINT ( 'NONE', #59363 ) ;
#28034=VERTEX_POINT ( 'NONE', #52085 ) ;
#28067=CARTESIAN_POINT ( 'NONE',  ( -158.9822249764575020, 20.32000000000000028, 139.6999999999999886 ) ) ;
#28090=CIRCLE ( 'NONE', #45447, 12.69999999999998863 ) ;
#28091=ORIENTED_EDGE ( 'NONE', *, *, #46792, .F. ) ;
#28094=ORIENTED_EDGE ( 'NONE', *, *, #41731, .F. ) ;
#28105=ORIENTED_EDGE ( 'NONE', *, *, #43504, .F. ) ;
#28135=EDGE_CURVE ( 'NONE', #31769, #64268, #82976, .T. ) ;
#28138=DIRECTION ( 'NONE',  ( 0.000000000000000000, 1.000000000000000000, 0.000000000000000000 ) ) ;
#28148=ORIENTED_EDGE ( 'NONE', *, *, #59929, .T. ) ;
#28150=CARTESIAN_POINT ( 'NONE',  ( 124.0809317655093764, 45.78809315698909899, -40.60603252858108903 ) ) ;
#28156=EDGE_CURVE ( 'NONE', #57167, #13204, #13916, .T. ) ;
#28169=DIRECTION ( 'NONE',  ( 0.000000000000000000, 0.000000000000000000, -1.000000000000000000 ) ) ;
#28175=CARTESIAN_POINT ( 'NONE',  ( 3.110602869834275287E-15, 2.031999999999865025, -25.39999999999999858 ) ) ;
#28205=ADVANCED_FACE ( 'NONE', ( #284 ), #35691, .T. ) ;
#28207=CARTESIAN_POINT ( 'NONE',  ( 123.4696824136382105, 20.32000000000000028, -179.8898777604649979 ) ) ;
#28224=FACE_BOUND ( 'NONE', #49213, .T. ) ;
#28246=VERTEX_POINT ( 'NONE', #14825 ) ;
#28253=ORIENTED_EDGE ( 'NONE', *, *, #19558, .T. ) ;
#28270=VECTOR ( 'NONE', #85457, 1000.000000000000000 ) ;
#28285=ORIENTED_EDGE ( 'NONE', *, *, #33703, .F. ) ;
#28288=EDGE_CURVE ( 'NONE', #69150, #60648, #42051, .T. ) ;
#28290=AXIS2_PLACEMENT_3D ( 'NONE', #33364, #39282, #67427 ) ;
#28297=CARTESIAN_POINT ( 'NONE',  ( 11.58771219026867527, 77.33901287876103936, 130.0408192685323741 ) ) ;
#28326=CARTESIAN_POINT ( 'NONE',  ( 23.27731929905162289, 53.53152164542878211, 30.16249999999999787 ) ) ;
#28339=CIRCLE ( 'NONE', #60296, 6.349999999999994316 ) ;
#28341=CIRCLE ( 'NONE', #6630, 1.523999999999053889 ) ;
#28350=AXIS2_PLACEMENT_3D ( 'NONE', #19724, #41493, #48297 ) ;
#28357=EDGE_CURVE ( 'NONE', #79893, #57125, #85219, .T. ) ;
#28362=CARTESIAN_POINT ( 'NONE',  ( 148.0533267522749838, 20.32000000000000028, -160.2664750769289697 ) ) ;
#28386=CARTESIAN_POINT ( 'NONE',  ( -121.5196524476492215, 74.38311268679323973, 47.72707487632980161 ) ) ;
#28469=ORIENTED_EDGE ( 'NONE', *, *, #89603, .F. ) ;
#28507=CARTESIAN_POINT ( 'NONE',  ( 0.000000000000000000, 8.255000000000000782, 0.000000000000000000 ) ) ;
#28510=CARTESIAN_POINT ( 'NONE',  ( 22.56045403639487290, 58.71535241393495141, 30.70317686336609597 ) ) ;
#28532=CARTESIAN_POINT ( 'NONE',  ( -179.8898777604655095, 20.32000000000000028, 114.2999999999999972 ) ) ;
#28534=ORIENTED_EDGE ( 'NONE', *, *, #3902, .F. ) ;
#28536=CIRCLE ( 'NONE', #67709, 179.8898777604655095 ) ;
#28545=DIRECTION ( 'NONE',  ( 0.000000000000000000, -1.000000000000000000, 0.000000000000000000 ) ) ;
#28563=EDGE_CURVE ( 'NONE', #60315, #7937, #11576, .T. ) ;
#28567=CARTESIAN_POINT ( 'NONE',  ( 196.2150000000000034, 43.68799999999999528, 44.45000000000000284 ) ) ;
#28571=DIRECTION ( 'NONE',  ( -0.000000000000000000, 1.000000000000000000, -0.000000000000000000 ) ) ;
#28573=ORIENTED_EDGE ( 'NONE', *, *, #30339, .F. ) ;
#28583=CARTESIAN_POINT ( 'NONE',  ( 12.69999999999999929, 82.54999999999999716, -179.8908777604655143 ) ) ;
#28609=CARTESIAN_POINT ( 'NONE',  ( 124.4929055791733248, 46.65249925418791577, -39.32612047173540049 ) ) ;
#28618=CARTESIAN_POINT ( 'NONE',  ( -123.4696824136392053, 0.000000000000000000, -179.8898777604655095 ) ) ;
#28627=CARTESIAN_POINT ( 'NONE',  ( 141.3509999999999991, 20.32000000000000028, 141.3509999999999991 ) ) ;
#28637=CARTESIAN_POINT ( 'NONE',  ( 123.2646066340916349, 73.09139164160541213, 43.02039627876905570 ) ) ;
#28642=CARTESIAN_POINT ( 'NONE',  ( -31.75000000000000000, 17.78000000000000114, 3.175000000000219647 ) ) ;
#28651=CARTESIAN_POINT ( 'NONE',  ( -147.4575741623270062, 20.32000000000000028, 135.2444258376732193 ) ) ;
#28654=EDGE_CURVE ( 'NONE', #54956, #67371, #16225, .T. ) ;
#28660=VERTEX_POINT ( 'NONE', #13803 ) ;
#28681=VECTOR ( 'NONE', #60184, 1000.000000000000000 ) ;
#28698=AXIS2_PLACEMENT_3D ( 'NONE', #38504, #11712, #66205 ) ;
#28720=VERTEX_POINT ( 'NONE', #9232 ) ;
#28722=DIRECTION ( 'NONE',  ( -1.047445008332813989E-14, 0.000000000000000000, -1.000000000000000000 ) ) ;
#28738=VECTOR ( 'NONE', #23106, 1000.000000000000000 ) ;
#28769=CARTESIAN_POINT ( 'NONE',  ( -135.2444258376730204, 20.32000000000000028, 147.4575741623271767 ) ) ;
#28800=CARTESIAN_POINT ( 'NONE',  ( 208.9149999999999920, 30.98800000000000310, 57.14999999999999858 ) ) ;
#28805=VECTOR ( 'NONE', #10325, 1000.000000000000000 ) ;
#28820=LINE ( 'NONE', #43772, #75052 ) ;
#28843=ORIENTED_EDGE ( 'NONE', *, *, #50519, .T. ) ;
#28850=CARTESIAN_POINT ( 'NONE',  ( -113.0224119320542400, 68.60953631961947963, 65.35142026045585339 ) ) ;
#28879=CARTESIAN_POINT ( 'NONE',  ( -215.9000000000000057, 101.5999999999999943, 146.9389999999999930 ) ) ;
#28943=ADVANCED_FACE ( 'NONE', ( #47638 ), #48515, .T. ) ;
#28971=ORIENTED_EDGE ( 'NONE', *, *, #31173, .T. ) ;
#28976=VECTOR ( 'NONE', #38298, 1000.000000000000000 ) ;
#28979=DIRECTION ( 'NONE',  ( 0.000000000000000000, -1.000000000000000000, 0.000000000000000000 ) ) ;
#28981=CARTESIAN_POINT ( 'NONE',  ( 23.23280569011280505, 55.35248209492627325, 30.19701270168030405 ) ) ;
#29038=ORIENTED_EDGE ( 'NONE', *, *, #66840, .F. ) ;
#29039=VECTOR ( 'NONE', #35392, 1000.000000000000000 ) ;
#29069=CARTESIAN_POINT ( 'NONE',  ( 124.7270369540910622, 47.39308626936165325, -38.57547257139917463 ) ) ;
#29083=PLANE ( 'NONE',  #68857 ) ;
#29092=CARTESIAN_POINT ( 'NONE',  ( 183.5150000000000148, 37.33800000000000097, 32.46912895322940074 ) ) ;
#29093=CARTESIAN_POINT ( 'NONE',  ( 160.2664750769289697, 20.32000000000000028, 148.0533267522752112 ) ) ;
#29109=CARTESIAN_POINT ( 'NONE',  ( -31.75000000000000000, 24.56180297284579694, -3.174999999999779998 ) ) ;
#29119=EDGE_CURVE ( 'NONE', #15522, #20262, #83096, .T. ) ;
#29177=EDGE_CURVE ( 'NONE', #5363, #23986, #50786, .T. ) ;
#29184=AXIS2_PLACEMENT_3D ( 'NONE', #60628, #67006, #80657 ) ;
#29218=CARTESIAN_POINT ( 'NONE',  ( 12.10537486922539863, 78.70349232879850376, 129.9937543560634481 ) ) ;
#29279=CARTESIAN_POINT ( 'NONE',  ( 0.000000000000000000, 2.269999999999994245, 0.000000000000000000 ) ) ;
#29288=ORIENTED_EDGE ( 'NONE', *, *, #59088, .T. ) ;
#29305=ORIENTED_EDGE ( 'NONE', *, *, #37185, .F. ) ;
#29318=ORIENTED_EDGE ( 'NONE', *, *, #18001, .T. ) ;
#29323=ORIENTED_EDGE ( 'NONE', *, *, #75319, .F. ) ;
#29330=LINE ( 'NONE', #15252, #53623 ) ;
#29331=CARTESIAN_POINT ( 'NONE',  ( 0.000000000000000000, 20.32000000000000028, 0.000000000000000000 ) ) ;
#29356=ORIENTED_EDGE ( 'NONE', *, *, #13403, .T. ) ;
#29427=CARTESIAN_POINT ( 'NONE',  ( 0.000000000000000000, 20.32000000000000028, 0.000000000000000000 ) ) ;
#29433=DIRECTION ( 'NONE',  ( 0.000000000000000000, 0.000000000000000000, -1.000000000000000000 ) ) ;
#29448=LINE ( 'NONE', #86203, #28738 ) ;
#29503=CARTESIAN_POINT ( 'NONE',  ( -23.27731929905162289, 53.08310398829927834, 30.16249999999998721 ) ) ;
#29505=DIRECTION ( 'NONE',  ( 0.000000000000000000, 0.000000000000000000, -1.000000000000000000 ) ) ;
#29520=EDGE_CURVE ( 'NONE', #4943, #44354, #58598, .T. ) ;
#29526=DIRECTION ( 'NONE',  ( 0.000000000000000000, 0.000000000000000000, 1.000000000000000000 ) ) ;
#29531=EDGE_LOOP ( 'NONE', ( #87144, #3105, #32702, #36704 ) ) ;
#29542=CARTESIAN_POINT ( 'NONE',  ( 123.0975592459876822, 73.27678779245984231, 43.49559623943592612 ) ) ;
#29544=ORIENTED_EDGE ( 'NONE', *, *, #89065, .F. ) ;
#29563=ORIENTED_EDGE ( 'NONE', *, *, #80592, .F. ) ;
#29572=ORIENTED_EDGE ( 'NONE', *, *, #42504, .F. ) ;
#29620=ADVANCED_FACE ( 'NONE', ( #41188 ), #42085, .F. ) ;
#29656=CARTESIAN_POINT ( 'NONE',  ( 11.73526988453661346, 77.69473719258546396, 130.0275070810828311 ) ) ;
#29658=CARTESIAN_POINT ( 'NONE',  ( 50.03799999999999670, 0.000000000000000000, 206.3750000000000000 ) ) ;
#29683=CARTESIAN_POINT ( 'NONE',  ( 4.811414547114572393, 94.30331772199949114, 130.4673117074386823 ) ) ;
#29697=VERTEX_POINT ( 'NONE', #56615 ) ;
#29743=EDGE_CURVE ( 'NONE', #18491, #85626, #84804, .T. ) ;
#29749=CARTESIAN_POINT ( 'NONE',  ( -126.8151218862759180, 59.90404055707092823, 31.02911582310609973 ) ) ;
#29780=DIRECTION ( 'NONE',  ( -1.000000000000000000, 0.000000000000000000, 0.000000000000000000 ) ) ;
#29792=CARTESIAN_POINT ( 'NONE',  ( -147.4575741623271767, 101.5999999999999943, -135.2444258376735888 ) ) ;
#29830=CARTESIAN_POINT ( 'NONE',  ( -5.303323664314122610, 94.09012423098154443, 130.4482521264637285 ) ) ;
#29849=CARTESIAN_POINT ( 'NONE',  ( 57.91199999999999903, 20.32000000000000028, 178.6098374884404905 ) ) ;
#29866=CARTESIAN_POINT ( 'NONE',  ( -110.7653435595065901, 44.45000000000000284, 69.10794311903988785 ) ) ;
#29874=FACE_OUTER_BOUND ( 'NONE', #88311, .T. ) ;
#29877=ORIENTED_EDGE ( 'NONE', *, *, #64054, .T. ) ;
#29878=EDGE_CURVE ( 'NONE', #81504, #60315, #71277, .T. ) ;
#29919=DIRECTION ( 'NONE',  ( -1.000000000000000000, 7.980413499659419871E-32, 0.000000000000000000 ) ) ;
#29945=DIRECTION ( 'NONE',  ( 0.000000000000000000, 0.000000000000000000, -1.000000000000000000 ) ) ;
#29948=DIRECTION ( 'NONE',  ( -0.000000000000000000, 1.000000000000000000, 0.000000000000000000 ) ) ;
#29978=VECTOR ( 'NONE', #49375, 1000.000000000000000 ) ;
#29996=DIRECTION ( 'NONE',  ( 0.000000000000000000, -1.000000000000000000, 0.000000000000000000 ) ) ;
#30007=FACE_OUTER_BOUND ( 'NONE', #31506, .T. ) ;
#30012=CARTESIAN_POINT ( 'NONE',  ( -215.9000000000000057, 0.000000000000000000, -45.33899999999999864 ) ) ;
#30019=CARTESIAN_POINT ( 'NONE',  ( -215.9000000000000057, 0.000000000000000000, 146.9389999999999930 ) ) ;
#30026=ORIENTED_EDGE ( 'NONE', *, *, #969, .F. ) ;
#30029=EDGE_CURVE ( 'NONE', #54555, #30833, #26324, .T. ) ;
#30037=AXIS2_PLACEMENT_3D ( 'NONE', #23441, #77490, #30676 ) ;
#30079=ORIENTED_EDGE ( 'NONE', *, *, #34196, .F. ) ;
#30097=AXIS2_PLACEMENT_3D ( 'NONE', #39127, #65930, #66830 ) ;
#30103=CIRCLE ( 'NONE', #1054, 34.13125000000000142 ) ;
#30124=CARTESIAN_POINT ( 'NONE',  ( -109.2774118001976120, 53.97500000000000142, 71.43750000000000000 ) ) ;
#30142=CARTESIAN_POINT ( 'NONE',  ( -75.61066417432020614, 101.5999999999999943, 177.0380000000000109 ) ) ;
#30181=CARTESIAN_POINT ( 'NONE',  ( 0.000000000000000000, 44.45000000000000284, 0.000000000000000000 ) ) ;
#30193=EDGE_CURVE ( 'NONE', #11178, #56606, #86028, .T. ) ;
#30199=EDGE_CURVE ( 'NONE', #14989, #82724, #44204, .T. ) ;
#30219=DIRECTION ( 'NONE',  ( 0.000000000000000000, 1.000000000000000000, 0.000000000000000000 ) ) ;
#30241=LINE ( 'NONE', #23878, #52452 ) ;
#30243=EDGE_LOOP ( 'NONE', ( #51300, #30263 ) ) ;
#30247=ORIENTED_EDGE ( 'NONE', *, *, #74004, .T. ) ;
#30263=ORIENTED_EDGE ( 'NONE', *, *, #63536, .T. ) ;
#30269=CARTESIAN_POINT ( 'NONE',  ( -50.03799999999999670, 20.32000000000000028, 178.6098374884404905 ) ) ;
#30274=CARTESIAN_POINT ( 'NONE',  ( -10.56235306858779133, 89.60171684026197170, 130.1280363297576059 ) ) ;
#30304=ORIENTED_EDGE ( 'NONE', *, *, #50234, .T. ) ;
#30312=VECTOR ( 'NONE', #17639, 1000.000000000000000 ) ;
#30325=CARTESIAN_POINT ( 'NONE',  ( 4.804656715581928417, 70.00525152650509142, 37.80205776086838654 ) ) ;
#30333=CARTESIAN_POINT ( 'NONE',  ( -50.03799999999999670, 20.32000000000000028, 206.3750000000000000 ) ) ;
#30335=CIRCLE ( 'NONE', #49163, 6.350000000000659561 ) ;
#30339=EDGE_CURVE ( 'NONE', #66654, #76607, #55366, .T. ) ;
#30386=ORIENTED_EDGE ( 'NONE', *, *, #19350, .F. ) ;
#30391=EDGE_LOOP ( 'NONE', ( #86802, #13236, #10624, #50881, #19517, #27197, #58468, #56942, #74406, #58859, #61343, #52768, #51702, #34279, #75484, #60220, #27345, #39456, #46114, #68164, #7842, #39424, #18555, #15892, #3454, #30500, #22069, #6445, #3714, #15569, #28029, #50427, #69176, #59504, #16414, #16177, #37101, #50635, #36506, #62082, #16350, #82916, #71512, #2395, #74730, #43568, #39715, #24213, #57478 ) ) ;
#30408=ORIENTED_EDGE ( 'NONE', *, *, #52309, .F. ) ;
#30417=DIRECTION ( 'NONE',  ( 0.000000000000000000, -1.000000000000000000, 0.000000000000000000 ) ) ;
#30439=CARTESIAN_POINT ( 'NONE',  ( 0.000000000000000000, 101.5999999999999943, 0.000000000000000000 ) ) ;
#30452=AXIS2_PLACEMENT_3D ( 'NONE', #88847, #10847, #24493 ) ;
#30453=FACE_OUTER_BOUND ( 'NONE', #69610, .T. ) ;
#30475=AXIS2_PLACEMENT_3D ( 'NONE', #8606, #23142, #72167 ) ;
#30500=ORIENTED_EDGE ( 'NONE', *, *, #43224, .F. ) ;
#30501=SURFACE_STYLE_FILL_AREA ( #3685 ) ;
#30515=ADVANCED_FACE ( 'NONE', ( #58950 ), #86238, .T. ) ;
#30569=EDGE_CURVE ( 'NONE', #13373, #51663, #79888, .T. ) ;
#30578=ORIENTED_EDGE ( 'NONE', *, *, #20866, .T. ) ;
#30584=DIRECTION ( 'NONE',  ( 0.000000000000000000, -1.000000000000000000, 0.000000000000000000 ) ) ;
#30593=CIRCLE ( 'NONE', #3039, 218.1859999999999786 ) ;
#30602=DIRECTION ( 'NONE',  ( 0.000000000000000000, 0.000000000000000000, 1.000000000000000000 ) ) ;
#30609=DIRECTION ( 'NONE',  ( 0.000000000000000000, -1.000000000000000000, 0.000000000000000000 ) ) ;
#30664=CARTESIAN_POINT ( 'NONE',  ( 196.2150000000000034, 30.98800000000000310, 44.45000000000000284 ) ) ;
#30676=DIRECTION ( 'NONE',  ( 1.000000000000000000, 0.000000000000000000, 0.000000000000000000 ) ) ;
#30684=EDGE_CURVE ( 'NONE', #65669, #83014, #38080, .T. ) ;
#30700=APPLICATION_CONTEXT ( 'automotive_design' ) ;
#30710=CARTESIAN_POINT ( 'NONE',  ( -7.066900032206758553, 93.10220157233833049, 130.3645965947815455 ) ) ;
#30712=ORIENTED_EDGE ( 'NONE', *, *, #20318, .F. ) ;
#30715=CARTESIAN_POINT ( 'NONE',  ( 126.5426538762358604, 45.18699313767324099, 32.12251388581796618 ) ) ;
#30716=VECTOR ( 'NONE', #27305, 1000.000000000000000 ) ;
#30721=CARTESIAN_POINT ( 'NONE',  ( -31.75000000000000000, 24.56180297284579694, -3.174999999999779998 ) ) ;
#30723=ORIENTED_EDGE ( 'NONE', *, *, #80061, .F. ) ;
#30755=AXIS2_PLACEMENT_3D ( 'NONE', #84823, #57537, #70738 ) ;
#30783=VECTOR ( 'NONE', #59913, 1000.000000000000000 ) ;
#30833=VERTEX_POINT ( 'NONE', #13955 ) ;
#30838=CARTESIAN_POINT ( 'NONE',  ( 0.000000000000000000, 17.78000000000000114, 0.000000000000000000 ) ) ;
#30850=CARTESIAN_POINT ( 'NONE',  ( 124.9714502624620707, 48.43269546781706936, -37.77605326482454018 ) ) ;
#30877=CONICAL_SURFACE ( 'NONE', #68553, 161.5439999999999827, 0.08726646259971625186 ) ;
#30880=CARTESIAN_POINT ( 'NONE',  ( 110.8238305604934624, 63.68415021057004566, 69.01438277976548363 ) ) ;
#30947=FACE_OUTER_BOUND ( 'NONE', #12378, .T. ) ;
#30970=VERTEX_POINT ( 'NONE', #71619 ) ;
#30999=DIRECTION ( 'NONE',  ( 0.000000000000000000, 1.000000000000000000, 0.000000000000000000 ) ) ;
#31017=VECTOR ( 'NONE', #32582, 1000.000000000000000 ) ;
#31026=EDGE_CURVE ( 'NONE', #17885, #15997, #23558, .T. ) ;
#31030=ORIENTED_EDGE ( 'NONE', *, *, #49250, .T. ) ;
#31056=VERTEX_POINT ( 'NONE', #51148 ) ;
#31065=CARTESIAN_POINT ( 'NONE',  ( -126.8390414488319635, 59.56676029426186858, 30.93113591434403276 ) ) ;
#31112=LINE ( 'NONE', #38823, #35617 ) ;
#31121=ADVANCED_FACE ( 'NONE', ( #72061 ), #51588, .T. ) ;
#31140=CIRCLE ( 'NONE', #45570, 218.1859999999999786 ) ;
#31148=CARTESIAN_POINT ( 'NONE',  ( -0.7868074802740107065, 95.24999999999995737, 130.5560000000000400 ) ) ;
#31166=EDGE_CURVE ( 'NONE', #13980, #62710, #68474, .T. ) ;
#31173=EDGE_CURVE ( 'NONE', #7552, #59397, #32937, .T. ) ;
#31179=DIRECTION ( 'NONE',  ( 0.000000000000000000, -1.000000000000000000, 0.000000000000000000 ) ) ;
#31195=DIRECTION ( 'NONE',  ( -1.000000000000000000, 0.000000000000000000, 0.000000000000000000 ) ) ;
#31210=EDGE_CURVE ( 'NONE', #45792, #83969, #52893, .T. ) ;
#31217=CARTESIAN_POINT ( 'NONE',  ( 131.3179999999999836, 53.97500000000000142, 71.43750000000000000 ) ) ;
#31226=ORIENTED_EDGE ( 'NONE', *, *, #83344, .T. ) ;
#31255=AXIS2_PLACEMENT_3D ( 'NONE', #19627, #19190, #88246 ) ;
#31264=CARTESIAN_POINT ( 'NONE',  ( 122.3615910276390650, 60.60584201542124561, -45.52561893181081132 ) ) ;
#31294=CARTESIAN_POINT ( 'NONE',  ( 0.000000000000000000, 44.45000000000000284, 0.000000000000000000 ) ) ;
#31296=DIRECTION ( 'NONE',  ( 0.000000000000000000, -1.000000000000000000, 0.000000000000000000 ) ) ;
#31303=DIRECTION ( 'NONE',  ( 0.000000000000000000, 0.000000000000000000, 1.000000000000000000 ) ) ;
#31308=CARTESIAN_POINT ( 'NONE',  ( 109.7396867053641643, 59.36954314920819797, 70.72544642611300958 ) ) ;
#31314=FACE_BOUND ( 'NONE', #9394, .T. ) ;
#31315=LINE ( 'NONE', #9552, #53677 ) ;
#31320=LINE ( 'NONE', #72678, #34582 ) ;
#31326=CARTESIAN_POINT ( 'NONE',  ( 0.000000000000000000, 82.54999999999999716, 206.3750000000000000 ) ) ;
#31327=AXIS2_PLACEMENT_3D ( 'NONE', #48785, #76515, #27465 ) ;
#31335=DIRECTION ( 'NONE',  ( 0.000000000000000000, 1.000000000000000000, 0.000000000000000000 ) ) ;
#31340=ORIENTED_EDGE ( 'NONE', *, *, #64375, .F. ) ;
#31342=CARTESIAN_POINT ( 'NONE',  ( -179.8898777604655095, 101.5999999999999943, -12.69999999999999929 ) ) ;
#31343=EDGE_CURVE ( 'NONE', #43788, #8973, #17761, .T. ) ;
#31348=CIRCLE ( 'NONE', #13974, 34.13125000000000142 ) ;
#31358=ADVANCED_FACE ( 'NONE', ( #75640 ), #56514, .F. ) ;
#31362=LINE ( 'NONE', #53568, #38515 ) ;
#31370=DIRECTION ( 'NONE',  ( 0.000000000000000000, 0.000000000000000000, -1.000000000000000000 ) ) ;
#31384=CARTESIAN_POINT ( 'NONE',  ( -187.8075999999999794, 20.32000000000000028, -3.174999999999999822 ) ) ;
#31429=CARTESIAN_POINT ( 'NONE',  ( 183.5150000000000148, 53.21300000000000097, 59.96543552338529537 ) ) ;
#31466=VERTEX_POINT ( 'NONE', #57866 ) ;
#31477=LINE ( 'NONE', #24239, #45830 ) ;
#31479=VERTEX_POINT ( 'NONE', #22919 ) ;
#31490=DIRECTION ( 'NONE',  ( 0.000000000000000000, 1.000000000000000000, 0.000000000000000000 ) ) ;
#31499=ORIENTED_EDGE ( 'NONE', *, *, #30193, .F. ) ;
#31506=EDGE_LOOP ( 'NONE', ( #75178, #21655, #64804, #64897 ) ) ;
#31510=AXIS2_PLACEMENT_3D ( 'NONE', #37434, #71524, #84264 ) ;
#31512=EDGE_LOOP ( 'NONE', ( #8014, #19842, #40828, #38227, #81162, #82040 ) ) ;
#31515=ADVANCED_FACE ( 'NONE', ( #44670, #17431 ), #38309, .F. ) ;
#31537=CARTESIAN_POINT ( 'NONE',  ( -13.28435107523728220, 68.09058761799009574, 35.73330652649276828 ) ) ;
#31544=DIRECTION ( 'NONE',  ( 0.000000000000000000, -1.000000000000000000, 0.000000000000000000 ) ) ;
#31574=EDGE_CURVE ( 'NONE', #6845, #88991, #26034, .T. ) ;
#31589=CARTESIAN_POINT ( 'NONE',  ( -4.941314120920629271, 94.24933258371393663, 130.4624588263053226 ) ) ;
#31605=ORIENTED_EDGE ( 'NONE', *, *, #37990, .F. ) ;
#31617=ORIENTED_EDGE ( 'NONE', *, *, #80865, .F. ) ;
#31643=ORIENTED_EDGE ( 'NONE', *, *, #57990, .T. ) ;
#31660=CARTESIAN_POINT ( 'NONE',  ( 0.000000000000000000, 44.45000000000000284, 130.5560000000000116 ) ) ;
#31688=ORIENTED_EDGE ( 'NONE', *, *, #461, .F. ) ;
#31692=DIRECTION ( 'NONE',  ( 0.000000000000000000, -1.000000000000000000, 0.000000000000000000 ) ) ;
#31721=CARTESIAN_POINT ( 'NONE',  ( -148.0533267522759786, 0.000000000000000000, -160.2664750769289697 ) ) ;
#31729=EDGE_LOOP ( 'NONE', ( #74955, #67282 ) ) ;
#31754=DIRECTION ( 'NONE',  ( 0.000000000000000000, -0.000000000000000000, -1.000000000000000000 ) ) ;
#31759=CARTESIAN_POINT ( 'NONE',  ( 110.3862196296579299, 62.23620089231086894, 69.71192191839192276 ) ) ;
#31768=CARTESIAN_POINT ( 'NONE',  ( 3.110602869834275287E-15, 8.255000000000000782, -25.39999999999999858 ) ) ;
#31769=VERTEX_POINT ( 'NONE', #13301 ) ;
#31770=VECTOR ( 'NONE', #22861, 1000.000000000000000 ) ;
#31785=AXIS2_PLACEMENT_3D ( 'NONE', #69059, #21822, #63138 ) ;
#31792=LINE ( 'NONE', #79073, #52282 ) ;
#31825=AXIS2_PLACEMENT_3D ( 'NONE', #61601, #6657, #41602 ) ;
#31854=ORIENTED_EDGE ( 'NONE', *, *, #80762, .T. ) ;
#31873=CARTESIAN_POINT ( 'NONE',  ( 31.75000000000000000, 8.255000000000000782, -3.174999999999999822 ) ) ;
#31963=DIRECTION ( 'NONE',  ( -1.047445008332813989E-14, 0.000000000000000000, -1.000000000000000000 ) ) ;
#31983=CARTESIAN_POINT ( 'NONE',  ( -16.16525963187149983, 66.64697067941781938, 34.50616615423284372 ) ) ;
#31992=DIRECTION ( 'NONE',  ( 0.000000000000000000, -1.000000000000000000, 0.000000000000000000 ) ) ;
#32045=CARTESIAN_POINT ( 'NONE',  ( 127.0122246826498866, 52.32189085609214629, 30.21215538458211824 ) ) ;
#32052=ORIENTED_EDGE ( 'NONE', *, *, #67572, .F. ) ;
#32058=DIRECTION ( 'NONE',  ( 0.000000000000000000, 0.000000000000000000, -1.000000000000000000 ) ) ;
#32064=CARTESIAN_POINT ( 'NONE',  ( -109.7630092984566801, 59.52527381720275201, 70.68955123198077217 ) ) ;
#32091=FACE_OUTER_BOUND ( 'NONE', #82726, .T. ) ;
#32116=ADVANCED_FACE ( 'NONE', ( #30947 ), #86370, .F. ) ;
#32163=AXIS2_PLACEMENT_3D ( 'NONE', #7424, #70556, #48282 ) ;
#32188=ORIENTED_EDGE ( 'NONE', *, *, #22220, .T. ) ;
#32201=CARTESIAN_POINT ( 'NONE',  ( 120.2829076421031544, 74.61365623713926709, 50.76363797295935854 ) ) ;
#32235=PLANE ( 'NONE',  #9502 ) ;
#32243=EDGE_CURVE ( 'NONE', #52020, #61274, #26366, .T. ) ;
#32245=ADVANCED_FACE ( 'NONE', ( #81794 ), #19547, .T. ) ;
#32261=CARTESIAN_POINT ( 'NONE',  ( 173.9900000000000091, 20.32000000000000028, -71.37400000000000944 ) ) ;
#32272=DIRECTION ( 'NONE',  ( -1.004914528670390057E-14, 0.000000000000000000, 1.000000000000000000 ) ) ;
#32278=ORIENTED_EDGE ( 'NONE', *, *, #39113, .T. ) ;
#32309=VERTEX_POINT ( 'NONE', #39542 ) ;
#32327=EDGE_CURVE ( 'NONE', #66477, #71033, #12930, .T. ) ;
#32341=CARTESIAN_POINT ( 'NONE',  ( 11.72308525109137634, 87.43461473045920229, 130.0286063932555294 ) ) ;
#32352=ORIENTED_EDGE ( 'NONE', *, *, #27560, .F. ) ;
#32389=DIRECTION ( 'NONE',  ( 0.000000000000000000, -1.000000000000000000, 0.000000000000000000 ) ) ;
#32395=AXIS2_PLACEMENT_3D ( 'NONE', #20722, #62938, #42483 ) ;
#32410=VERTEX_POINT ( 'NONE', #20006 ) ;
#32415=EDGE_CURVE ( 'NONE', #58184, #30833, #20456, .T. ) ;
#32468=AXIS2_PLACEMENT_3D ( 'NONE', #26085, #52404, #24740 ) ;
#32473=CARTESIAN_POINT ( 'NONE',  ( -187.8075999999999794, 101.5999999999999943, -9.525000000000000355 ) ) ;
#32518=EDGE_LOOP ( 'NONE', ( #754, #78348, #87901, #66418, #52281, #12082 ) ) ;
#32528=CARTESIAN_POINT ( 'NONE',  ( -4.046498181513055847, 70.50995738321196882, 130.4933223593253047 ) ) ;
#32548=ADVANCED_FACE ( 'NONE', ( #57188 ), #35858, .T. ) ;
#32564=ORIENTED_EDGE ( 'NONE', *, *, #9236, .T. ) ;
#32582=DIRECTION ( 'NONE',  ( 0.000000000000000000, -1.000000000000000000, 0.000000000000000000 ) ) ;
#32586=DIRECTION ( 'NONE',  ( -0.000000000000000000, 1.000000000000000000, 0.000000000000000000 ) ) ;
#32631=LINE ( 'NONE', #88064, #49050 ) ;
#32633=DIRECTION ( 'NONE',  ( 0.000000000000000000, 0.000000000000000000, -1.000000000000000000 ) ) ;
#32634=VERTEX_POINT ( 'NONE', #54717 ) ;
#32638=ADVANCED_FACE ( 'NONE', ( #13422 ), #53819, .F. ) ;
#32645=EDGE_CURVE ( 'NONE', #32309, #75634, #11489, .T. ) ;
#32650=CARTESIAN_POINT ( 'NONE',  ( -186.2398777604655038, 0.000000000000000000, -6.349999999999999645 ) ) ;
#32652=CARTESIAN_POINT ( 'NONE',  ( 113.1214584048637732, 68.77817172032477799, 65.17982383002866698 ) ) ;
#32666=UNCERTAINTY_MEASURE_WITH_UNIT (LENGTH_MEASURE( 1.000000000000000082E-05 ), #45438, 'distance_accuracy_value', 'NONE');
#32667=DIRECTION ( 'NONE',  ( 3.491483361109380094E-15, 0.000000000000000000, 1.000000000000000000 ) ) ;
#32693=VECTOR ( 'NONE', #43577, 1000.000000000000000 ) ;
#32702=ORIENTED_EDGE ( 'NONE', *, *, #25884, .T. ) ;
#32706=EDGE_CURVE ( 'NONE', #79978, #4573, #76845, .T. ) ;
#32740=DIRECTION ( 'NONE',  ( -1.000000000000000000, 0.000000000000000000, -7.867884063170659983E-16 ) ) ;
#32755=ORIENTED_EDGE ( 'NONE', *, *, #9007, .F. ) ;
#32760=EDGE_CURVE ( 'NONE', #57180, #67629, #34748, .T. ) ;
#32799=CARTESIAN_POINT ( 'NONE',  ( 11.71935769674032279, 87.44354605777512290, 130.0289424465127581 ) ) ;
#32818=FACE_OUTER_BOUND ( 'NONE', #54354, .T. ) ;
#32831=CARTESIAN_POINT ( 'NONE',  ( -187.8075999999999794, 101.5999999999999943, -6.349999999999999645 ) ) ;
#32875=( GEOMETRIC_REPRESENTATION_CONTEXT ( 3 ) GLOBAL_UNCERTAINTY_ASSIGNED_CONTEXT ( ( #32666 ) ) GLOBAL_UNIT_ASSIGNED_CONTEXT ( ( #45438, #87257, #19543 ) ) REPRESENTATION_CONTEXT ( 'NONE', 'WORKASPACE' ) );
#32878=CARTESIAN_POINT ( 'NONE',  ( -23.18606991449689403, 55.71041480586442418, 30.23275321802606186 ) ) ;
#32884=DIRECTION ( 'NONE',  ( 0.000000000000000000, 0.000000000000000000, -1.000000000000000000 ) ) ;
#32889=EDGE_CURVE ( 'NONE', #89539, #20262, #675, .T. ) ;
#32932=ORIENTED_EDGE ( 'NONE', *, *, #3191, .T. ) ;
#32935=VECTOR ( 'NONE', #72021, 1000.000000000000000 ) ;
#32937=LINE ( 'NONE', #60185, #55407 ) ;
#32946=EDGE_CURVE ( 'NONE', #14773, #32309, #37887, .T. ) ;
#32955=EDGE_CURVE ( 'NONE', #78242, #59655, #51927, .T. ) ;
#32961=CARTESIAN_POINT ( 'NONE',  ( -110.2127075062171997, 61.58157470217958007, 69.98598948281733101 ) ) ;
#32964=AXIS2_PLACEMENT_3D ( 'NONE', #89149, #75521, #88267 ) ;
#32986=CARTESIAN_POINT ( 'NONE',  ( -11.71543264365797477, 77.64706452475591902, 130.0292962180824929 ) ) ;
#33009=LINE ( 'NONE', #18941, #14291 ) ;
#33030=VECTOR ( 'NONE', #83388, 1000.000000000000000 ) ;
#33046=FACE_OUTER_BOUND ( 'NONE', #11332, .T. ) ;
#33057=CARTESIAN_POINT ( 'NONE',  ( 124.8316159268321712, 57.68278277478432159, -38.23569996530863335 ) ) ;
#33068=CARTESIAN_POINT ( 'NONE',  ( 1.154229608196380665E-15, 152.3879256507328250, 9.425000000000000711 ) ) ;
#33093=AXIS2_PLACEMENT_3D ( 'NONE', #15868, #2238, #29945 ) ;
#33114=CARTESIAN_POINT ( 'NONE',  ( 131.3179999999999836, 53.97500000000000142, 30.16249999999999787 ) ) ;
#33161=CARTESIAN_POINT ( 'NONE',  ( -3.174999999999644995, 8.255000000000000782, 33.98325472291465132 ) ) ;
#33168=ORIENTED_EDGE ( 'NONE', *, *, #84781, .F. ) ;
#33182=CARTESIAN_POINT ( 'NONE',  ( 8.588557746091451506, 73.17833598766388548, 130.2737784290322338 ) ) ;
#33183=AXIS2_PLACEMENT_3D ( 'NONE', #16077, #78762, #37402 ) ;
#33185=FACE_OUTER_BOUND ( 'NONE', #17010, .T. ) ;
#33223=AXIS2_PLACEMENT_3D ( 'NONE', #11492, #39187, #26461 ) ;
#33232=ORIENTED_EDGE ( 'NONE', *, *, #54665, .T. ) ;
#33239=VECTOR ( 'NONE', #77691, 1000.000000000000000 ) ;
#33281=DIRECTION ( 'NONE',  ( 0.000000000000000000, -1.000000000000000000, 0.000000000000000000 ) ) ;
#33283=DIRECTION ( 'NONE',  ( 0.000000000000000000, 1.000000000000000000, 0.000000000000000000 ) ) ;
#33329=CARTESIAN_POINT ( 'NONE',  ( 0.000000000000000000, 8.255000000000000782, 0.000000000000000000 ) ) ;
#33340=CARTESIAN_POINT ( 'NONE',  ( 148.0533267522752112, 0.000000000000000000, 160.2664750769284865 ) ) ;
#33364=CARTESIAN_POINT ( 'NONE',  ( 0.000000000000000000, 152.3879256507328250, 0.000000000000000000 ) ) ;
#33380=DIRECTION ( 'NONE',  ( 0.000000000000000000, 0.000000000000000000, 1.000000000000000000 ) ) ;
#33384=CIRCLE ( 'NONE', #30475, 9.524999999999998579 ) ;
#33401=ORIENTED_EDGE ( 'NONE', *, *, #14209, .F. ) ;
#33412=CIRCLE ( 'NONE', #55108, 7.937500000000000000 ) ;
#33476=EDGE_CURVE ( 'NONE', #55433, #38579, #8289, .T. ) ;
#33479=VERTEX_POINT ( 'NONE', #48246 ) ;
#33490=AXIS2_PLACEMENT_3D ( 'NONE', #12028, #89679, #67878 ) ;
#33498=AXIS2_PLACEMENT_3D ( 'NONE', #11898, #18700, #74559 ) ;
#33503=FACE_OUTER_BOUND ( 'NONE', #89032, .T. ) ;
#33536=PLANE ( 'NONE',  #10330 ) ;
#33573=EDGE_LOOP ( 'NONE', ( #78362, #40765, #6787, #64322 ) ) ;
#33616=EDGE_CURVE ( 'NONE', #65725, #28720, #66813, .T. ) ;
#33633=DIRECTION ( 'NONE',  ( 0.000000000000000000, -1.000000000000000000, 0.000000000000000000 ) ) ;
#33648=LINE ( 'NONE', #81376, #37825 ) ;
#33670=VERTEX_POINT ( 'NONE', #66358 ) ;
#33703=EDGE_CURVE ( 'NONE', #76607, #18319, #67258, .T. ) ;
#33705=CARTESIAN_POINT ( 'NONE',  ( 8.220576097192926923, 92.23944561992415458, 130.2971762513506917 ) ) ;
#33768=DIRECTION ( 'NONE',  ( 0.000000000000000000, 0.000000000000000000, -1.000000000000000000 ) ) ;
#33787=AXIS2_PLACEMENT_3D ( 'NONE', #3851, #31544, #59247 ) ;
#33794=ORIENTED_EDGE ( 'NONE', *, *, #36461, .T. ) ;
#33813=ORIENTED_EDGE ( 'NONE', *, *, #74509, .T. ) ;
#33844=VECTOR ( 'NONE', #23535, 1000.000000000000000 ) ;
#33857=CARTESIAN_POINT ( 'NONE',  ( -112.8531487064678913, 68.31472480788332291, 65.64348722659526914 ) ) ;
#33864=ORIENTED_EDGE ( 'NONE', *, *, #30684, .T. ) ;
#33883=CARTESIAN_POINT ( 'NONE',  ( -10.19015296090227274, 74.96840031402189197, 130.1578716281692607 ) ) ;
#33931=LINE ( 'NONE', #61628, #31017 ) ;
#33933=CARTESIAN_POINT ( 'NONE',  ( -185.9961463128564958, 20.32000000000000028, -3.174999999999514877 ) ) ;
#33938=EDGE_LOOP ( 'NONE', ( #9095, #89325, #33168, #26753 ) ) ;
#33944=LINE ( 'NONE', #39859, #4046 ) ;
#33962=ORIENTED_EDGE ( 'NONE', *, *, #54665, .F. ) ;
#33971=CARTESIAN_POINT ( 'NONE',  ( -3.175000000000109956, 24.56180297284579694, -31.75000000000000000 ) ) ;
#33982=CARTESIAN_POINT ( 'NONE',  ( -187.8075999999999794, 20.32000000000000028, -9.525000000000000355 ) ) ;
#33993=CARTESIAN_POINT ( 'NONE',  ( 3.944304526105059924E-28, 95.25000000000000000, 130.5560000000000116 ) ) ;
#33994=AXIS2_PLACEMENT_3D ( 'NONE', #59681, #66508, #79722 ) ;
#34022=ORIENTED_EDGE ( 'NONE', *, *, #20701, .F. ) ;
#34027=CARTESIAN_POINT ( 'NONE',  ( 1.598849875094819542E-14, 44.45000000000000284, -130.5560000000000116 ) ) ;
#34029=CARTESIAN_POINT ( 'NONE',  ( 0.000000000000000000, 82.54999999999999716, -179.8908777604655143 ) ) ;
#34057=CARTESIAN_POINT ( 'NONE',  ( 75.61066417432020614, 101.5999999999999943, 177.0380000000000109 ) ) ;
#34065=CARTESIAN_POINT ( 'NONE',  ( 124.6708583049006194, 47.20033540421172802, -38.75675120859585121 ) ) ;
#34070=LINE ( 'NONE', #61774, #52046 ) ;
#34073=CARTESIAN_POINT ( 'NONE',  ( -141.3509999999999991, 101.5999999999999943, 141.3509999999999991 ) ) ;
#34078=ORIENTED_EDGE ( 'NONE', *, *, #32243, .T. ) ;
#34080=EDGE_CURVE ( 'NONE', #78334, #15725, #15897, .T. ) ;
#34082=VERTEX_POINT ( 'NONE', #1372 ) ;
#34104=EDGE_LOOP ( 'NONE', ( #69603, #61441, #59946, #10435 ) ) ;
#34108=LINE ( 'NONE', #82298, #30716 ) ;
#34170=CARTESIAN_POINT ( 'NONE',  ( -148.0533267522752112, 20.32000000000000028, 160.2664750769289697 ) ) ;
#34192=CARTESIAN_POINT ( 'NONE',  ( 3.175000000000334666, 24.56180297284579694, 31.75000000000000000 ) ) ;
#34196=EDGE_CURVE ( 'NONE', #44232, #28660, #25431, .T. ) ;
#34200=CARTESIAN_POINT ( 'NONE',  ( -158.9822249764580135, 20.32000000000000028, 107.9500000000000028 ) ) ;
#34247=VECTOR ( 'NONE', #81344, 1000.000000000000000 ) ;
#34248=VECTOR ( 'NONE', #83909, 1000.000000000000000 ) ;
#34273=DIRECTION ( 'NONE',  ( 0.000000000000000000, 1.000000000000000000, 0.000000000000000000 ) ) ;
#34279=ORIENTED_EDGE ( 'NONE', *, *, #30684, .F. ) ;
#34300=DIRECTION ( 'NONE',  ( 0.000000000000000000, 0.000000000000000000, 1.000000000000000000 ) ) ;
#34301=CARTESIAN_POINT ( 'NONE',  ( -122.1472860046453945, 74.08167498906739468, 46.10177541449112226 ) ) ;
#34303=ORIENTED_EDGE ( 'NONE', *, *, #29119, .T. ) ;
#34304=EDGE_CURVE ( 'NONE', #12226, #28034, #61634, .T. ) ;
#34360=CARTESIAN_POINT ( 'NONE',  ( -126.9262659221376310, 49.86651706459634426, 30.57119546983337344 ) ) ;
#34386=CYLINDRICAL_SURFACE ( 'NONE', #52055, 8.636000000000004562 ) ;
#34396=VERTEX_POINT ( 'NONE', #82571 ) ;
#34399=ORIENTED_EDGE ( 'NONE', *, *, #34304, .T. ) ;
#34401=ORIENTED_EDGE ( 'NONE', *, *, #79318, .T. ) ;
#34405=EDGE_CURVE ( 'NONE', #51500, #14773, #321, .T. ) ;
#34431=AXIS2_PLACEMENT_3D ( 'NONE', #51256, #78569, #9065 ) ;
#34443=CARTESIAN_POINT ( 'NONE',  ( 0.000000000000000000, 8.255000000000000782, 0.000000000000000000 ) ) ;
#34458=EDGE_CURVE ( 'NONE', #22713, #65669, #2313, .T. ) ;
#34517=CARTESIAN_POINT ( 'NONE',  ( 0.7859143630660275770, 69.84999999999999432, 130.5560000000000684 ) ) ;
#34566=VECTOR ( 'NONE', #78512, 1000.000000000000000 ) ;
#34569=CARTESIAN_POINT ( 'NONE',  ( 141.3509999999999991, 101.5999999999999943, 132.7150000000000034 ) ) ;
#34582=VECTOR ( 'NONE', #74456, 1000.000000000000000 ) ;
#34692=VECTOR ( 'NONE', #14078, 1000.000000000000000 ) ;
#34694=VERTEX_POINT ( 'NONE', #6465 ) ;
#34695=EDGE_CURVE ( 'NONE', #88388, #57559, #60981, .T. ) ;
#34724=DIRECTION ( 'NONE',  ( 0.000000000000000000, 0.000000000000000000, 1.000000000000000000 ) ) ;
#34731=ORIENTED_EDGE ( 'NONE', *, *, #70431, .T. ) ;
#34734=CARTESIAN_POINT ( 'NONE',  ( -33.98325472291460159, 24.56180297284579694, 3.175000000000234746 ) ) ;
#34748=LINE ( 'NONE', #77438, #40527 ) ;
#34755=CARTESIAN_POINT ( 'NONE',  ( -113.0572828966228514, 68.66927669777484766, 65.29107463701845404 ) ) ;
#34778=CARTESIAN_POINT ( 'NONE',  ( 3.174999999999889688, 17.78000000000000114, -31.75000000000000000 ) ) ;
#34781=CARTESIAN_POINT ( 'NONE',  ( -11.72449278718255172, 77.66876991058626345, 130.0284793542324167 ) ) ;
#34788=DIRECTION ( 'NONE',  ( -0.000000000000000000, 1.000000000000000000, -0.000000000000000000 ) ) ;
#34808=DIRECTION ( 'NONE',  ( -1.825781832977094422E-16, -0.4999999999999998890, 0.8660254037844387076 ) ) ;
#34838=CARTESIAN_POINT ( 'NONE',  ( -11.80546680113316071, 87.23253990012126735, 130.0211617397174848 ) ) ;
#34839=PRODUCT_DEFINITION_FORMATION_WITH_SPECIFIED_SOURCE ( 'ANY', '', #36229, .NOT_KNOWN. ) ;
#34844=CARTESIAN_POINT ( 'NONE',  ( -141.3509999999999991, 101.5999999999999943, 141.3509999999999991 ) ) ;
#34850=VERTEX_POINT ( 'NONE', #48671 ) ;
#34881=DIRECTION ( 'NONE',  ( 0.000000000000000000, 0.000000000000000000, 1.000000000000000000 ) ) ;
#34890=CARTESIAN_POINT ( 'NONE',  ( -194.1576000000000022, 101.5999999999999943, -45.33899999999999864 ) ) ;
#34900=ORIENTED_EDGE ( 'NONE', *, *, #55917, .T. ) ;
#34918=CARTESIAN_POINT ( 'NONE',  ( -215.9000000000000057, 0.000000000000000000, 146.9389999999999930 ) ) ;
#34969=CARTESIAN_POINT ( 'NONE',  ( 123.0962380253862705, 44.85295700224565962, -43.50008466296358023 ) ) ;
#34971=ORIENTED_EDGE ( 'NONE', *, *, #70161, .T. ) ;
#35021=EDGE_CURVE ( 'NONE', #49608, #67615, #53083, .T. ) ;
#35038=DIRECTION ( 'NONE',  ( -1.472650733923983947E-14, 0.000000000000000000, 1.000000000000000000 ) ) ;
#35040=CARTESIAN_POINT ( 'NONE',  ( 183.5150000000000148, 5.588000000000000078, 50.79999999999999716 ) ) ;
#35047=ORIENTED_EDGE ( 'NONE', *, *, #20971, .T. ) ;
#35078=CIRCLE ( 'NONE', #10463, 161.5439999999999827 ) ;
#35109=UNCERTAINTY_MEASURE_WITH_UNIT (LENGTH_MEASURE( 1.000000000000000082E-05 ), #20515, 'distance_accuracy_value', 'NONE');
#35117=FACE_OUTER_BOUND ( 'NONE', #46413, .T. ) ;
#35137=ORIENTED_EDGE ( 'NONE', *, *, #82429, .T. ) ;
#35163=LINE ( 'NONE', #77869, #49174 ) ;
#35191=CARTESIAN_POINT ( 'NONE',  ( -125.1495029386209552, 69.48255809094938229, 37.18183539621997369 ) ) ;
#35215=EDGE_LOOP ( 'NONE', ( #48316, #54464, #79207, #84974, #63323, #62348 ) ) ;
#35249=ORIENTED_EDGE ( 'NONE', *, *, #59816, .F. ) ;
#35258=FACE_OUTER_BOUND ( 'NONE', #6500, .T. ) ;
#35277=CARTESIAN_POINT ( 'NONE',  ( -11.75417947995160795, 87.35930891448199986, 130.0257995324023170 ) ) ;
#35310=CARTESIAN_POINT ( 'NONE',  ( -109.2774118001976120, 53.97500000000000142, 71.43750000000000000 ) ) ;
#35328=LINE ( 'NONE', #13119, #10034 ) ;
#35348=CARTESIAN_POINT ( 'NONE',  ( 160.2664750769284865, 101.5999999999999943, -148.0533267522753818 ) ) ;
#35392=DIRECTION ( 'NONE',  ( 0.000000000000000000, 0.000000000000000000, 1.000000000000000000 ) ) ;
#35394=EDGE_LOOP ( 'NONE', ( #7737, #25033, #6045, #61254 ) ) ;
#35428=VERTEX_POINT ( 'NONE', #18986 ) ;
#35442=CARTESIAN_POINT ( 'NONE',  ( 127.0239848601436563, 54.68407512302287188, 30.16250000000001563 ) ) ;
#35452=CARTESIAN_POINT ( 'NONE',  ( -31.75000000000000000, 8.255000000000000782, 3.175000000000219647 ) ) ;
#35495=DIRECTION ( 'NONE',  ( -0.9347835805883503157, 0.000000000000000000, 0.3552177606235690788 ) ) ;
#35523=DIRECTION ( 'NONE',  ( 0.000000000000000000, 1.000000000000000000, 0.000000000000000000 ) ) ;
#35528=CARTESIAN_POINT ( 'NONE',  ( 33.98325472291465132, 17.78000000000000114, 3.174999999999999822 ) ) ;
#35532=ORIENTED_EDGE ( 'NONE', *, *, #36972, .F. ) ;
#35549=CARTESIAN_POINT ( 'NONE',  ( -160.2664750769284865, 20.32000000000000028, 148.0533267522753818 ) ) ;
#35563=CARTESIAN_POINT ( 'NONE',  ( 12.38957946698288026, 79.72838755146472067, 129.9671884813441807 ) ) ;
#35569=DIRECTION ( 'NONE',  ( 0.000000000000000000, -1.000000000000000000, 0.000000000000000000 ) ) ;
#35573=LINE ( 'NONE', #84205, #75308 ) ;
#35588=ORIENTED_EDGE ( 'NONE', *, *, #72694, .F. ) ;
#35617=VECTOR ( 'NONE', #4318, 1000.000000000000000 ) ;
#35647=DIRECTION ( 'NONE',  ( -0.000000000000000000, -1.000000000000000000, -0.000000000000000000 ) ) ;
#35649=CARTESIAN_POINT ( 'NONE',  ( -117.1541088471463041, 73.49112389501519260, 57.63291976239248271 ) ) ;
#35678=CARTESIAN_POINT ( 'NONE',  ( -148.0533267522752112, 101.5999999999999943, 160.2664750769289697 ) ) ;
#35691=CYLINDRICAL_SURFACE ( 'NONE', #77109, 218.1859999999999786 ) ;
#35699=CARTESIAN_POINT ( 'NONE',  ( -185.9961463128564958, 20.32000000000000028, -3.174999999999349676 ) ) ;
#35727=CARTESIAN_POINT ( 'NONE',  ( -10.86025490963659301, 89.13458635777121231, 130.1035480231986980 ) ) ;
#35763=CARTESIAN_POINT ( 'NONE',  ( -109.8429120651473454, 48.03328757174836738, 70.56492720431617727 ) ) ;
#35777=CARTESIAN_POINT ( 'NONE',  ( 21.80448803080050979, 60.57658380354070715, 31.24433384097766719 ) ) ;
#35784=DIRECTION ( 'NONE',  ( 0.000000000000000000, 0.000000000000000000, -1.000000000000000000 ) ) ;
#35850=VERTEX_POINT ( 'NONE', #74296 ) ;
#35858=CYLINDRICAL_SURFACE ( 'NONE', #59320, 218.1859999999999786 ) ;
#35869=CARTESIAN_POINT ( 'NONE',  ( 120.5298512137159008, 47.23280909986927156, -50.17433177954229961 ) ) ;
#35897=B_SPLINE_CURVE_WITH_KNOTS ( 'NONE', 3,
 ( #45588, #18354, #86529, #38798, #45155, #66504, #4293, #3841, #87408, #43489, #77589, #31537, #59240, #31983, #25169, #52832, #15372, #80606, #46040, #73772, #43038, #70780, #26078, #5185, #46939, #67392, #74669, #48275, #12006, #32878, #75118, #39251, #12903, #82849 ),
 .UNSPECIFIED., .F., .F.,
 ( 4, 2, 2, 2, 2, 2, 2, 2, 2, 2, 2, 2, 2, 2, 2, 2, 4 ),
 ( 0.05204795639664543117, 0.05411398420652786811, 0.05618001201641030506, 0.06031206763617517896, 0.06237809544605762285, 0.06444412325594006674, 0.06857617887570495452, 0.07064220668558740535, 0.07270823449546987005, 0.07477426230535232088, 0.07580727621029356711, 0.07684029011523479946, 0.07890631792511729192, 0.08097234573499978438, 0.08303837354488227684, 0.08407138744982353695, 0.08510440135476479706 ),
 .UNSPECIFIED. ) ;
#35929=AXIS2_PLACEMENT_3D ( 'NONE', #50893, #39047, #4085 ) ;
#35964=PLANE ( 'NONE',  #38647 ) ;
#35973=DIRECTION ( 'NONE',  ( 0.000000000000000000, 0.000000000000000000, 1.000000000000000000 ) ) ;
#36023=DIRECTION ( 'NONE',  ( -1.000000000000000000, 0.000000000000000000, -0.000000000000000000 ) ) ;
#36027=FACE_OUTER_BOUND ( 'NONE', #20342, .T. ) ;
#36047=ORIENTED_EDGE ( 'NONE', *, *, #38105, .F. ) ;
#36058=AXIS2_PLACEMENT_3D ( 'NONE', #12110, #5300, #82517 ) ;
#36088=DIRECTION ( 'NONE',  ( -1.000000000000000000, 0.000000000000000000, 0.000000000000000000 ) ) ;
#36091=PLANE ( 'NONE',  #31510 ) ;
#36095=VECTOR ( 'NONE', #82612, 1000.000000000000114 ) ;
#36097=ORIENTED_EDGE ( 'NONE', *, *, #20866, .F. ) ;
#36180=VERTEX_POINT ( 'NONE', #42883 ) ;
#36192=ORIENTED_EDGE ( 'NONE', *, *, #51672, .T. ) ;
#36218=CIRCLE ( 'NONE', #44888, 179.8898777604655095 ) ;
#36229=PRODUCT ( 'Rotary Table Central Base', 'Rotary Table Central Base', '', ( #25868 ) ) ;
#36230=ORIENTED_EDGE ( 'NONE', *, *, #63006, .F. ) ;
#36239=CARTESIAN_POINT ( 'NONE',  ( 20.83015309964465800, 62.29495534028188786, 31.90425691968162170 ) ) ;
#36265=CIRCLE ( 'NONE', #68159, 179.8898777604655095 ) ;
#36266=ADVANCED_FACE ( 'NONE', ( #43336 ), #36091, .F. ) ;
#36354=CARTESIAN_POINT ( 'NONE',  ( -179.8898777604655095, 0.000000000000000000, 114.2999999999999972 ) ) ;
#36358=CARTESIAN_POINT ( 'NONE',  ( 124.7484337486687593, 70.55550032976780983, 38.50686379248426761 ) ) ;
#36360=ORIENTED_EDGE ( 'NONE', *, *, #15464, .T. ) ;
#36380=SURFACE_STYLE_FILL_AREA ( #7770 ) ;
#36415=EDGE_CURVE ( 'NONE', #16965, #79928, #4249, .T. ) ;
#36441=AXIS2_PLACEMENT_3D ( 'NONE', #50502, #24157, #8748 ) ;
#36461=EDGE_CURVE ( 'NONE', #7095, #65449, #17872, .T. ) ;
#36495=ORIENTED_EDGE ( 'NONE', *, *, #81168, .F. ) ;
#36506=ORIENTED_EDGE ( 'NONE', *, *, #17802, .F. ) ;
#36510=CARTESIAN_POINT ( 'NONE',  ( 4.773412683384191446, 94.31885047369215158, 130.4687102160306438 ) ) ;
#36514=CARTESIAN_POINT ( 'NONE',  ( 170.2205283966864897, 20.32000000000000028, 79.24800000000000466 ) ) ;
#36532=DIRECTION ( 'NONE',  ( 0.7071067811865835440, 0.000000000000000000, 0.7071067811865114905 ) ) ;
#36552=VERTEX_POINT ( 'NONE', #14 ) ;
#36597=DIRECTION ( 'NONE',  ( 0.000000000000000000, 1.000000000000000000, 0.000000000000000000 ) ) ;
#36604=CARTESIAN_POINT ( 'NONE',  ( 131.3179999999999836, 53.97500000000000142, 50.79999999999999716 ) ) ;
#36621=DIRECTION ( 'NONE',  ( 0.000000000000000000, -1.000000000000000000, 0.000000000000000000 ) ) ;
#36646=CARTESIAN_POINT ( 'NONE',  ( -11.76970797181927431, 87.32129802024908827, 130.0243965492825566 ) ) ;
#36649=ORIENTED_EDGE ( 'NONE', *, *, #82547, .F. ) ;
#36658=ORIENTED_EDGE ( 'NONE', *, *, #30569, .F. ) ;
#36675=ORIENTED_EDGE ( 'NONE', *, *, #43477, .T. ) ;
#36695=CARTESIAN_POINT ( 'NONE',  ( 23.09780390562728414, 56.38017385884855770, 30.30024197629754923 ) ) ;
#36704=ORIENTED_EDGE ( 'NONE', *, *, #6531, .T. ) ;
#36716=B_SPLINE_CURVE_WITH_KNOTS ( 'NONE', 3,
 ( #15309, #55695, #43427, #42975, #71174, #69369, #7143, #8947, #69819, #34838, #36646, #35277, #766, #56156, #83907, #49351, #70262, #8033, #35727, #78441, #45211, #50700, #24348, #38405, #86135, #30274, #65234, #3893, #87022, #37968, #59292, #72928, #57516, #66109, #23911, #58843, #3452, #79326, #23026, #44322, #17088, #30710, #16204, #72054, #9828, #2573, #78882, #51142, #16643, #29830, #44775, #79775, #31589, #85260, #80215, #10698, #10267, #24788, #43880, #31148, #51580 ),
 .UNSPECIFIED., .F., .F.,
 ( 4, 2, 2, 2, 1, 1, 1, 2, 2, 2, 2, 1, 1, 1, 1, 1, 2, 2, 2, 2, 2, 2, 2, 1, 1, 1, 1, 2, 2, 2, 2, 1, 1, 1, 2, 2, 2, 4 ),
 ( 0.000000000000000000, 0.1250000000003168854, 0.1875000000004742595, 0.2187500000005539458, 0.2343750000005937750, 0.2421875000006136758, 0.2460937500006236400, 0.2480468750006286638, 0.2500000000006336598, 0.3125000000007292500, 0.3437500000007759904, 0.3593750000008001932, 0.3671875000008131829, 0.3710937500008197332, 0.3730468750008228973, 0.3740234375008252288, 0.3745117187508265055, 0.3750000000008277823, 0.4375000000008258949, 0.5000000000008238965, 0.5625000000008220091, 0.5937500000008211209, 0.6093750000008205658, 0.6171875000008203438, 0.6210937500008208989, 0.6230468750008205658, 0.6240234375008203438, 0.6245117187508192336, 0.6250000000008181233, 0.6875000000006927792, 0.7187500000006302736, 0.7343750000005995204, 0.7421875000005839773, 0.7460937500005763168, 0.7480468750005724310, 0.7500000000005684342, 0.8750000000002843281, 1.000000000000000000 ),
 .UNSPECIFIED. ) ;
#36758=DIRECTION ( 'NONE',  ( 1.000000000000000000, 0.000000000000000000, 0.000000000000000000 ) ) ;
#36777=CARTESIAN_POINT ( 'NONE',  ( 125.3463460965257354, 52.19566713291690263, -36.51250000000000995 ) ) ;
#36798=LINE ( 'NONE', #71329, #25468 ) ;
#36804=CARTESIAN_POINT ( 'NONE',  ( 127.0239848601435995, 53.97500000000000142, 30.16249999999999787 ) ) ;
#36817=CARTESIAN_POINT ( 'NONE',  ( 0.000000000000000000, 0.000000000000000000, 0.000000000000000000 ) ) ;
#36826=CARTESIAN_POINT ( 'NONE',  ( 196.2150000000000034, 30.98800000000000310, 57.14999999999999858 ) ) ;
#36860=EDGE_LOOP ( 'NONE', ( #19395, #4442, #87100, #87382 ) ) ;
#36872=DIRECTION ( 'NONE',  ( 1.000000000000000000, 0.000000000000000000, 0.000000000000000000 ) ) ;
#36879=ADVANCED_FACE ( 'NONE', ( #60771 ), #60316, .T. ) ;
#36905=EDGE_CURVE ( 'NONE', #40524, #65725, #76197, .T. ) ;
#36938=VERTEX_POINT ( 'NONE', #20793 ) ;
#36946=DIRECTION ( 'NONE',  ( 0.000000000000000000, 0.000000000000000000, 1.000000000000000000 ) ) ;
#36972=EDGE_CURVE ( 'NONE', #40524, #71527, #82596, .T. ) ;
#36977=DIRECTION ( 'NONE',  ( 0.000000000000000000, -0.000000000000000000, -1.000000000000000000 ) ) ;
#36982=PLANE ( 'NONE',  #49436 ) ;
#37034=DIRECTION ( 'NONE',  ( -1.000000000000000000, 0.000000000000000000, 0.000000000000000000 ) ) ;
#37049=CARTESIAN_POINT ( 'NONE',  ( -178.3658777604659917, 101.5999999999999943, 122.9960808104842016 ) ) ;
#37076=APPLICATION_CONTEXT ( 'automotive_design' ) ;
#37084=CARTESIAN_POINT ( 'NONE',  ( 160.2664750769284865, 20.32000000000000028, -148.0533267522753818 ) ) ;
#37101=ORIENTED_EDGE ( 'NONE', *, *, #27435, .F. ) ;
#37123=CARTESIAN_POINT ( 'NONE',  ( 173.9900000000000091, 21.46300000000000097, 59.96543552338529537 ) ) ;
#37138=CARTESIAN_POINT ( 'NONE',  ( 9.506033823739755917, 69.25266161161103184, 36.92015570084876686 ) ) ;
#37139=VECTOR ( 'NONE', #4196, 1000.000000000000000 ) ;
#37147=ORIENTED_EDGE ( 'NONE', *, *, #64870, .T. ) ;
#37158=CARTESIAN_POINT ( 'NONE',  ( -3.174999999999664979, 8.255000000000000782, 31.75000000000000000 ) ) ;
#37159=DIRECTION ( 'NONE',  ( -2.108231265501709878E-16, 0.000000000000000000, 1.000000000000000000 ) ) ;
#37173=DIRECTION ( 'NONE',  ( 0.000000000000000000, 0.000000000000000000, -1.000000000000000000 ) ) ;
#37185=EDGE_CURVE ( 'NONE', #66356, #4943, #38565, .T. ) ;
#37221=ORIENTED_EDGE ( 'NONE', *, *, #17193, .F. ) ;
#37232=ORIENTED_EDGE ( 'NONE', *, *, #52435, .T. ) ;
#37250=DIRECTION ( 'NONE',  ( -2.761895400282000234E-15, 0.000000000000000000, -1.000000000000000000 ) ) ;
#37273=ORIENTED_EDGE ( 'NONE', *, *, #75188, .T. ) ;
#37299=ORIENTED_EDGE ( 'NONE', *, *, #39113, .F. ) ;
#37374=EDGE_CURVE ( 'NONE', #31479, #64725, #64793, .T. ) ;
#37375=CARTESIAN_POINT ( 'NONE',  ( 0.000000000000000000, 20.32000000000000028, 0.000000000000000000 ) ) ;
#37395=CARTESIAN_POINT ( 'NONE',  ( 148.0533267522752112, 20.32000000000000028, 160.2664750769284865 ) ) ;
#37402=DIRECTION ( 'NONE',  ( 1.000000000000000000, 0.000000000000000000, 0.000000000000000000 ) ) ;
#37432=FACE_OUTER_BOUND ( 'NONE', #1603, .T. ) ;
#37434=CARTESIAN_POINT ( 'NONE',  ( 50.03799999999999670, 101.5999999999999943, 206.3750000000000000 ) ) ;
#37465=EDGE_LOOP ( 'NONE', ( #67342, #28091 ) ) ;
#37506=AXIS2_PLACEMENT_3D ( 'NONE', #17712, #44054, #9558 ) ;
#37551=EDGE_LOOP ( 'NONE', ( #56724, #49891, #22599, #72919 ) ) ;
#37554=CYLINDRICAL_SURFACE ( 'NONE', #42337, 7.874000000000186184 ) ;
#37561=ORIENTED_EDGE ( 'NONE', *, *, #52564, .T. ) ;
#37587=DIRECTION ( 'NONE',  ( -0.000000000000000000, 1.000000000000000000, 0.000000000000000000 ) ) ;
#37702=CARTESIAN_POINT ( 'NONE',  ( 121.3880544210665988, 74.44113218321618319, 48.06552997551920470 ) ) ;
#37716=EDGE_LOOP ( 'NONE', ( #22758, #23385, #70623, #49576 ) ) ;
#37727=ORIENTED_EDGE ( 'NONE', *, *, #26301, .T. ) ;
#37741=VERTEX_POINT ( 'NONE', #23134 ) ;
#37746=VECTOR ( 'NONE', #15050, 1000.000000000000114 ) ;
#37763=ORIENTED_EDGE ( 'NONE', *, *, #27973, .T. ) ;
#37767=FILL_AREA_STYLE_COLOUR ( '', #40131 ) ;
#37787=ORIENTED_EDGE ( 'NONE', *, *, #36415, .T. ) ;
#37804=ORIENTED_EDGE ( 'NONE', *, *, #27560, .T. ) ;
#37811=CARTESIAN_POINT ( 'NONE',  ( 1.166476076187854022E-15, 12.27000000000000313, 9.525000000000000355 ) ) ;
#37822=DIRECTION ( 'NONE',  ( 2.761895400282000234E-15, 0.000000000000000000, 1.000000000000000000 ) ) ;
#37825=VECTOR ( 'NONE', #26824, 1000.000000000000000 ) ;
#37826=EDGE_CURVE ( 'NONE', #18319, #14989, #12656, .T. ) ;
#37842=CARTESIAN_POINT ( 'NONE',  ( 6.884321588596717945, 93.22247119488908140, 130.3743772813626549 ) ) ;
#37884=ORIENTED_EDGE ( 'NONE', *, *, #74918, .T. ) ;
#37887=LINE ( 'NONE', #58752, #1384 ) ;
#37889=AXIS2_PLACEMENT_3D ( 'NONE', #40808, #82627, #81727 ) ;
#37903=VECTOR ( 'NONE', #82768, 1000.000000000000000 ) ;
#37956=ORIENTED_EDGE ( 'NONE', *, *, #20202, .F. ) ;
#37958=ORIENTED_EDGE ( 'NONE', *, *, #84883, .F. ) ;
#37968=CARTESIAN_POINT ( 'NONE',  ( -9.690133600363056487, 90.76968238247971499, 130.1963199222103356 ) ) ;
#37990=EDGE_CURVE ( 'NONE', #7552, #66356, #45934, .T. ) ;
#38019=ORIENTED_EDGE ( 'NONE', *, *, #47452, .F. ) ;
#38048=VECTOR ( 'NONE', #24866, 1000.000000000000000 ) ;
#38073=VECTOR ( 'NONE', #71125, 1000.000000000000000 ) ;
#38080=LINE ( 'NONE', #65772, #27807 ) ;
#38105=EDGE_CURVE ( 'NONE', #12226, #84394, #10303, .T. ) ;
#38130=CARTESIAN_POINT ( 'NONE',  ( 173.9900000000000091, 52.73749999999999716, -52.38749999999999574 ) ) ;
#38136=CARTESIAN_POINT ( 'NONE',  ( 109.6076600728624015, 58.52556248408083661, 70.92975744315074849 ) ) ;
#38227=ORIENTED_EDGE ( 'NONE', *, *, #15110, .T. ) ;
#38253=VECTOR ( 'NONE', #26834, 1000.000000000000000 ) ;
#38283=DIRECTION ( 'NONE',  ( 1.000000000000000000, 0.000000000000000000, 0.000000000000000000 ) ) ;
#38284=FACE_BOUND ( 'NONE', #45352, .T. ) ;
#38298=DIRECTION ( 'NONE',  ( 0.000000000000000000, -1.000000000000000000, 0.000000000000000000 ) ) ;
#38309=PLANE ( 'NONE',  #54030 ) ;
#38344=ORIENTED_EDGE ( 'NONE', *, *, #72118, .F. ) ;
#38360=CARTESIAN_POINT ( 'NONE',  ( -3.175000000000120171, 24.56180297284579694, -33.98325472291460159 ) ) ;
#38390=ORIENTED_EDGE ( 'NONE', *, *, #15110, .F. ) ;
#38405=CARTESIAN_POINT ( 'NONE',  ( -10.57225270112366822, 89.58687159901970176, 130.1272325585186991 ) ) ;
#38412=CARTESIAN_POINT ( 'NONE',  ( 127.0239848601436279, 53.14682735907139488, 30.16250000000001563 ) ) ;
#38429=CARTESIAN_POINT ( 'NONE',  ( -111.5664126600051418, 65.66542280838000067, 67.80711950243038189 ) ) ;
#38441=ORIENTED_EDGE ( 'NONE', *, *, #81037, .F. ) ;
#38447=ORIENTED_EDGE ( 'NONE', *, *, #84885, .T. ) ;
#38454=DIRECTION ( 'NONE',  ( 1.000000000000000000, 0.000000000000000000, 7.867884063170659983E-16 ) ) ;
#38469=AXIS2_PLACEMENT_3D ( 'NONE', #69007, #55349, #27670 ) ;
#38479=PLANE ( 'NONE',  #67450 ) ;
#38482=ADVANCED_FACE ( 'NONE', ( #11426 ), #67733, .F. ) ;
#38500=CARTESIAN_POINT ( 'NONE',  ( 33.98325472291465132, 24.56180297284579694, 3.174999999999999822 ) ) ;
#38504=CARTESIAN_POINT ( 'NONE',  ( 0.000000000000000000, 17.78000000000000114, 0.000000000000000000 ) ) ;
#38515=VECTOR ( 'NONE', #53110, 1000.000000000000000 ) ;
#38518=CARTESIAN_POINT ( 'NONE',  ( -127.5252020268932114, 0.000000000000000000, 177.0380000000000109 ) ) ;
#38522=AXIS2_PLACEMENT_3D ( 'NONE', #61497, #76031, #82872 ) ;
#38526=CARTESIAN_POINT ( 'NONE',  ( 125.3463460965257070, 52.73749999999999716, -36.51249999999992468 ) ) ;
#38565=B_SPLINE_CURVE_WITH_KNOTS ( 'NONE', 3,
 ( #67935, #26594, #54273, #4376, #4818, #5720, #82038, #46123, #38878, #19788, #32064, #73850, #80237, #32961, #60656, #81591, #39330, #10724, #52913, #53378, #11173, #19342, #47017, #17988, #80682, #12528, #38429, #70174, #41111, #6169, #21595, #33857, #7950, #28850, #34755, #82488, #47915, #681, #13426, #7061, #27053, #27938, #14329, #20242, #75657, #7507, #77001, #35649, #83822, #234, #55166, #56533, #27491, #83367, #68837, #21139, #49267, #63361, #22052, #69287, #28386, #75203, #6605, #34301, #48810, #61553, #12984, #40671, #14784, #42006, #76546, #76092, #69737, #89289, #62902, #84279, #13869, #56072, #62460, #62009, #68392, #35191, #42449, #1144, #41549, #54725, #89744, #55614, #82929, #20688, #48356, #84728, #71978, #51498, #72421, #58331, #64710, #29749, #31065, #2041, #57887, #85620, #23828, #10186 ),
 .UNSPECIFIED., .F., .F.,
 ( 4, 2, 1, 1, 2, 2, 2, 1, 1, 1, 2, 2, 2, 1, 1, 1, 2, 2, 2, 1, 1, 2, 2, 2, 1, 1, 2, 2, 2, 2, 2, 1, 1, 1, 2, 2, 1, 1, 2, 2, 2, 1, 1, 2, 2, 2, 1, 2, 2, 2, 1, 2, 2, 2, 1, 2, 2, 2, 2, 2, 2, 2, 4 ),
 ( 0.000000000000000000, 0.03124999999999297784, 0.04687499999998949451, 0.05468749999998755856, 0.05859374999998673977, 0.06249999999998591405, 0.09374999999997923883, 0.1093749999999759082, 0.1171874999999741596, 0.1210937499999732714, 0.1230468749999728273, 0.1249999999999723832, 0.1562499999999672207, 0.1718749999999646949, 0.1796874999999637790, 0.1835937499999631961, 0.1855468749999625577, 0.1874999999999619194, 0.2187499999999570899, 0.2343749999999545641, 0.2421874999999530931, 0.2460937499999527045, 0.2499999999999522604, 0.2812499999999505396, 0.2968749999999500400, 0.3046874999999500400, 0.3085937499999499845, 0.3124999999999499289, 0.3437499999999493738, 0.3749999999999488742, 0.4374999999999475975, 0.4687499999999467648, 0.4843749999999463207, 0.4921874999999461542, 0.4960937499999459876, 0.4999999999999458211, 0.5312499999999467093, 0.5468749999999470424, 0.5546874999999472644, 0.5624999999999474865, 0.5937499999999481526, 0.6093749999999482636, 0.6171874999999482636, 0.6210937499999483746, 0.6249999999999484857, 0.6562499999999525935, 0.6718749999999547029, 0.6796874999999555911, 0.6874999999999564793, 0.7187499999999598099, 0.7343749999999615863, 0.7421874999999624745, 0.7499999999999633626, 0.7812499999999671374, 0.7968749999999690248, 0.8046874999999700240, 0.8124999999999710232, 0.8437499999999762412, 0.8749999999999814593, 0.9062499999999863443, 0.9218749999999886757, 0.9374999999999910072, 1.000000000000000000 ),
 .UNSPECIFIED. ) ;
#38566=DIRECTION ( 'NONE',  ( 0.000000000000000000, -1.000000000000000000, 0.000000000000000000 ) ) ;
#38571=CARTESIAN_POINT ( 'NONE',  ( 116.2447374730602547, 72.73035545477121389, 59.43458213646708543 ) ) ;
#38579=VERTEX_POINT ( 'NONE', #20041 ) ;
#38584=VECTOR ( 'NONE', #10173, 1000.000000000000114 ) ;
#38585=DIRECTION ( 'NONE',  ( 0.000000000000000000, 1.000000000000000000, 0.000000000000000000 ) ) ;
#38606=DIRECTION ( 'NONE',  ( 0.000000000000000000, -0.9961946980917455452, -0.08715574274765836016 ) ) ;
#38624=CARTESIAN_POINT ( 'NONE',  ( -160.2664750769294812, 20.32000000000000028, -148.0533267522755807 ) ) ;
#38647=AXIS2_PLACEMENT_3D ( 'NONE', #41858, #62767, #62321 ) ;
#38648=DIRECTION ( 'NONE',  ( 0.000000000000000000, 0.000000000000000000, 1.000000000000000000 ) ) ;
#38694=ADVANCED_FACE ( 'NONE', ( #21839 ), #12781, .F. ) ;
#38700=EDGE_CURVE ( 'NONE', #71527, #28720, #22284, .T. ) ;
#38717=CARTESIAN_POINT ( 'NONE',  ( 11.53693603528213529, 87.86025992443330779, 130.0452829984675134 ) ) ;
#38775=PLANE ( 'NONE',  #66215 ) ;
#38777=ORIENTED_EDGE ( 'NONE', *, *, #36905, .F. ) ;
#38787=ORIENTED_EDGE ( 'NONE', *, *, #32415, .F. ) ;
#38798=CARTESIAN_POINT ( 'NONE',  ( -2.767668950682794282, 70.16797056649836861, 38.00561040827691528 ) ) ;
#38814=VERTEX_POINT ( 'NONE', #29093 ) ;
#38823=CARTESIAN_POINT ( 'NONE',  ( 173.9900000000000091, 53.21300000000000097, 59.96543552338529537 ) ) ;
#38824=DIRECTION ( 'NONE',  ( 0.000000000000000000, 1.000000000000000000, 0.000000000000000000 ) ) ;
#38843=CIRCLE ( 'NONE', #62064, 130.5560000000000116 ) ;
#38870=ORIENTED_EDGE ( 'NONE', *, *, #32706, .F. ) ;
#38874=CARTESIAN_POINT ( 'NONE',  ( 173.9900000000000091, 37.33800000000000097, 42.86249999999999716 ) ) ;
#38878=CARTESIAN_POINT ( 'NONE',  ( -109.5466416834841539, 58.08661539045247935, 71.02395987518927711 ) ) ;
#38892=CARTESIAN_POINT ( 'NONE',  ( -215.9000000000000057, 101.5999999999999943, -45.33899999999999864 ) ) ;
#38934=VERTEX_POINT ( 'NONE', #67169 ) ;
#38951=DIRECTION ( 'NONE',  ( 0.000000000000000000, 0.000000000000000000, 1.000000000000000000 ) ) ;
#38953=DIRECTION ( 'NONE',  ( 8.503806984168930281E-16, 0.000000000000000000, -1.000000000000000000 ) ) ;
#38961=LINE ( 'NONE', #3554, #30312 ) ;
#38975=CARTESIAN_POINT ( 'NONE',  ( 122.9150858762449587, 60.67894162041066153, -44.01180387395123006 ) ) ;
#39004=ADVANCED_FACE ( 'NONE', ( #19927 ), #13120, .T. ) ;
#39018=CARTESIAN_POINT ( 'NONE',  ( 110.3758871135606796, 62.19865536329562872, 69.72828050043732162 ) ) ;
#39041=DIRECTION ( 'NONE',  ( 0.000000000000000000, 0.000000000000000000, -1.000000000000000000 ) ) ;
#39047=DIRECTION ( 'NONE',  ( 0.000000000000000000, 1.000000000000000000, 0.000000000000000000 ) ) ;
#39052=AXIS2_PLACEMENT_3D ( 'NONE', #72457, #10658, #51537 ) ;
#39071=VECTOR ( 'NONE', #70715, 1000.000000000000000 ) ;
#39078=ORIENTED_EDGE ( 'NONE', *, *, #13451, .T. ) ;
#39106=DIRECTION ( 'NONE',  ( 0.000000000000000000, 0.000000000000000000, 1.000000000000000000 ) ) ;
#39113=EDGE_CURVE ( 'NONE', #31056, #19557, #82622, .T. ) ;
#39115=FACE_OUTER_BOUND ( 'NONE', #80893, .T. ) ;
#39119=EDGE_CURVE ( 'NONE', #66356, #60724, #26286, .T. ) ;
#39127=CARTESIAN_POINT ( 'NONE',  ( -57.91199999999999903, 20.32000000000000028, 178.6098374884404905 ) ) ;
#39135=EDGE_CURVE ( 'NONE', #64336, #19304, #57567, .T. ) ;
#39161=ADVANCED_FACE ( 'NONE', ( #2625 ), #15364, .T. ) ;
#39171=CARTESIAN_POINT ( 'NONE',  ( 11.41096683840008552, 88.12842719786394241, 130.0564362339166280 ) ) ;
#39178=DIRECTION ( 'NONE',  ( 0.000000000000000000, 1.000000000000000000, 0.000000000000000000 ) ) ;
#39187=DIRECTION ( 'NONE',  ( 0.000000000000000000, -1.000000000000000000, 0.000000000000000000 ) ) ;
#39190=AXIS2_PLACEMENT_3D ( 'NONE', #35678, #57010, #84752 ) ;
#39194=FACE_OUTER_BOUND ( 'NONE', #12740, .T. ) ;
#39211=ORIENTED_EDGE ( 'NONE', *, *, #13693, .F. ) ;
#39246=CARTESIAN_POINT ( 'NONE',  ( 1.154229608196380665E-15, 152.3879256507328250, 9.425000000000000711 ) ) ;
#39251=CARTESIAN_POINT ( 'NONE',  ( -23.26572343534745357, 54.67490044792280202, 30.17145907252543324 ) ) ;
#39258=CIRCLE ( 'NONE', #7362, 9.425000000000000711 ) ;
#39279=ORIENTED_EDGE ( 'NONE', *, *, #14863, .T. ) ;
#39282=DIRECTION ( 'NONE',  ( 0.000000000000000000, -1.000000000000000000, 0.000000000000000000 ) ) ;
#39291=DIRECTION ( 'NONE',  ( 0.000000000000000000, 0.000000000000000000, 1.000000000000000000 ) ) ;
#39296=AXIS2_PLACEMENT_3D ( 'NONE', #11789, #80843, #53073 ) ;
#39312=DIRECTION ( 'NONE',  ( 0.000000000000000000, 0.000000000000000000, -1.000000000000000000 ) ) ;
#39324=DIRECTION ( 'NONE',  ( 0.000000000000000000, 0.000000000000000000, -1.000000000000000000 ) ) ;
#39330=CARTESIAN_POINT ( 'NONE',  ( -110.3398647909624515, 62.06622433141639306, 69.78526909086103558 ) ) ;
#39346=DIRECTION ( 'NONE',  ( 0.000000000000000000, -1.000000000000000000, 0.000000000000000000 ) ) ;
#39353=CARTESIAN_POINT ( 'NONE',  ( 3.175000000000334666, 24.56180297284579694, 31.75000000000000000 ) ) ;
#39366=LINE ( 'NONE', #61586, #46617 ) ;
#39376=ORIENTED_EDGE ( 'NONE', *, *, #27435, .T. ) ;
#39386=ORIENTED_EDGE ( 'NONE', *, *, #29878, .F. ) ;
#39420=FACE_BOUND ( 'NONE', #11657, .T. ) ;
#39424=ORIENTED_EDGE ( 'NONE', *, *, #65582, .F. ) ;
#39426=CARTESIAN_POINT ( 'NONE',  ( 120.0660739680716915, 56.80016398518806398, -51.27402828685031011 ) ) ;
#39456=ORIENTED_EDGE ( 'NONE', *, *, #71437, .F. ) ;
#39469=DIRECTION ( 'NONE',  ( 0.000000000000000000, 1.000000000000000000, 0.000000000000000000 ) ) ;
#39471=CARTESIAN_POINT ( 'NONE',  ( 113.1543859615763949, 68.83350072574626211, 65.12264306354134646 ) ) ;
#39513=ORIENTED_EDGE ( 'NONE', *, *, #42504, .T. ) ;
#39541=DIRECTION ( 'NONE',  ( 0.000000000000000000, 0.000000000000000000, 1.000000000000000000 ) ) ;
#39542=CARTESIAN_POINT ( 'NONE',  ( 135.2444258376725941, 0.000000000000000000, 147.4575741623265799 ) ) ;
#39550=ORIENTED_EDGE ( 'NONE', *, *, #75766, .T. ) ;
#39609=CARTESIAN_POINT ( 'NONE',  ( 10.53542287845765557, 89.64189664627865284, 130.1302201369519196 ) ) ;
#39610=ORIENTED_EDGE ( 'NONE', *, *, #14332, .F. ) ;
#39621=EDGE_LOOP ( 'NONE', ( #33, #7799, #1855, #33813 ) ) ;
#39645=DIRECTION ( 'NONE',  ( -6.982966722218760189E-15, 0.000000000000000000, -1.000000000000000000 ) ) ;
#39658=EDGE_CURVE ( 'NONE', #77506, #51500, #31140, .T. ) ;
#39686=VERTEX_POINT ( 'NONE', #57464 ) ;
#39715=ORIENTED_EDGE ( 'NONE', *, *, #47910, .F. ) ;
#39733=VECTOR ( 'NONE', #57017, 1000.000000000000000 ) ;
#39746=EDGE_CURVE ( 'NONE', #84162, #5960, #9374, .T. ) ;
#39750=DIRECTION ( 'NONE',  ( 1.000000000000000000, 0.000000000000000000, 0.000000000000000000 ) ) ;
#39771=ORIENTED_EDGE ( 'NONE', *, *, #37374, .T. ) ;
#39804=EDGE_LOOP ( 'NONE', ( #86618, #33401 ) ) ;
#39820=VERTEX_POINT ( 'NONE', #83849 ) ;
#39859=CARTESIAN_POINT ( 'NONE',  ( 163.0822201311030142, 20.32000000000000028, -75.92468371870729982 ) ) ;
#39863=CARTESIAN_POINT ( 'NONE',  ( 121.9913672821676869, 60.41918071833632098, -46.51076114057810429 ) ) ;
#39871=EDGE_CURVE ( 'NONE', #56606, #23728, #2957, .T. ) ;
#39875=CARTESIAN_POINT ( 'NONE',  ( 0.000000000000000000, 44.45000000000000284, 0.000000000000000000 ) ) ;
#39877=ORIENTED_EDGE ( 'NONE', *, *, #52302, .F. ) ;
#39893=DIRECTION ( 'NONE',  ( 0.000000000000000000, -1.000000000000000000, 0.000000000000000000 ) ) ;
#39901=DIRECTION ( 'NONE',  ( 0.000000000000000000, 0.000000000000000000, 1.000000000000000000 ) ) ;
#39913=DIRECTION ( 'NONE',  ( -1.000000000000000000, 0.000000000000000000, 0.000000000000000000 ) ) ;
#40008=ORIENTED_EDGE ( 'NONE', *, *, #82573, .F. ) ;
#40023=ORIENTED_EDGE ( 'NONE', *, *, #67638, .T. ) ;
#40069=ORIENTED_EDGE ( 'NONE', *, *, #59086, .T. ) ;
#40082=DIRECTION ( 'NONE',  ( 0.000000000000000000, 0.000000000000000000, 1.000000000000000000 ) ) ;
#40085=DIRECTION ( 'NONE',  ( 3.491483361109380094E-15, 0.000000000000000000, 1.000000000000000000 ) ) ;
#40092=CIRCLE ( 'NONE', #53159, 9.525000000000000355 ) ;
#40094=EDGE_LOOP ( 'NONE', ( #10311, #20643, #24562, #13144, #88383, #28469 ) ) ;
#40110=ORIENTED_EDGE ( 'NONE', *, *, #69602, .T. ) ;
#40111=ORIENTED_EDGE ( 'NONE', *, *, #75212, .F. ) ;
#40126=ORIENTED_EDGE ( 'NONE', *, *, #41869, .F. ) ;
#40131=COLOUR_RGB ( '', 0.72549020, 0.75294118, 0.79215686) ;
#40164=CARTESIAN_POINT ( 'NONE',  ( 23.18381393575008786, 52.19607888965136056, 30.23446726999232226 ) ) ;
#40192=AXIS2_PLACEMENT_3D ( 'NONE', #22098, #89338, #49763 ) ;
#40236=ADVANCED_FACE ( 'NONE', ( #55535, #63282 ), #1058, .T. ) ;
#40255=DIRECTION ( 'NONE',  ( 0.000000000000000000, 0.000000000000000000, -1.000000000000000000 ) ) ;
#40281=CARTESIAN_POINT ( 'NONE',  ( -127.0122462326317958, 52.31737473627642743, 30.21206415535068146 ) ) ;
#40289=CARTESIAN_POINT ( 'NONE',  ( 0.000000000000000000, 20.32000000000000028, 0.000000000000000000 ) ) ;
#40291=AXIS2_PLACEMENT_3D ( 'NONE', #20711, #68417, #67062 ) ;
#40377=ORIENTED_EDGE ( 'NONE', *, *, #69515, .T. ) ;
#40411=LINE ( 'NONE', #45858, #47079 ) ;
#40441=ORIENTED_EDGE ( 'NONE', *, *, #2533, .F. ) ;
#40446=ADVANCED_FACE ( 'NONE', ( #83516 ), #42159, .F. ) ;
#40473=CARTESIAN_POINT ( 'NONE',  ( 141.3509999999999991, 101.5999999999999943, 141.3509999999999991 ) ) ;
#40483=ORIENTED_EDGE ( 'NONE', *, *, #78002, .T. ) ;
#40495=CARTESIAN_POINT ( 'NONE',  ( 196.2150000000000034, 30.98800000000000310, 57.14999999999999858 ) ) ;
#40497=VERTEX_POINT ( 'NONE', #82191 ) ;
#40512=CARTESIAN_POINT ( 'NONE',  ( 10.07149677053134162, 90.28936803021488799, 130.1671656890560200 ) ) ;
#40523=ORIENTED_EDGE ( 'NONE', *, *, #89079, .F. ) ;
#40524=VERTEX_POINT ( 'NONE', #28532 ) ;
#40527=VECTOR ( 'NONE', #7501, 1000.000000000000000 ) ;
#40552=EDGE_CURVE ( 'NONE', #84701, #86605, #57560, .T. ) ;
#40564=ADVANCED_FACE ( 'NONE', ( #3088, #9901 ), #79402, .T. ) ;
#40573=DIRECTION ( 'NONE',  ( 0.000000000000000000, 1.000000000000000000, 0.000000000000000000 ) ) ;
#40597=DIRECTION ( 'NONE',  ( 0.000000000000000000, -1.000000000000000000, 0.000000000000000000 ) ) ;
#40626=DIRECTION ( 'NONE',  ( -6.982966722218760189E-15, 0.000000000000000000, -1.000000000000000000 ) ) ;
#40633=ORIENTED_EDGE ( 'NONE', *, *, #85204, .F. ) ;
#40635=ORIENTED_EDGE ( 'NONE', *, *, #28135, .F. ) ;
#40649=EDGE_LOOP ( 'NONE', ( #67582, #30079 ) ) ;
#40671=CARTESIAN_POINT ( 'NONE',  ( -122.9597727627798918, 73.41921189914249624, 43.88359923157533871 ) ) ;
#40690=ORIENTED_EDGE ( 'NONE', *, *, #79360, .F. ) ;
#40697=CARTESIAN_POINT ( 'NONE',  ( -6.304597144436756118, 71.52322690941528549, 130.4037788038045846 ) ) ;
#40712=ORIENTED_EDGE ( 'NONE', *, *, #20798, .F. ) ;
#40721=DIRECTION ( 'NONE',  ( 1.000000000000000000, 0.000000000000000000, 2.108231265501709878E-16 ) ) ;
#40765=ORIENTED_EDGE ( 'NONE', *, *, #58407, .T. ) ;
#40808=CARTESIAN_POINT ( 'NONE',  ( 0.000000000000000000, 20.32000000000000028, 0.000000000000000000 ) ) ;
#40828=ORIENTED_EDGE ( 'NONE', *, *, #20945, .T. ) ;
#40889=ORIENTED_EDGE ( 'NONE', *, *, #18028, .T. ) ;
#40915=AXIS2_PLACEMENT_3D ( 'NONE', #42931, #2074, #15708 ) ;
#40924=DIRECTION ( 'NONE',  ( 0.000000000000000000, -3.785359618865284342E-16, -1.000000000000000000 ) ) ;
#40965=LINE ( 'NONE', #56379, #23953 ) ;
#40971=CIRCLE ( 'NONE', #65675, 7.873999999999991672 ) ;
#40977=CIRCLE ( 'NONE', #33787, 34.13125000000000142 ) ;
#40992=ORIENTED_EDGE ( 'NONE', *, *, #75188, .F. ) ;
#41040=CARTESIAN_POINT ( 'NONE',  ( 141.3509999999999991, 20.32000000000000028, -141.3509999999999991 ) ) ;
#41104=EDGE_LOOP ( 'NONE', ( #39386, #77889, #13782, #52861 ) ) ;
#41111=CARTESIAN_POINT ( 'NONE',  ( -112.0489691580589096, 66.76700720547121648, 67.00851989138369902 ) ) ;
#41120=AXIS2_PLACEMENT_3D ( 'NONE', #13713, #68236, #6019 ) ;
#41137=CARTESIAN_POINT ( 'NONE',  ( -4.809187206306169138, 70.79577073431487122, 130.4673938299285396 ) ) ;
#41138=CARTESIAN_POINT ( 'NONE',  ( -57.91199999999999903, 20.32000000000000028, 191.3008000794699797 ) ) ;
#41188=FACE_OUTER_BOUND ( 'NONE', #50975, .T. ) ;
#41229=CARTESIAN_POINT ( 'NONE',  ( 0.000000000000000000, 12.27000000000000313, -9.425000000000000711 ) ) ;
#41306=DIRECTION ( 'NONE',  ( 1.047445008332813989E-14, 0.000000000000000000, 1.000000000000000000 ) ) ;
#41318=CARTESIAN_POINT ( 'NONE',  ( 5.165685852724023697, 70.94733280150917665, 130.4538059770566747 ) ) ;
#41333=DIRECTION ( 'NONE',  ( 0.000000000000000000, -1.000000000000000000, 0.000000000000000000 ) ) ;
#41340=ORIENTED_EDGE ( 'NONE', *, *, #85346, .T. ) ;
#41363=LINE ( 'NONE', #5070, #12531 ) ;
#41377=ORIENTED_EDGE ( 'NONE', *, *, #58143, .F. ) ;
#41378=CIRCLE ( 'NONE', #87759, 218.1859999999999786 ) ;
#41384=EDGE_LOOP ( 'NONE', ( #77401, #71836, #47655, #7701 ) ) ;
#41386=CARTESIAN_POINT ( 'NONE',  ( 71.09939861440099662, 20.32000000000000028, 177.8662485265279827 ) ) ;
#41387=DIRECTION ( 'NONE',  ( 0.000000000000000000, 0.000000000000000000, 1.000000000000000000 ) ) ;
#41413=CARTESIAN_POINT ( 'NONE',  ( -23.27731929905162289, 53.97500000000000142, 30.16249999999999076 ) ) ;
#41424=CARTESIAN_POINT ( 'NONE',  ( 0.000000000000000000, 8.255000000000000782, 0.000000000000000000 ) ) ;
#41493=DIRECTION ( 'NONE',  ( 0.000000000000000000, -1.000000000000000000, 0.000000000000000000 ) ) ;
#41500=CARTESIAN_POINT ( 'NONE',  ( 71.09939861440099662, 101.5999999999999943, 177.8662485265279827 ) ) ;
#41522=CARTESIAN_POINT ( 'NONE',  ( 75.61066417432020614, 0.000000000000000000, 189.7379999999999995 ) ) ;
#41543=ORIENTED_EDGE ( 'NONE', *, *, #17193, .T. ) ;
#41549=CARTESIAN_POINT ( 'NONE',  ( -125.4478282125672877, 68.54351064866861520, 36.16615773164556913 ) ) ;
#41572=ADVANCED_FACE ( 'NONE', ( #75439 ), #13651, .F. ) ;
#41579=CARTESIAN_POINT ( 'NONE',  ( -7.053076781563553332, 71.98855499260324109, 130.3653452852127828 ) ) ;
#41595=CARTESIAN_POINT ( 'NONE',  ( -185.9961463128564958, 20.32000000000000028, -3.174999999999349676 ) ) ;
#41602=DIRECTION ( 'NONE',  ( 1.000000000000000000, 0.000000000000000000, -3.491483361109380094E-15 ) ) ;
#41641=CIRCLE ( 'NONE', #19951, 218.1859999999999786 ) ;
#41646=ORIENTED_EDGE ( 'NONE', *, *, #65376, .F. ) ;
#41678=AXIS2_PLACEMENT_3D ( 'NONE', #6428, #20522, #62281 ) ;
#41690=FACE_OUTER_BOUND ( 'NONE', #22779, .T. ) ;
#41696=CARTESIAN_POINT ( 'NONE',  ( 109.5221484136284005, 50.04810782126799751, 71.06173480727821357 ) ) ;
#41727=AXIS2_PLACEMENT_3D ( 'NONE', #34073, #41333, #62238 ) ;
#41729=CARTESIAN_POINT ( 'NONE',  ( 33.98325472291465132, 17.78000000000000114, -3.174999999999999822 ) ) ;
#41730=DIRECTION ( 'NONE',  ( -0.7071067811865621167, 0.000000000000000000, 0.7071067811865330288 ) ) ;
#41731=EDGE_CURVE ( 'NONE', #57559, #39820, #79509, .T. ) ;
#41753=ORIENTED_EDGE ( 'NONE', *, *, #32955, .T. ) ;
#41765=CARTESIAN_POINT ( 'NONE',  ( 1.925672578516905147E-22, 69.84999999999999432, 130.5560000000000116 ) ) ;
#41787=CIRCLE ( 'NONE', #20029, 25.39999999999999858 ) ;
#41806=EDGE_LOOP ( 'NONE', ( #73183, #37147, #67728, #87270, #72186, #78367 ) ) ;
#41840=DIRECTION ( 'NONE',  ( -1.000000000000000000, -8.741913579725640327E-16, -1.514143847546115117E-15 ) ) ;
#41858=CARTESIAN_POINT ( 'NONE',  ( -148.0533267522759786, 101.5999999999999943, -160.2664750769289697 ) ) ;
#41869=EDGE_CURVE ( 'NONE', #58184, #77506, #32631, .T. ) ;
#41891=ORIENTED_EDGE ( 'NONE', *, *, #26429, .T. ) ;
#41920=CARTESIAN_POINT ( 'NONE',  ( 10.66920567967061650, 75.66061691139891821, 130.1193289296744524 ) ) ;
#41925=CARTESIAN_POINT ( 'NONE',  ( 141.3509999999999991, 0.000000000000000000, 132.7150000000000034 ) ) ;
#41931=VERTEX_POINT ( 'NONE', #17070 ) ;
#41961=EDGE_LOOP ( 'NONE', ( #32188, #33794, #89054, #66461, #38441, #2550 ) ) ;
#41966=CARTESIAN_POINT ( 'NONE',  ( 0.000000000000000000, 44.45000000000000284, 0.000000000000000000 ) ) ;
#42006=CARTESIAN_POINT ( 'NONE',  ( -123.0424546654431452, 73.33497890737675107, 43.65123806753916114 ) ) ;
#42051=LINE ( 'NONE', #43392, #78553 ) ;
#42057=VECTOR ( 'NONE', #75409, 1000.000000000000000 ) ;
#42085=PLANE ( 'NONE',  #43627 ) ;
#42093=CARTESIAN_POINT ( 'NONE',  ( -179.8898777604655095, 20.32000000000000028, -12.69999999999999929 ) ) ;
#42113=AXIS2_PLACEMENT_3D ( 'NONE', #85375, #50363, #51698 ) ;
#42139=CYLINDRICAL_SURFACE ( 'NONE', #81180, 218.1859999999999786 ) ;
#42149=CARTESIAN_POINT ( 'NONE',  ( 109.6133334940117976, 49.38454753513003226, 70.92099578410642380 ) ) ;
#42159=PLANE ( 'NONE',  #54684 ) ;
#42162=ADVANCED_FACE ( 'NONE', ( #75157 ), #4778, .T. ) ;
#42181=CARTESIAN_POINT ( 'NONE',  ( -148.0533267522752112, 20.32000000000000028, 160.2664750769289697 ) ) ;
#42203=EDGE_CURVE ( 'NONE', #66001, #13914, #69241, .T. ) ;
#42213=CIRCLE ( 'NONE', #37889, 218.1859999999999786 ) ;
#42219=CARTESIAN_POINT ( 'NONE',  ( 7.060148683296544547, 71.99328113033080001, 130.3649624909047020 ) ) ;
#42226=CARTESIAN_POINT ( 'NONE',  ( 123.1844716773658348, 44.88724112343236072, -43.24955686283671952 ) ) ;
#42242=CARTESIAN_POINT ( 'NONE',  ( 31.75000000000000000, 8.255000000000000782, 3.174999999999999822 ) ) ;
#42257=VERTEX_POINT ( 'NONE', #7010 ) ;
#42285=LINE ( 'NONE', #23238, #53463 ) ;
#42337=AXIS2_PLACEMENT_3D ( 'NONE', #29849, #57082, #16221 ) ;
#42366=CARTESIAN_POINT ( 'NONE',  ( 12.62678658230826123, 80.95407853623918015, 129.9444177315847355 ) ) ;
#42373=EDGE_CURVE ( 'NONE', #16001, #28030, #79203, .T. ) ;
#42390=ADVANCED_FACE ( 'NONE', ( #57386, #38284 ), #85129, .F. ) ;
#42407=PLANE ( 'NONE',  #84619 ) ;
#42433=CARTESIAN_POINT ( 'NONE',  ( 131.3179999999999836, 53.97500000000000142, 50.79999999999999716 ) ) ;
#42437=ORIENTED_EDGE ( 'NONE', *, *, #3798, .F. ) ;
#42439=ORIENTED_EDGE ( 'NONE', *, *, #13605, .F. ) ;
#42448=CARTESIAN_POINT ( 'NONE',  ( 0.000000000000000000, 101.5999999999999943, 0.000000000000000000 ) ) ;
#42449=CARTESIAN_POINT ( 'NONE',  ( -125.2253049228147290, 69.25379042415792696, 36.92573596021566829 ) ) ;
#42478=DIRECTION ( 'NONE',  ( 0.000000000000000000, 0.000000000000000000, 1.000000000000000000 ) ) ;
#42482=CARTESIAN_POINT ( 'NONE',  ( -215.9010000000000105, 52.73749999999999716, -36.51250000000000284 ) ) ;
#42483=DIRECTION ( 'NONE',  ( 0.000000000000000000, 0.000000000000000000, 1.000000000000000000 ) ) ;
#42500=DIRECTION ( 'NONE',  ( 0.000000000000000000, 0.000000000000000000, 1.000000000000000000 ) ) ;
#42504=EDGE_CURVE ( 'NONE', #13582, #12226, #66568, .T. ) ;
#42511=ORIENTED_EDGE ( 'NONE', *, *, #47315, .F. ) ;
#42519=EDGE_LOOP ( 'NONE', ( #88061, #76382, #3279, #68146 ) ) ;
#42547=ORIENTED_EDGE ( 'NONE', *, *, #191, .T. ) ;
#42557=ORIENTED_EDGE ( 'NONE', *, *, #75434, .T. ) ;
#42565=DIRECTION ( 'NONE',  ( 0.000000000000000000, -1.000000000000000000, 0.000000000000000000 ) ) ;
#42575=CIRCLE ( 'NONE', #3446, 38.10000000000000142 ) ;
#42588=CARTESIAN_POINT ( 'NONE',  ( 109.2774118001977826, 53.13983499867891425, 71.43750000000004263 ) ) ;
#42621=VERTEX_POINT ( 'NONE', #9933 ) ;
#42638=DIRECTION ( 'NONE',  ( -1.000000000000000000, 0.000000000000000000, -2.108231265501709878E-16 ) ) ;
#42639=VECTOR ( 'NONE', #63265, 1000.000000000000000 ) ;
#42642=EDGE_LOOP ( 'NONE', ( #35249, #44665, #76410, #38870 ) ) ;
#42693=CARTESIAN_POINT ( 'NONE',  ( 124.6194816332305635, 70.85869709054320253, 38.92310640268541988 ) ) ;
#42706=CIRCLE ( 'NONE', #60076, 9.525000000000000355 ) ;
#42719=DIRECTION ( 'NONE',  ( 6.982966722218760189E-15, 0.000000000000000000, 1.000000000000000000 ) ) ;
#42729=DIRECTION ( 'NONE',  ( -1.000000000000000000, 0.000000000000000000, -2.108231265501709878E-16 ) ) ;
#42749=CARTESIAN_POINT ( 'NONE',  ( -123.4696824136392053, 0.000000000000000000, -179.8898777604655095 ) ) ;
#42762=CARTESIAN_POINT ( 'NONE',  ( 3.174999999999889688, 24.56180297284579694, -31.75000000000000000 ) ) ;
#42800=VERTEX_POINT ( 'NONE', #56823 ) ;
#42813=CARTESIAN_POINT ( 'NONE',  ( 11.74129241494043896, 77.70931405037566719, 130.0269635525507965 ) ) ;
#42838=ORIENTED_EDGE ( 'NONE', *, *, #43090, .F. ) ;
#42883=CARTESIAN_POINT ( 'NONE',  ( 1.926769467660224795E-14, 17.78000000000000114, 154.1697486074984909 ) ) ;
#42885=ORIENTED_EDGE ( 'NONE', *, *, #3523, .T. ) ;
#42931=CARTESIAN_POINT ( 'NONE',  ( 0.000000000000000000, 101.5999999999999943, 0.000000000000000000 ) ) ;
#42945=ADVANCED_FACE ( 'NONE', ( #88919 ), #4898, .T. ) ;
#42966=ORIENTED_EDGE ( 'NONE', *, *, #46067, .T. ) ;
#42975=CARTESIAN_POINT ( 'NONE',  ( -12.39034654063912555, 85.36816127604853932, 129.9671126930435037 ) ) ;
#43016=EDGE_CURVE ( 'NONE', #51337, #28246, #55258, .T. ) ;
#43025=DIRECTION ( 'NONE',  ( 0.000000000000000000, -1.000000000000000000, 0.000000000000000000 ) ) ;
#43038=CARTESIAN_POINT ( 'NONE',  ( -20.44586087093906812, 62.81651420408395126, 32.15007357241096031 ) ) ;
#43052=DIRECTION ( 'NONE',  ( 0.000000000000000000, -1.000000000000000000, 0.000000000000000000 ) ) ;
#43073=VECTOR ( 'NONE', #75227, 1000.000000000000000 ) ;
#43075=LINE ( 'NONE', #42181, #68023 ) ;
#43090=EDGE_CURVE ( 'NONE', #85960, #77712, #36716, .T. ) ;
#43106=CARTESIAN_POINT ( 'NONE',  ( 3.174999999999879918, 17.78000000000000114, -33.98325472291465132 ) ) ;
#43119=CARTESIAN_POINT ( 'NONE',  ( 125.2199481402020353, 50.10030656833554019, -36.94431110519001749 ) ) ;
#43122=VERTEX_POINT ( 'NONE', #61524 ) ;
#43123=ORIENTED_EDGE ( 'NONE', *, *, #28135, .T. ) ;
#43128=CARTESIAN_POINT ( 'NONE',  ( 57.91199999999999903, 101.5999999999999943, 178.6098374884404905 ) ) ;
#43149=CARTESIAN_POINT ( 'NONE',  ( 126.1219783984286238, 65.58371290633178319, 33.73612174402128971 ) ) ;
#43158=VERTEX_POINT ( 'NONE', #4348 ) ;
#43166=SURFACE_STYLE_USAGE ( .BOTH. , #48181 ) ;
#43180=PLANE ( 'NONE',  #23406 ) ;
#43224=EDGE_CURVE ( 'NONE', #65312, #61695, #35163, .T. ) ;
#43233=DIRECTION ( 'NONE',  ( 0.000000000000000000, 1.000000000000000000, 0.000000000000000000 ) ) ;
#43271=CYLINDRICAL_SURFACE ( 'NONE', #32163, 7.874000000000227928 ) ;
#43336=FACE_OUTER_BOUND ( 'NONE', #41806, .T. ) ;
#43342=VERTEX_POINT ( 'NONE', #55587 ) ;
#43367=VERTEX_POINT ( 'NONE', #76514 ) ;
#43379=LINE ( 'NONE', #78390, #54891 ) ;
#43384=CYLINDRICAL_SURFACE ( 'NONE', #3493, 20.63750000000000284 ) ;
#43386=CARTESIAN_POINT ( 'NONE',  ( 160.2664750769289697, 101.5999999999999943, 148.0533267522752112 ) ) ;
#43392=CARTESIAN_POINT ( 'NONE',  ( 208.9149999999999920, 37.33800000000000097, 60.32499999999999574 ) ) ;
#43427=CARTESIAN_POINT ( 'NONE',  ( -12.62695347127759327, 84.14402871178053545, 129.9443987845095876 ) ) ;
#43432=CARTESIAN_POINT ( 'NONE',  ( 126.4481529151155996, 44.45000000000000284, 32.49205688096009936 ) ) ;
#43442=EDGE_CURVE ( 'NONE', #30970, #74824, #9713, .T. ) ;
#43447=EDGE_CURVE ( 'NONE', #72639, #13914, #71947, .T. ) ;
#43464=CARTESIAN_POINT ( 'NONE',  ( -109.4095239551054419, 50.64688101357703687, 71.23662271831288706 ) ) ;
#43470=CARTESIAN_POINT ( 'NONE',  ( 0.000000000000000000, 2.031999999999865025, 0.000000000000000000 ) ) ;
#43477=EDGE_CURVE ( 'NONE', #33479, #77555, #75400, .T. ) ;
#43489=CARTESIAN_POINT ( 'NONE',  ( -10.76925785606963437, 68.90738082334692649, 36.55253304027624495 ) ) ;
#43492=VECTOR ( 'NONE', #57487, 1000.000000000000000 ) ;
#43496=CARTESIAN_POINT ( 'NONE',  ( 173.9900000000000091, 37.33800000000000097, 69.13087104677069306 ) ) ;
#43504=EDGE_CURVE ( 'NONE', #54166, #48373, #2904, .T. ) ;
#43527=CYLINDRICAL_SURFACE ( 'NONE', #2809, 218.1859999999999786 ) ;
#43530=AXIS2_PLACEMENT_3D ( 'NONE', #41138, #48837, #68862 ) ;
#43550=EDGE_LOOP ( 'NONE', ( #14545, #55612, #38390, #9857 ) ) ;
#43559=CARTESIAN_POINT ( 'NONE',  ( -20.89537973703602347, 45.76944718839217074, 31.86023317849521419 ) ) ;
#43561=DIRECTION ( 'NONE',  ( 0.000000000000000000, -1.000000000000000000, 0.000000000000000000 ) ) ;
#43568=ORIENTED_EDGE ( 'NONE', *, *, #70242, .F. ) ;
#43577=DIRECTION ( 'NONE',  ( 0.000000000000000000, -1.000000000000000000, 0.000000000000000000 ) ) ;
#43597=CARTESIAN_POINT ( 'NONE',  ( 124.3932715389403256, 71.33461644843129079, 39.63843969546147861 ) ) ;
#43627=AXIS2_PLACEMENT_3D ( 'NONE', #28014, #76627, #21675 ) ;
#43650=EDGE_LOOP ( 'NONE', ( #13889, #30304, #24869, #42437 ) ) ;
#43669=EDGE_CURVE ( 'NONE', #71713, #77555, #5585, .T. ) ;
#43679=VECTOR ( 'NONE', #43233, 1000.000000000000000 ) ;
#43718=CARTESIAN_POINT ( 'NONE',  ( 11.13113089042260384, 76.43192475021864141, 130.0807045952973908 ) ) ;
#43748=CARTESIAN_POINT ( 'NONE',  ( 7.028760451216134797, 93.12764692289525215, 130.3666587255899287 ) ) ;
#43757=EDGE_CURVE ( 'NONE', #15522, #30970, #75961, .T. ) ;
#43772=CARTESIAN_POINT ( 'NONE',  ( -179.8898777604655095, 101.5999999999999943, -12.69999999999999929 ) ) ;
#43773=DIRECTION ( 'NONE',  ( 0.000000000000000000, 0.000000000000000000, 1.000000000000000000 ) ) ;
#43788=VERTEX_POINT ( 'NONE', #7811 ) ;
#43799=AXIS2_PLACEMENT_3D ( 'NONE', #57131, #43052, #76705 ) ;
#43817=AXIS2_PLACEMENT_3D ( 'NONE', #65673, #79333, #17098 ) ;
#43831=ADVANCED_FACE ( 'NONE', ( #1000 ), #48672, .T. ) ;
#43838=VECTOR ( 'NONE', #81852, 1000.000000000000000 ) ;
#43880=CARTESIAN_POINT ( 'NONE',  ( -1.596709470477730486, 95.17668143650945467, 130.5484419168967349 ) ) ;
#43914=CARTESIAN_POINT ( 'NONE',  ( -110.5284195268215228, 45.17989370491086731, 69.48768198397286255 ) ) ;
#43927=CARTESIAN_POINT ( 'NONE',  ( 21.33963204133176461, 61.45598276206009558, 31.56377395493905524 ) ) ;
#43962=DIRECTION ( 'NONE',  ( 0.000000000000000000, 0.000000000000000000, 1.000000000000000000 ) ) ;
#43971=VERTEX_POINT ( 'NONE', #77757 ) ;
#43984=CARTESIAN_POINT ( 'NONE',  ( 1.166476076187854022E-15, 114.2999999999999972, 9.525000000000000355 ) ) ;
#44011=CARTESIAN_POINT ( 'NONE',  ( 125.3463460965257070, 52.73749999999999716, -36.51249999999992468 ) ) ;
#44041=CARTESIAN_POINT ( 'NONE',  ( 126.7473051586034387, 60.90675218994213225, 31.31017718299094454 ) ) ;
#44048=DIRECTION ( 'NONE',  ( 0.000000000000000000, 0.000000000000000000, -1.000000000000000000 ) ) ;
#44054=DIRECTION ( 'NONE',  ( -1.000000000000000000, 0.000000000000000000, 0.000000000000000000 ) ) ;
#44068=EDGE_CURVE ( 'NONE', #71033, #46484, #73153, .T. ) ;
#44078=DIRECTION ( 'NONE',  ( 0.7071067811865370256, 0.000000000000000000, -0.7071067811865580088 ) ) ;
#44125=EDGE_CURVE ( 'NONE', #7095, #84589, #11660, .T. ) ;
#44132=EDGE_CURVE ( 'NONE', #64884, #60724, #85665, .T. ) ;
#44185=CARTESIAN_POINT ( 'NONE',  ( 1.595580815131592001, 95.17678229987137684, 130.5484528442787564 ) ) ;
#44204=LINE ( 'NONE', #50131, #55275 ) ;
#44210=EDGE_LOOP ( 'NONE', ( #30247, #37561 ) ) ;
#44232=VERTEX_POINT ( 'NONE', #12735 ) ;
#44253=CARTESIAN_POINT ( 'NONE',  ( 3.175000000000334666, 8.255000000000000782, 31.75000000000000000 ) ) ;
#44293=AXIS2_PLACEMENT_3D ( 'NONE', #9049, #28571, #14964 ) ;
#44306=EDGE_CURVE ( 'NONE', #19042, #19304, #49007, .T. ) ;
#44313=EDGE_CURVE ( 'NONE', #18319, #18059, #89033, .T. ) ;
#44321=DIRECTION ( 'NONE',  ( -1.000000000000000000, 0.000000000000000000, 0.000000000000000000 ) ) ;
#44322=CARTESIAN_POINT ( 'NONE',  ( -7.105823921952652888, 93.07605504633957594, 130.3624800658744505 ) ) ;
#44339=ADVANCED_FACE ( 'NONE', ( #13182 ), #75849, .F. ) ;
#44354=VERTEX_POINT ( 'NONE', #76296 ) ;
#44364=CARTESIAN_POINT ( 'NONE',  ( -160.2664750769284865, 101.5999999999999943, 148.0533267522753818 ) ) ;
#44375=CARTESIAN_POINT ( 'NONE',  ( 22.82730048992621263, 57.73250703860936994, 30.50469867578552652 ) ) ;
#44376=AXIS2_PLACEMENT_3D ( 'NONE', #15047, #42719, #55447 ) ;
#44384=ORIENTED_EDGE ( 'NONE', *, *, #3902, .T. ) ;
#44396=DIRECTION ( 'NONE',  ( 0.000000000000000000, -1.000000000000000000, 0.000000000000000000 ) ) ;
#44415=EDGE_CURVE ( 'NONE', #40497, #28660, #26793, .T. ) ;
#44429=CARTESIAN_POINT ( 'NONE',  ( 0.000000000000000000, 101.5999999999999943, 0.000000000000000000 ) ) ;
#44450=ADVANCED_FACE ( 'NONE', ( #50823 ), #78993, .F. ) ;
#44485=PLANE ( 'NONE',  #85463 ) ;
#44490=CARTESIAN_POINT ( 'NONE',  ( 116.8422689635382454, 73.23116755977939363, 58.25111782077112110 ) ) ;
#44495=CARTESIAN_POINT ( 'NONE',  ( 173.9900000000000091, 20.32000000000000028, -71.37400000000000944 ) ) ;
#44498=ORIENTED_EDGE ( 'NONE', *, *, #45114, .T. ) ;
#44530=ADVANCED_FACE ( 'NONE', ( #85820 ), #22243, .T. ) ;
#44534=AXIS2_PLACEMENT_3D ( 'NONE', #19459, #61233, #76212 ) ;
#44547=DIRECTION ( 'NONE',  ( 0.000000000000000000, 0.000000000000000000, 1.000000000000000000 ) ) ;
#44573=ADVANCED_FACE ( 'NONE', ( #23587, #49913 ), #51250, .T. ) ;
#44633=CARTESIAN_POINT ( 'NONE',  ( 5.565016159906887694, 93.97330845465467064, 130.4378072086274756 ) ) ;
#44635=CARTESIAN_POINT ( 'NONE',  ( 0.000000000000000000, 1.270000000000000018, 0.000000000000000000 ) ) ;
#44652=FACE_OUTER_BOUND ( 'NONE', #53492, .T. ) ;
#44660=CARTESIAN_POINT ( 'NONE',  ( -215.9000000000000057, 101.5999999999999943, 146.9389999999999930 ) ) ;
#44665=ORIENTED_EDGE ( 'NONE', *, *, #3028, .F. ) ;
#44670=FACE_BOUND ( 'NONE', #22006, .T. ) ;
#44709=ORIENTED_EDGE ( 'NONE', *, *, #17626, .F. ) ;
#44719=DIRECTION ( 'NONE',  ( 0.000000000000000000, 1.000000000000000000, 0.000000000000000000 ) ) ;
#44728=ORIENTED_EDGE ( 'NONE', *, *, #50519, .F. ) ;
#44738=CARTESIAN_POINT ( 'NONE',  ( -187.8075999999999794, 20.32000000000000028, -9.525000000000000355 ) ) ;
#44742=VECTOR ( 'NONE', #13598, 1000.000000000000000 ) ;
#44749=VECTOR ( 'NONE', #54484, 1000.000000000000000 ) ;
#44755=CIRCLE ( 'NONE', #51931, 130.5560000000000116 ) ;
#44775=CARTESIAN_POINT ( 'NONE',  ( -5.170486730135384512, 94.15052322753994929, 130.4536157927243778 ) ) ;
#44782=CARTESIAN_POINT ( 'NONE',  ( 0.000000000000000000, 11.98343896644750117, 0.000000000000000000 ) ) ;
#44868=ORIENTED_EDGE ( 'NONE', *, *, #2468, .F. ) ;
#44888=AXIS2_PLACEMENT_3D ( 'NONE', #75236, #14358, #267 ) ;
#44892=CARTESIAN_POINT ( 'NONE',  ( 122.2688682072174942, 60.56780087056017692, -45.77403049370062860 ) ) ;
#44925=AXIS2_PLACEMENT_3D ( 'NONE', #5715, #61550, #46116 ) ;
#44930=CARTESIAN_POINT ( 'NONE',  ( 160.2664750769284865, 101.5999999999999943, -148.0533267522753818 ) ) ;
#44931=FACE_OUTER_BOUND ( 'NONE', #68616, .T. ) ;
#44934=DIRECTION ( 'NONE',  ( 0.000000000000000000, 0.000000000000000000, 1.000000000000000000 ) ) ;
#44936=CARTESIAN_POINT ( 'NONE',  ( 110.6772377970183214, 63.23435454354248009, 69.24934357568848498 ) ) ;
#44976=ORIENTED_EDGE ( 'NONE', *, *, #9007, .T. ) ;
#45053=DIRECTION ( 'NONE',  ( -1.000000000000000000, 0.000000000000000000, -2.108231265501709878E-16 ) ) ;
#45070=CARTESIAN_POINT ( 'NONE',  ( -135.1318726873890341, 20.32000000000000028, 118.7423475625884066 ) ) ;
#45083=ADVANCED_FACE ( 'NONE', ( #37432, #45113 ), #36982, .T. ) ;
#45113=FACE_BOUND ( 'NONE', #4261, .T. ) ;
#45114=EDGE_CURVE ( 'NONE', #74303, #3666, #65132, .T. ) ;
#45155=CARTESIAN_POINT ( 'NONE',  ( -3.452160436674259536, 70.12364187744314847, 37.94944277985399594 ) ) ;
#45184=ORIENTED_EDGE ( 'NONE', *, *, #5053, .T. ) ;
#45185=VERTEX_POINT ( 'NONE', #19661 ) ;
#45186=VECTOR ( 'NONE', #47165, 1000.000000000000000 ) ;
#45211=CARTESIAN_POINT ( 'NONE',  ( -10.66780431135453000, 89.44155629055205736, 130.1194439449466813 ) ) ;
#45245=CARTESIAN_POINT ( 'NONE',  ( 208.9149999999999920, 43.68799999999999528, 57.14999999999999858 ) ) ;
#45266=DIRECTION ( 'NONE',  ( -7.867884063170659983E-16, 0.000000000000000000, 1.000000000000000000 ) ) ;
#45327=CARTESIAN_POINT ( 'NONE',  ( 119.7718215552501704, 55.36764569511297651, -51.95798173397368203 ) ) ;
#45348=EDGE_CURVE ( 'NONE', #82724, #84701, #64181, .T. ) ;
#45352=EDGE_LOOP ( 'NONE', ( #69723, #7523 ) ) ;
#45362=ORIENTED_EDGE ( 'NONE', *, *, #68027, .F. ) ;
#45376=CARTESIAN_POINT ( 'NONE',  ( 118.6191002195142374, 74.28059613835587527, 54.54229135122187699 ) ) ;
#45392=ORIENTED_EDGE ( 'NONE', *, *, #36972, .T. ) ;
#45402=LINE ( 'NONE', #79520, #25112 ) ;
#45403=CARTESIAN_POINT ( 'NONE',  ( 0.000000000000000000, 0.000000000000000000, 0.000000000000000000 ) ) ;
#45406=ADVANCED_FACE ( 'NONE', ( #59568, #10986 ), #86861, .T. ) ;
#45438=( LENGTH_UNIT ( ) NAMED_UNIT ( * ) SI_UNIT ( .MILLI., .METRE. ) );
#45440=CARTESIAN_POINT ( 'NONE',  ( -215.9000000000000057, 53.97500000000000142, 50.79999999999999716 ) ) ;
#45447=AXIS2_PLACEMENT_3D ( 'NONE', #62072, #1664, #70241 ) ;
#45467=ORIENTED_EDGE ( 'NONE', *, *, #74422, .T. ) ;
#45475=ORIENTED_EDGE ( 'NONE', *, *, #17502, .T. ) ;
#45570=AXIS2_PLACEMENT_3D ( 'NONE', #29331, #84310, #85646 ) ;
#45571=EDGE_CURVE ( 'NONE', #14989, #51056, #34108, .T. ) ;
#45588=CARTESIAN_POINT ( 'NONE',  ( -1.415542646969860267E-16, 70.24203434096102683, 38.10000000000000142 ) ) ;
#45594=CARTESIAN_POINT ( 'NONE',  ( -187.8075999999999794, 101.5999999999999943, 107.9500000000000028 ) ) ;
#45634=CARTESIAN_POINT ( 'NONE',  ( -31.75000000000000000, 8.255000000000000782, -3.174999999999779998 ) ) ;
#45651=CARTESIAN_POINT ( 'NONE',  ( 126.8694562117858595, 48.85726633079141834, 30.80605124856342414 ) ) ;
#45672=VERTEX_POINT ( 'NONE', #62270 ) ;
#45698=CARTESIAN_POINT ( 'NONE',  ( -2.818947171159547960, 70.15983271286830814, 130.5258393308032225 ) ) ;
#45721=FACE_BOUND ( 'NONE', #37465, .T. ) ;
#45760=CIRCLE ( 'NONE', #80558, 7.874000000000186184 ) ;
#45792=VERTEX_POINT ( 'NONE', #28651 ) ;
#45805=DIRECTION ( 'NONE',  ( 0.000000000000000000, 1.000000000000000000, 0.000000000000000000 ) ) ;
#45814=CARTESIAN_POINT ( 'NONE',  ( 120.1084960442967002, 74.60926949527541296, 51.17446912123692471 ) ) ;
#45819=CARTESIAN_POINT ( 'NONE',  ( 173.9900000000000091, 0.000000000000000000, 131.6533725204182019 ) ) ;
#45830=VECTOR ( 'NONE', #10160, 1000.000000000000000 ) ;
#45836=DIRECTION ( 'NONE',  ( 0.000000000000000000, -1.000000000000000000, 0.000000000000000000 ) ) ;
#45858=CARTESIAN_POINT ( 'NONE',  ( -186.2398777604655038, 20.32000000000000028, -6.349999999999999645 ) ) ;
#45910=EDGE_LOOP ( 'NONE', ( #37956, #22158, #74913, #36649 ) ) ;
#45911=CARTESIAN_POINT ( 'NONE',  ( 148.0533267522749838, 0.000000000000000000, -160.2664750769289697 ) ) ;
#45934=B_SPLINE_CURVE_WITH_KNOTS ( 'NONE', 3,
 ( #29866, #43914, #84837, #50279, #77559, #35763, #78475, #77120, #85292, #49385, #50740, #43464, #23068, #35310 ),
 .UNSPECIFIED., .F., .F.,
 ( 4, 2, 2, 1, 1, 2, 2, 4 ),
 ( 0.000000000000000000, 0.2499999999999974465, 0.3749999999999963918, 0.4374999999999964473, 0.4687499999999965583, 0.4843749999999975575, 0.4999999999999985567, 1.000000000000000000 ),
 .UNSPECIFIED. ) ;
#45953=ORIENTED_EDGE ( 'NONE', *, *, #78002, .F. ) ;
#45956=VERTEX_POINT ( 'NONE', #10450 ) ;
#45957=EDGE_CURVE ( 'NONE', #71033, #53038, #80397, .T. ) ;
#45975=EDGE_LOOP ( 'NONE', ( #8854, #49931, #62624, #46137 ) ) ;
#46040=CARTESIAN_POINT ( 'NONE',  ( -19.63071693306478949, 63.82648643955351986, 32.65698028270841036 ) ) ;
#46067=EDGE_CURVE ( 'NONE', #28660, #44232, #3168, .T. ) ;
#46102=CARTESIAN_POINT ( 'NONE',  ( 126.9648347381352949, 50.67849012603234371, 30.41069370691922558 ) ) ;
#46114=ORIENTED_EDGE ( 'NONE', *, *, #86304, .F. ) ;
#46116=DIRECTION ( 'NONE',  ( 0.000000000000000000, 0.000000000000000000, 1.000000000000000000 ) ) ;
#46123=CARTESIAN_POINT ( 'NONE',  ( -109.5351475254747839, 57.99849859213713898, 71.04168492196464513 ) ) ;
#46127=EDGE_LOOP ( 'NONE', ( #15281, #52794, #59977, #70163, #42838, #11161, #23952, #7409, #79466, #16267, #78582 ) ) ;
#46137=ORIENTED_EDGE ( 'NONE', *, *, #65769, .F. ) ;
#46151=DIRECTION ( 'NONE',  ( 0.000000000000000000, 0.000000000000000000, 1.000000000000000000 ) ) ;
#46157=LINE ( 'NONE', #25286, #77066 ) ;
#46176=ORIENTED_EDGE ( 'NONE', *, *, #3216, .F. ) ;
#46209=AXIS2_PLACEMENT_3D ( 'NONE', #20080, #25992, #68674 ) ;
#46217=CARTESIAN_POINT ( 'NONE',  ( 120.1244329748395643, 57.02142899650635854, -51.13721865063806860 ) ) ;
#46235=VERTEX_POINT ( 'NONE', #12694 ) ;
#46254=LINE ( 'NONE', #66264, #62280 ) ;
#46259=CARTESIAN_POINT ( 'NONE',  ( 111.6142026935021079, 65.77908918206766486, 67.72842572080216428 ) ) ;
#46271=ADVANCED_FACE ( 'NONE', ( #69889 ), #22648, .T. ) ;
#46275=CARTESIAN_POINT ( 'NONE',  ( -194.1576000000000022, 101.5999999999999943, -45.33899999999999864 ) ) ;
#46333=CARTESIAN_POINT ( 'NONE',  ( 0.000000000000000000, 20.32000000000000028, 0.000000000000000000 ) ) ;
#46356=CARTESIAN_POINT ( 'NONE',  ( 0.000000000000000000, 12.27000000000000313, -9.525000000000000355 ) ) ;
#46362=VERTEX_POINT ( 'NONE', #64417 ) ;
#46365=EDGE_CURVE ( 'NONE', #79928, #34694, #69946, .T. ) ;
#46379=DIRECTION ( 'NONE',  ( 1.000000000000000000, 0.000000000000000000, 0.000000000000000000 ) ) ;
#46413=EDGE_LOOP ( 'NONE', ( #18673, #5105, #7484, #30723 ) ) ;
#46424=EDGE_CURVE ( 'NONE', #21031, #57125, #66638, .T. ) ;
#46431=DIRECTION ( 'NONE',  ( 0.000000000000000000, 0.000000000000000000, -1.000000000000000000 ) ) ;
#46446=DIRECTION ( 'NONE',  ( 0.000000000000000000, 1.000000000000000000, 0.000000000000000000 ) ) ;
#46484=VERTEX_POINT ( 'NONE', #65738 ) ;
#46499=ADVANCED_FACE ( 'NONE', ( #58045 ), #86653, .T. ) ;
#46531=CIRCLE ( 'NONE', #11539, 6.349999999999999645 ) ;
#46547=AXIS2_PLACEMENT_3D ( 'NONE', #44364, #17128, #71652 ) ;
#46607=CARTESIAN_POINT ( 'NONE',  ( 170.2205283966864897, 20.32000000000000028, -79.24800000000000466 ) ) ;
#46612=ORIENTED_EDGE ( 'NONE', *, *, #61993, .F. ) ;
#46617=VECTOR ( 'NONE', #89323, 1000.000000000000000 ) ;
#46669=VECTOR ( 'NONE', #64847, 1000.000000000000000 ) ;
#46705=ORIENTED_EDGE ( 'NONE', *, *, #63956, .T. ) ;
#46706=CIRCLE ( 'NONE', #27921, 12.69999999999998863 ) ;
#46707=CARTESIAN_POINT ( 'NONE',  ( -178.3658777604659917, 0.000000000000000000, 122.9960808104842016 ) ) ;
#46783=LINE ( 'NONE', #12294, #9889 ) ;
#46784=DIRECTION ( 'NONE',  ( 0.000000000000000000, 1.000000000000000000, 0.000000000000000000 ) ) ;
#46792=EDGE_CURVE ( 'NONE', #33670, #26732, #10283, .T. ) ;
#46852=ORIENTED_EDGE ( 'NONE', *, *, #23860, .F. ) ;
#46887=DIRECTION ( 'NONE',  ( 0.000000000000000000, -1.000000000000000000, 0.000000000000000000 ) ) ;
#46908=CARTESIAN_POINT ( 'NONE',  ( -135.1318726873890341, 101.5999999999999943, 118.7423475625884066 ) ) ;
#46939=CARTESIAN_POINT ( 'NONE',  ( -21.81213075493552012, 60.58772898943853846, 31.24010949910693924 ) ) ;
#46950=CARTESIAN_POINT ( 'NONE',  ( 31.75000000000000000, 24.56180297284579694, 3.174999999999999822 ) ) ;
#46960=FACE_OUTER_BOUND ( 'NONE', #14148, .T. ) ;
#46997=PRODUCT_DEFINITION_SHAPE ( 'NONE', 'NONE',  #80551 ) ;
#47017=CARTESIAN_POINT ( 'NONE',  ( -111.3778403937640604, 65.20424434049171225, 68.11656773419859690 ) ) ;
#47018=VERTEX_POINT ( 'NONE', #23879 ) ;
#47044=CARTESIAN_POINT ( 'NONE',  ( -10.55578339146518196, 75.48845273559737734, 130.1285694115591696 ) ) ;
#47072=CIRCLE ( 'NONE', #74645, 9.525000000000000355 ) ;
#47079=VECTOR ( 'NONE', #53107, 1000.000000000000000 ) ;
#47081=CARTESIAN_POINT ( 'NONE',  ( -126.6438945437297292, 45.91417521994105755, 31.73029632275546774 ) ) ;
#47090=VERTEX_POINT ( 'NONE', #20957 ) ;
#47101=CARTESIAN_POINT ( 'NONE',  ( 0.000000000000000000, 44.45000000000000284, 0.000000000000000000 ) ) ;
#47113=PLANE ( 'NONE',  #6965 ) ;
#47165=DIRECTION ( 'NONE',  ( 0.000000000000000000, -1.000000000000000000, 0.000000000000000000 ) ) ;
#47168=DIRECTION ( 'NONE',  ( 0.000000000000000000, 0.000000000000000000, 1.000000000000000000 ) ) ;
#47179=VERTEX_POINT ( 'NONE', #4491 ) ;
#47183=ORIENTED_EDGE ( 'NONE', *, *, #58581, .T. ) ;
#47194=CIRCLE ( 'NONE', #31255, 6.349999999999994316 ) ;
#47216=ORIENTED_EDGE ( 'NONE', *, *, #44313, .T. ) ;
#47235=DIRECTION ( 'NONE',  ( 0.000000000000000000, 0.000000000000000000, 1.000000000000000000 ) ) ;
#47271=LINE ( 'NONE', #58341, #55390 ) ;
#47309=CARTESIAN_POINT ( 'NONE',  ( 11.02882537043472233, 88.86092628232667323, 130.0895302200946162 ) ) ;
#47315=EDGE_CURVE ( 'NONE', #72419, #64158, #5839, .T. ) ;
#47327=AXIS2_PLACEMENT_3D ( 'NONE', #81125, #68814, #5702 ) ;
#47341=EDGE_LOOP ( 'NONE', ( #29544, #58226, #22481, #61793 ) ) ;
#47347=CARTESIAN_POINT ( 'NONE',  ( -186.2398777604659870, 20.32000000000000028, 107.9500000000000028 ) ) ;
#47365=VERTEX_POINT ( 'NONE', #66704 ) ;
#47376=ORIENTED_EDGE ( 'NONE', *, *, #59013, .T. ) ;
#47426=FACE_OUTER_BOUND ( 'NONE', #76142, .T. ) ;
#47452=EDGE_CURVE ( 'NONE', #42257, #34850, #6717, .T. ) ;
#47464=CARTESIAN_POINT ( 'NONE',  ( -20.16291403587278097, 44.76340627898822078, 32.32900225554683260 ) ) ;
#47469=AXIS2_PLACEMENT_3D ( 'NONE', #24404, #31195, #46151 ) ;
#47497=CARTESIAN_POINT ( 'NONE',  ( -11.60276384529982430, 77.38453301234325465, 130.0394192264149922 ) ) ;
#47529=CIRCLE ( 'NONE', #4030, 24.63800000000000168 ) ;
#47532=VERTEX_POINT ( 'NONE', #41729 ) ;
#47542=DIRECTION ( 'NONE',  ( 0.000000000000000000, 0.000000000000000000, 1.000000000000000000 ) ) ;
#47607=DIRECTION ( 'NONE',  ( 1.000000000000000000, 0.000000000000000000, 2.108231265501709878E-16 ) ) ;
#47612=DIRECTION ( 'NONE',  ( -8.503806984168940141E-16, 0.000000000000000000, 1.000000000000000000 ) ) ;
#47638=FACE_OUTER_BOUND ( 'NONE', #77858, .T. ) ;
#47655=ORIENTED_EDGE ( 'NONE', *, *, #5558, .T. ) ;
#47686=CARTESIAN_POINT ( 'NONE',  ( 9.673933672768200154, 74.31810048158574489, 130.1973409905385495 ) ) ;
#47692=CARTESIAN_POINT ( 'NONE',  ( 122.9163323945412998, 44.80836990040677392, -44.00586793101803806 ) ) ;
#47722=CARTESIAN_POINT ( 'NONE',  ( 173.9900000000000091, 101.5999999999999943, -131.6533725204182019 ) ) ;
#47758=CARTESIAN_POINT ( 'NONE',  ( 10.54753116919433964, 89.62386675693470295, 130.1292385957734155 ) ) ;
#47786=PLANE ( 'NONE',  #32964 ) ;
#47827=DIRECTION ( 'NONE',  ( 0.000000000000000000, -1.000000000000000000, 0.000000000000000000 ) ) ;
#47848=CARTESIAN_POINT ( 'NONE',  ( 183.5150000000000148, 37.33800000000000097, 41.27499999999999858 ) ) ;
#47849=ADVANCED_FACE ( 'NONE', ( #72601 ), #10366, .F. ) ;
#47876=FACE_BOUND ( 'NONE', #40649, .T. ) ;
#47895=DIRECTION ( 'NONE',  ( 0.000000000000000000, -1.000000000000000000, 0.000000000000000000 ) ) ;
#47898=CIRCLE ( 'NONE', #17521, 218.1859999999999786 ) ;
#47910=EDGE_CURVE ( 'NONE', #75634, #5474, #26786, .T. ) ;
#47914=DIRECTION ( 'NONE',  ( 0.000000000000000000, 1.000000000000000000, 0.000000000000000000 ) ) ;
#47915=CARTESIAN_POINT ( 'NONE',  ( -113.6350504498463323, 69.61314433698439075, 64.28280664495177632 ) ) ;
#47936=LINE ( 'NONE', #25723, #88027 ) ;
#47941=CARTESIAN_POINT ( 'NONE',  ( -9.688862330989991278, 74.32879814653003336, 130.1964161894449035 ) ) ;
#47949=ORIENTED_EDGE ( 'NONE', *, *, #89603, .T. ) ;
#47957=VECTOR ( 'NONE', #52651, 1000.000000000000000 ) ;
#47969=LINE ( 'NONE', #75705, #59379 ) ;
#48028=ORIENTED_EDGE ( 'NONE', *, *, #11675, .T. ) ;
#48030=ORIENTED_EDGE ( 'NONE', *, *, #67572, .T. ) ;
#48052=CARTESIAN_POINT ( 'NONE',  ( 148.0533267522752112, 0.000000000000000000, 160.2664750769284865 ) ) ;
#48058=CARTESIAN_POINT ( 'NONE',  ( 31.75000000000000000, 8.255000000000000782, 3.174999999999999822 ) ) ;
#48064=CARTESIAN_POINT ( 'NONE',  ( 109.9216266489743248, 47.43999764421818099, 70.44375787698940883 ) ) ;
#48077=ORIENTED_EDGE ( 'NONE', *, *, #70288, .T. ) ;
#48087=CARTESIAN_POINT ( 'NONE',  ( -160.2664750769294812, 0.000000000000000000, -148.0533267522755807 ) ) ;
#48107=DIRECTION ( 'NONE',  ( 0.000000000000000000, 0.000000000000000000, -1.000000000000000000 ) ) ;
#48128=CARTESIAN_POINT ( 'NONE',  ( 5.299065574771610443, 71.00791656138970609, 130.4484248277202880 ) ) ;
#48136=CARTESIAN_POINT ( 'NONE',  ( 120.7609492062753276, 46.70542043813176036, -49.61561143115795858 ) ) ;
#48160=CARTESIAN_POINT ( 'NONE',  ( 196.2150000000000034, 43.68799999999999528, 57.14999999999999858 ) ) ;
#48175=PLANE ( 'NONE',  #77839 ) ;
#48181=SURFACE_SIDE_STYLE ('',( #36380 ) ) ;
#48182=DIRECTION ( 'NONE',  ( 0.000000000000000000, -1.000000000000000000, 0.000000000000000000 ) ) ;
#48189=DIRECTION ( 'NONE',  ( 0.000000000000000000, -1.000000000000000000, 0.000000000000000000 ) ) ;
#48191=ORIENTED_EDGE ( 'NONE', *, *, #8690, .F. ) ;
#48196=CARTESIAN_POINT ( 'NONE',  ( -194.1576000000000022, 101.5999999999999943, 114.2999999999999972 ) ) ;
#48205=CARTESIAN_POINT ( 'NONE',  ( 173.9900000000000091, 20.32000000000000028, -71.37400000000000944 ) ) ;
#48217=LINE ( 'NONE', #70488, #48688 ) ;
#48242=ORIENTED_EDGE ( 'NONE', *, *, #57070, .T. ) ;
#48246=CARTESIAN_POINT ( 'NONE',  ( 160.2664750769289697, 0.000000000000000000, 148.0533267522752112 ) ) ;
#48253=ORIENTED_EDGE ( 'NONE', *, *, #74918, .F. ) ;
#48275=CARTESIAN_POINT ( 'NONE',  ( -22.91753934680783544, 57.39944268860868704, 30.43757021144150343 ) ) ;
#48276=AXIS2_PLACEMENT_3D ( 'NONE', #27836, #40573, #68293 ) ;
#48282=DIRECTION ( 'NONE',  ( 0.000000000000000000, 0.000000000000000000, 1.000000000000000000 ) ) ;
#48297=DIRECTION ( 'NONE',  ( 0.000000000000000000, 0.000000000000000000, -1.000000000000000000 ) ) ;
#48299=PLANE ( 'NONE',  #15246 ) ;
#48316=ORIENTED_EDGE ( 'NONE', *, *, #22220, .F. ) ;
#48322=DIRECTION ( 'NONE',  ( 0.000000000000000000, 0.000000000000000000, 1.000000000000000000 ) ) ;
#48323=LINE ( 'NONE', #76059, #27680 ) ;
#48355=LINE ( 'NONE', #22050, #59533 ) ;
#48356=CARTESIAN_POINT ( 'NONE',  ( -126.0395364549222137, 66.02220425850067897, 34.04284698069740500 ) ) ;
#48373=VERTEX_POINT ( 'NONE', #86571 ) ;
#48376=EDGE_LOOP ( 'NONE', ( #44498, #60450, #89097, #46176 ) ) ;
#48382=CARTESIAN_POINT ( 'NONE',  ( -10.48803521384346737, 75.38805513179248408, 130.1340587520734857 ) ) ;
#48392=CARTESIAN_POINT ( 'NONE',  ( 196.2150000000000034, 30.98800000000000310, 44.45000000000000284 ) ) ;
#48422=DIRECTION ( 'NONE',  ( 0.000000000000000000, -1.000000000000000000, 0.000000000000000000 ) ) ;
#48446=VERTEX_POINT ( 'NONE', #45634 ) ;
#48476=ORIENTED_EDGE ( 'NONE', *, *, #75319, .T. ) ;
#48497=CARTESIAN_POINT ( 'NONE',  ( 109.3101629130975709, 52.31002220769687483, 71.38747593275114411 ) ) ;
#48510=EDGE_CURVE ( 'NONE', #63113, #36552, #50057, .T. ) ;
#48513=ADVANCED_FACE ( 'NONE', ( #54687 ), #4786, .F. ) ;
#48515=CYLINDRICAL_SURFACE ( 'NONE', #74255, 34.13125000000000142 ) ;
#48559=CARTESIAN_POINT ( 'NONE',  ( 183.5150000000000148, 53.21300000000000097, 59.96543552338529537 ) ) ;
#48572=CARTESIAN_POINT ( 'NONE',  ( 10.56424515663473507, 75.50111803887961059, 130.1278827369076794 ) ) ;
#48580=CARTESIAN_POINT ( 'NONE',  ( 123.8510197158557418, 45.44641352664827849, -41.30202659462528203 ) ) ;
#48581=ORIENTED_EDGE ( 'NONE', *, *, #43442, .F. ) ;
#48599=SHAPE_REPRESENTATION ( 'Rotary Table Central Base', ( #50656 ), #10078 ) ;
#48624=DIRECTION ( 'NONE',  ( 0.000000000000000000, -1.000000000000000000, 0.000000000000000000 ) ) ;
#48643=VECTOR ( 'NONE', #88129, 1000.000000000000000 ) ;
#48671=CARTESIAN_POINT ( 'NONE',  ( 148.0533267522749838, 0.000000000000000000, -160.2664750769289697 ) ) ;
#48672=CYLINDRICAL_SURFACE ( 'NONE', #49245, 25.39999999999999858 ) ;
#48676=ORIENTED_EDGE ( 'NONE', *, *, #71034, .F. ) ;
#48681=LINE ( 'NONE', #42762, #6993 ) ;
#48688=VECTOR ( 'NONE', #8719, 1000.000000000000000 ) ;
#48708=CARTESIAN_POINT ( 'NONE',  ( -57.91199999999999903, 101.5999999999999943, 178.6098374884404905 ) ) ;
#48736=DIRECTION ( 'NONE',  ( 0.000000000000000000, 0.000000000000000000, 1.000000000000000000 ) ) ;
#48738=DIRECTION ( 'NONE',  ( -7.497410362015770371E-15, 0.000000000000000000, 1.000000000000000000 ) ) ;
#48758=CARTESIAN_POINT ( 'NONE',  ( -141.3509999999999991, 20.32000000000000028, 141.3509999999999991 ) ) ;
#48785=CARTESIAN_POINT ( 'NONE',  ( 0.000000000000000000, 95.00619999999999266, 0.000000000000000000 ) ) ;
#48810=CARTESIAN_POINT ( 'NONE',  ( -122.5031070146980028, 73.82525647761227106, 45.14392447952047149 ) ) ;
#48834=ORIENTED_EDGE ( 'NONE', *, *, #85066, .F. ) ;
#48836=CARTESIAN_POINT ( 'NONE',  ( -12.62696438262051046, 80.95609589054741662, 129.9443975344997284 ) ) ;
#48837=DIRECTION ( 'NONE',  ( 0.000000000000000000, -1.000000000000000000, 0.000000000000000000 ) ) ;
#48899=ADVANCED_FACE ( 'NONE', ( #44652 ), #9705, .F. ) ;
#48994=AXIS2_PLACEMENT_3D ( 'NONE', #28067, #61687, #68971 ) ;
#48999=VECTOR ( 'NONE', #18495, 1000.000000000000000 ) ;
#49007=LINE ( 'NONE', #61750, #53635 ) ;
#49009=LINE ( 'NONE', #48559, #61469 ) ;
#49012=ORIENTED_EDGE ( 'NONE', *, *, #22276, .T. ) ;
#49021=CARTESIAN_POINT ( 'NONE',  ( 7.305616351080206350, 72.16134662172612479, 130.3514124915961645 ) ) ;
#49050=VECTOR ( 'NONE', #66248, 1000.000000000000000 ) ;
#49067=CIRCLE ( 'NONE', #25877, 160.4955849403809793 ) ;
#49084=CARTESIAN_POINT ( 'NONE',  ( -194.1576000000000022, 20.32000000000000028, -9.525000000000000355 ) ) ;
#49104=DIRECTION ( 'NONE',  ( 0.000000000000000000, -1.000000000000000000, 0.000000000000000000 ) ) ;
#49120=DIRECTION ( 'NONE',  ( 0.000000000000000000, 0.000000000000000000, 1.000000000000000000 ) ) ;
#49141=ADVANCED_FACE ( 'NONE', ( #27348 ), #8256, .F. ) ;
#49163=AXIS2_PLACEMENT_3D ( 'NONE', #80375, #65823, #31303 ) ;
#49174=VECTOR ( 'NONE', #14299, 1000.000000000000000 ) ;
#49182=CARTESIAN_POINT ( 'NONE',  ( 12.69999999999999929, 82.54999999999999716, 129.9368274816650057 ) ) ;
#49213=EDGE_LOOP ( 'NONE', ( #85781, #87164 ) ) ;
#49245=AXIS2_PLACEMENT_3D ( 'NONE', #76405, #21452, #49120 ) ;
#49250=EDGE_CURVE ( 'NONE', #5960, #849, #48217, .T. ) ;
#49267=CARTESIAN_POINT ( 'NONE',  ( -120.3273848475766954, 74.62250637307523959, 50.66261013073812336 ) ) ;
#49270=AXIS2_PLACEMENT_3D ( 'NONE', #25694, #62001, #25243 ) ;
#49309=CARTESIAN_POINT ( 'NONE',  ( -187.8075999999999794, 20.32000000000000028, -6.349999999999999645 ) ) ;
#49312=DIRECTION ( 'NONE',  ( 0.000000000000000000, 0.000000000000000000, -1.000000000000000000 ) ) ;
#49325=FACE_OUTER_BOUND ( 'NONE', #65222, .T. ) ;
#49351=CARTESIAN_POINT ( 'NONE',  ( -11.42323817349576309, 88.11531169846917066, 130.0554870647972905 ) ) ;
#49354=EDGE_LOOP ( 'NONE', ( #21599, #68565, #73693, #51165 ) ) ;
#49375=DIRECTION ( 'NONE',  ( 7.340987889507870014E-14, 0.000000000000000000, 1.000000000000000000 ) ) ;
#49385=CARTESIAN_POINT ( 'NONE',  ( -109.6863455812695776, 48.91650121126127715, 70.80801475970909564 ) ) ;
#49398=CARTESIAN_POINT ( 'NONE',  ( -1.415542646969860267E-16, 70.24203434096102683, 38.10000000000000142 ) ) ;
#49409=CARTESIAN_POINT ( 'NONE',  ( 109.5618042869657387, 49.74144395212335468, 71.00059892473528578 ) ) ;
#49412=DIRECTION ( 'NONE',  ( -1.000000000000000000, 0.000000000000000000, -1.531877379624855416E-14 ) ) ;
#49434=CARTESIAN_POINT ( 'NONE',  ( -179.6205029264235122, 101.5999999999999943, 123.8612349545196025 ) ) ;
#49436=AXIS2_PLACEMENT_3D ( 'NONE', #10604, #2473, #57869 ) ;
#49445=CARTESIAN_POINT ( 'NONE',  ( -179.8898777604659927, 0.000000000000000000, -123.4696824136383952 ) ) ;
#49458=CARTESIAN_POINT ( 'NONE',  ( 183.5150000000000148, 21.46300000000000097, 59.96543552338529537 ) ) ;
#49468=EDGE_LOOP ( 'NONE', ( #4120, #10933, #23462, #28005 ) ) ;
#49476=LINE ( 'NONE', #70851, #12438 ) ;
#49517=ORIENTED_EDGE ( 'NONE', *, *, #62799, .T. ) ;
#49521=FACE_OUTER_BOUND ( 'NONE', #13483, .T. ) ;
#49524=LINE ( 'NONE', #35452, #53081 ) ;
#49530=FILL_AREA_STYLE_COLOUR ( '', #20259 ) ;
#49536=ORIENTED_EDGE ( 'NONE', *, *, #89872, .T. ) ;
#49576=ORIENTED_EDGE ( 'NONE', *, *, #17502, .F. ) ;
#49598=DIRECTION ( 'NONE',  ( 0.000000000000000000, -1.000000000000000000, 0.000000000000000000 ) ) ;
#49606=EDGE_CURVE ( 'NONE', #16666, #47179, #60404, .T. ) ;
#49608=VERTEX_POINT ( 'NONE', #33161 ) ;
#49633=CARTESIAN_POINT ( 'NONE',  ( 12.28931626436909497, 79.31803562664185847, 129.9766762937439069 ) ) ;
#49656=ADVANCED_FACE ( 'NONE', ( #55369 ), #63097, .F. ) ;
#49664=CARTESIAN_POINT ( 'NONE',  ( 23.27731929905161223, 53.97500000000000142, 30.16249999999999076 ) ) ;
#49684=DIRECTION ( 'NONE',  ( 0.000000000000000000, 0.000000000000000000, 1.000000000000000000 ) ) ;
#49689=CIRCLE ( 'NONE', #13576, 8.636000000000004562 ) ;
#49708=ORIENTED_EDGE ( 'NONE', *, *, #45114, .F. ) ;
#49726=ORIENTED_EDGE ( 'NONE', *, *, #45348, .F. ) ;
#49763=DIRECTION ( 'NONE',  ( 0.000000000000000000, 0.000000000000000000, -1.000000000000000000 ) ) ;
#49765=LINE ( 'NONE', #29792, #43492 ) ;
#49840=ORIENTED_EDGE ( 'NONE', *, *, #13993, .T. ) ;
#49847=CARTESIAN_POINT ( 'NONE',  ( 12.65714626781473839, 68.30105204775735217, 35.94211041470738621 ) ) ;
#49848=VECTOR ( 'NONE', #87179, 1000.000000000000114 ) ;
#49875=ADVANCED_FACE ( 'NONE', ( #82016 ), #74288, .F. ) ;
#49891=ORIENTED_EDGE ( 'NONE', *, *, #242, .T. ) ;
#49913=FACE_BOUND ( 'NONE', #39804, .T. ) ;
#49921=DIRECTION ( 'NONE',  ( -1.000000000000000000, 0.000000000000000000, 0.000000000000000000 ) ) ;
#49925=CARTESIAN_POINT ( 'NONE',  ( 173.9900000000000091, 20.32000000000000028, -71.37400000000000944 ) ) ;
#49931=ORIENTED_EDGE ( 'NONE', *, *, #45348, .T. ) ;
#49997=CIRCLE ( 'NONE', #5010, 218.1859999999999786 ) ;
#50001=EDGE_CURVE ( 'NONE', #25538, #67615, #20224, .T. ) ;
#50057=CIRCLE ( 'NONE', #57321, 6.349999999999999645 ) ;
#50095=DIRECTION ( 'NONE',  ( 0.000000000000000000, 0.000000000000000000, 1.000000000000000000 ) ) ;
#50103=VECTOR ( 'NONE', #63288, 1000.000000000000000 ) ;
#50108=EDGE_CURVE ( 'NONE', #29697, #42257, #656, .T. ) ;
#50131=CARTESIAN_POINT ( 'NONE',  ( -148.0533267522759786, 20.32000000000000028, -160.2664750769289697 ) ) ;
#50151=ORIENTED_EDGE ( 'NONE', *, *, #50001, .F. ) ;
#50161=EDGE_LOOP ( 'NONE', ( #55299, #14057, #33962, #64365 ) ) ;
#50183=ADVANCED_FACE ( 'NONE', ( #79224 ), #72835, .F. ) ;
#50193=AXIS2_PLACEMENT_3D ( 'NONE', #24676, #87357, #72392 ) ;
#50200=CARTESIAN_POINT ( 'NONE',  ( -1.415542646969860267E-16, 70.24203434096102683, 38.10000000000000142 ) ) ;
#50234=EDGE_CURVE ( 'NONE', #32410, #54956, #25570, .T. ) ;
#50265=AXIS2_PLACEMENT_3D ( 'NONE', #572, #135, #58231 ) ;
#50273=EDGE_CURVE ( 'NONE', #88226, #63113, #66908, .T. ) ;
#50279=CARTESIAN_POINT ( 'NONE',  ( -110.0436475921183899, 47.06665061967962060, 70.25164585318982802 ) ) ;
#50288=ORIENTED_EDGE ( 'NONE', *, *, #61025, .T. ) ;
#50296=CARTESIAN_POINT ( 'NONE',  ( 2.759391577539827445, 70.18407359651233435, 38.02468864519824621 ) ) ;
#50338=CARTESIAN_POINT ( 'NONE',  ( 0.000000000000000000, 101.5999999999999943, 0.000000000000000000 ) ) ;
#50346=DIRECTION ( 'NONE',  ( 0.000000000000000000, -1.000000000000000000, 0.000000000000000000 ) ) ;
#50363=DIRECTION ( 'NONE',  ( 0.000000000000000000, -1.000000000000000000, 0.000000000000000000 ) ) ;
#50375=DIRECTION ( 'NONE',  ( 0.000000000000000000, 0.000000000000000000, -1.000000000000000000 ) ) ;
#50402=CIRCLE ( 'NONE', #12692, 1.523999999999053889 ) ;
#50403=DIRECTION ( 'NONE',  ( 0.000000000000000000, -1.000000000000000000, 0.000000000000000000 ) ) ;
#50405=ORIENTED_EDGE ( 'NONE', *, *, #17305, .F. ) ;
#50409=CARTESIAN_POINT ( 'NONE',  ( 173.9900000000000091, 0.000000000000000000, 131.6533725204182019 ) ) ;
#50417=CARTESIAN_POINT ( 'NONE',  ( 126.1740464204627301, 65.29148310750557016, 33.54086098101917202 ) ) ;
#50427=ORIENTED_EDGE ( 'NONE', *, *, #19670, .F. ) ;
#50487=VECTOR ( 'NONE', #64579, 1000.000000000000000 ) ;
#50495=MANIFOLD_SOLID_BREP ( 'Stock-BR-Y-104-1', #25647 ) ;
#50497=ORIENTED_EDGE ( 'NONE', *, *, #43447, .F. ) ;
#50502=CARTESIAN_POINT ( 'NONE',  ( 0.000000000000000000, 11.42999999999999972, 0.000000000000000000 ) ) ;
#50519=EDGE_CURVE ( 'NONE', #6845, #7688, #28536, .T. ) ;
#50563=CARTESIAN_POINT ( 'NONE',  ( 6.579133765263863509, 93.41355262086047162, 130.3901338211574057 ) ) ;
#50564=VERTEX_POINT ( 'NONE', #81357 ) ;
#50567=DIRECTION ( 'NONE',  ( 0.000000000000000000, 0.000000000000000000, 1.000000000000000000 ) ) ;
#50635=ORIENTED_EDGE ( 'NONE', *, *, #2286, .F. ) ;
#50638=VECTOR ( 'NONE', #45053, 1000.000000000000000 ) ;
#50648=CARTESIAN_POINT ( 'NONE',  ( 3.175000000000355094, 17.78000000000000114, 33.98325472291460159 ) ) ;
#50656=AXIS2_PLACEMENT_3D ( 'NONE', #89656, #19265, #5642 ) ;
#50677=AXIS2_PLACEMENT_3D ( 'NONE', #80595, #4728, #33768 ) ;
#50695=CARTESIAN_POINT ( 'NONE',  ( 0.000000000000000000, 95.00619999999999266, 38.10000000000000142 ) ) ;
#50700=CARTESIAN_POINT ( 'NONE',  ( -10.61352881085396049, 89.52455520069554495, 130.1238749127236360 ) ) ;
#50740=CARTESIAN_POINT ( 'NONE',  ( -109.6785575274413418, 48.96444734860763504, 70.82007752391335487 ) ) ;
#50743=EDGE_CURVE ( 'NONE', #42621, #5363, #69493, .T. ) ;
#50786=LINE ( 'NONE', #63524, #78481 ) ;
#50796=ORIENTED_EDGE ( 'NONE', *, *, #27023, .T. ) ;
#50822=EDGE_LOOP ( 'NONE', ( #1476, #87264, #9923, #40008 ) ) ;
#50823=FACE_OUTER_BOUND ( 'NONE', #15564, .T. ) ;
#50839=ORIENTED_EDGE ( 'NONE', *, *, #23192, .F. ) ;
#50841=ORIENTED_EDGE ( 'NONE', *, *, #81037, .T. ) ;
#50843=CARTESIAN_POINT ( 'NONE',  ( 125.1260334383333657, 49.36275571881125046, -37.26066279344849619 ) ) ;
#50867=DIRECTION ( 'NONE',  ( 7.340987889507870014E-14, 0.000000000000000000, 1.000000000000000000 ) ) ;
#50869=DIRECTION ( 'NONE',  ( 1.000000000000000000, 0.000000000000000000, -2.761895400282000234E-15 ) ) ;
#50871=CARTESIAN_POINT ( 'NONE',  ( 123.1260477991215367, 73.24606306481838658, 43.41488809734197929 ) ) ;
#50881=ORIENTED_EDGE ( 'NONE', *, *, #5381, .F. ) ;
#50891=DIRECTION ( 'NONE',  ( 0.000000000000000000, -1.000000000000000000, 0.000000000000000000 ) ) ;
#50893=CARTESIAN_POINT ( 'NONE',  ( 0.000000000000000000, 2.031999999999865025, 0.000000000000000000 ) ) ;
#50901=EDGE_CURVE ( 'NONE', #4177, #25538, #30103, .T. ) ;
#50903=ADVANCED_FACE ( 'NONE', ( #73053 ), #84931, .F. ) ;
#50905=VECTOR ( 'NONE', #5738, 1000.000000000000000 ) ;
#50975=EDGE_LOOP ( 'NONE', ( #37763, #44868, #82279, #40110 ) ) ;
#50981=ORIENTED_EDGE ( 'NONE', *, *, #10689, .F. ) ;
#51016=B_SPLINE_CURVE_WITH_KNOTS ( 'NONE', 3,
 ( #49182, #70095, #42366, #35563, #49633, #29218, #77359, #56905, #14244, #16041, #64186, #1960, #42813, #29656, #28297, #599, #43718, #70552, #57348, #85089, #41920, #69651, #7420, #55989, #82698, #48572, #82250, #5487, #74965, #61322, #47686, #55832, #62223, #9, #60880, #33182, #14080, #54933, #81795, #27709, #49021, #75421, #75861, #76756, #13634, #19548, #68155, #89044, #42219, #69047, #83141, #20458, #14541, #48128, #41318, #13195, #20899, #21347, #68607, #76307, #55386, #69499, #6814, #34517, #41765 ),
 .UNSPECIFIED., .F., .F.,
 ( 4, 2, 2, 2, 1, 1, 1, 2, 2, 2, 2, 1, 1, 1, 1, 1, 2, 2, 2, 2, 2, 2, 2, 2, 2, 1, 1, 1, 1, 2, 2, 2, 2, 1, 1, 1, 2, 2, 2, 4 ),
 ( 0.000000000000000000, 0.1249999999995733135, 0.1874999999993589295, 0.2187499999992517374, 0.2343749999991982247, 0.2421874999991724120, 0.2460937499991595057, 0.2480468749991530386, 0.2499999999991465716, 0.3124999999989560573, 0.3437499999988598010, 0.3593749999988124499, 0.3671874999987889132, 0.3710937499987771448, 0.3730468749987704835, 0.3740234374987679300, 0.3745117187487666532, 0.3749999999987653210, 0.4374999999987978505, 0.4687499999988149479, 0.4843749999988227195, 0.4999999999988304911, 0.5624999999988645749, 0.5937499999988823385, 0.6093749999988912203, 0.6171874999988957722, 0.6210937499988979926, 0.6230468749988992139, 0.6240234374989007682, 0.6245117187489016564, 0.6249999999989025445, 0.6874999999990687449, 0.7187499999991523447, 0.7343749999991942001, 0.7421874999992156274, 0.7460937499992262856, 0.7480468749992316146, 0.7499999999992368327, 0.8749999999996184163, 1.000000000000000000 ),
 .UNSPECIFIED. ) ;
#51019=DIRECTION ( 'NONE',  ( 0.000000000000000000, 0.000000000000000000, 1.000000000000000000 ) ) ;
#51030=DIRECTION ( 'NONE',  ( -1.000000000000000000, 0.000000000000000000, 6.982966722218760189E-15 ) ) ;
#51047=CARTESIAN_POINT ( 'NONE',  ( 0.000000000000000000, 12.26999999999999957, 0.000000000000000000 ) ) ;
#51056=VERTEX_POINT ( 'NONE', #31721 ) ;
#51061=ORIENTED_EDGE ( 'NONE', *, *, #31574, .T. ) ;
#51077=CARTESIAN_POINT ( 'NONE',  ( 1.154229608196380665E-15, 2.269999999999994245, 9.425000000000000711 ) ) ;
#51084=EDGE_CURVE ( 'NONE', #60648, #24397, #82318, .T. ) ;
#51142=CARTESIAN_POINT ( 'NONE',  ( -5.751998507614636047, 93.87463779977233003, 130.4293086530511232 ) ) ;
#51148=CARTESIAN_POINT ( 'NONE',  ( 119.5843592605237120, 52.73749999999999716, -52.38749999999991758 ) ) ;
#51160=CYLINDRICAL_SURFACE ( 'NONE', #30755, 7.937500000000000000 ) ;
#51165=ORIENTED_EDGE ( 'NONE', *, *, #7221, .F. ) ;
#51180=VERTEX_POINT ( 'NONE', #19297 ) ;
#51185=EDGE_CURVE ( 'NONE', #23113, #54222, #74703, .T. ) ;
#51188=CARTESIAN_POINT ( 'NONE',  ( 20.45523698819324565, 62.82274409087659706, 32.14693258707937673 ) ) ;
#51190=CARTESIAN_POINT ( 'NONE',  ( 0.000000000000000000, 125.7300000000000040, 0.000000000000000000 ) ) ;
#51208=DIRECTION ( 'NONE',  ( 1.000000000000000000, 0.000000000000000000, 2.108231265501709878E-16 ) ) ;
#51213=ORIENTED_EDGE ( 'NONE', *, *, #70242, .T. ) ;
#51225=CYLINDRICAL_SURFACE ( 'NONE', #71885, 218.1859999999999786 ) ;
#51236=CIRCLE ( 'NONE', #23717, 154.1697486074984909 ) ;
#51243=DIRECTION ( 'NONE',  ( 0.000000000000000000, -1.000000000000000000, 0.000000000000000000 ) ) ;
#51247=CARTESIAN_POINT ( 'NONE',  ( 131.3179999999999836, 53.97500000000000142, 71.43750000000000000 ) ) ;
#51250=PLANE ( 'NONE',  #26177 ) ;
#51256=CARTESIAN_POINT ( 'NONE',  ( 3.174999999999879918, 24.56180297284579694, -33.98325472291465132 ) ) ;
#51260=CARTESIAN_POINT ( 'NONE',  ( -215.9000000000000057, 101.5999999999999943, -45.33899999999999864 ) ) ;
#51280=ORIENTED_EDGE ( 'NONE', *, *, #30029, .T. ) ;
#51287=CARTESIAN_POINT ( 'NONE',  ( 0.000000000000000000, 95.00619999999999266, 0.000000000000000000 ) ) ;
#51296=CARTESIAN_POINT ( 'NONE',  ( 111.6857113302616824, 65.94691145059840665, 67.61047547054599249 ) ) ;
#51300=ORIENTED_EDGE ( 'NONE', *, *, #2533, .T. ) ;
#51337=VERTEX_POINT ( 'NONE', #28800 ) ;
#51350=ORIENTED_EDGE ( 'NONE', *, *, #20271, .F. ) ;
#51362=DIRECTION ( 'NONE',  ( 0.000000000000000000, 1.000000000000000000, 0.000000000000000000 ) ) ;
#51395=EDGE_CURVE ( 'NONE', #66654, #58230, #83771, .T. ) ;
#51461=CARTESIAN_POINT ( 'NONE',  ( -33.98325472291465132, 24.56180297284579694, -3.174999999999764899 ) ) ;
#51498=CARTESIAN_POINT ( 'NONE',  ( -126.4537727773635254, 63.48808950043785870, 32.47212463199235088 ) ) ;
#51500=VERTEX_POINT ( 'NONE', #37395 ) ;
#51515=CARTESIAN_POINT ( 'NONE',  ( -57.91199999999999903, 0.000000000000000000, 191.3008000794699797 ) ) ;
#51516=ORIENTED_EDGE ( 'NONE', *, *, #72118, .T. ) ;
#51520=EDGE_CURVE ( 'NONE', #41931, #43342, #47529, .T. ) ;
#51537=DIRECTION ( 'NONE',  ( 0.000000000000000000, 0.000000000000000000, -1.000000000000000000 ) ) ;
#51548=CYLINDRICAL_SURFACE ( 'NONE', #14637, 6.349999999999999645 ) ;
#51574=DIRECTION ( 'NONE',  ( 1.000000000000000000, 0.000000000000000000, 0.000000000000000000 ) ) ;
#51576=AXIS2_PLACEMENT_3D ( 'NONE', #45403, #73121, #18158 ) ;
#51580=CARTESIAN_POINT ( 'NONE',  ( 3.944304526105059924E-28, 95.25000000000000000, 130.5560000000000116 ) ) ;
#51588=PLANE ( 'NONE',  #43817 ) ;
#51598=EDGE_LOOP ( 'NONE', ( #70620, #46705 ) ) ;
#51627=ORIENTED_EDGE ( 'NONE', *, *, #19558, .F. ) ;
#51661=ORIENTED_EDGE ( 'NONE', *, *, #85632, .T. ) ;
#51663=VERTEX_POINT ( 'NONE', #37811 ) ;
#51666=CARTESIAN_POINT ( 'NONE',  ( 0.000000000000000000, 44.45000000000000284, 0.000000000000000000 ) ) ;
#51672=EDGE_CURVE ( 'NONE', #20334, #10389, #23312, .T. ) ;
#51698=DIRECTION ( 'NONE',  ( 0.000000000000000000, 0.000000000000000000, -1.000000000000000000 ) ) ;
#51702=ORIENTED_EDGE ( 'NONE', *, *, #82809, .F. ) ;
#51707=DIRECTION ( 'NONE',  ( -2.913971193241881161E-15, 0.000000000000000000, 1.000000000000000000 ) ) ;
#51744=CARTESIAN_POINT ( 'NONE',  ( 109.8326081572954251, 59.86973552847310742, 70.58103716012563211 ) ) ;
#51749=ORIENTED_EDGE ( 'NONE', *, *, #25368, .F. ) ;
#51758=CARTESIAN_POINT ( 'NONE',  ( 0.000000000000000000, 8.255000000000000782, 0.000000000000000000 ) ) ;
#51770=DIRECTION ( 'NONE',  ( -2.505701470911820065E-15, 0.000000000000000000, -1.000000000000000000 ) ) ;
#51775=AXIS2_PLACEMENT_3D ( 'NONE', #8111, #51208, #37159 ) ;
#51817=CARTESIAN_POINT ( 'NONE',  ( 75.61066417432020614, 101.5999999999999943, 189.7379999999999995 ) ) ;
#51867=AXIS2_PLACEMENT_3D ( 'NONE', #80828, #39469, #44934 ) ;
#51881=CARTESIAN_POINT ( 'NONE',  ( 4.354213876134587657, 94.48073875936546528, 130.4833586261829055 ) ) ;
#51892=VERTEX_POINT ( 'NONE', #74115 ) ;
#51909=ORIENTED_EDGE ( 'NONE', *, *, #63824, .F. ) ;
#51911=EDGE_CURVE ( 'NONE', #54222, #48446, #77260, .T. ) ;
#51915=CARTESIAN_POINT ( 'NONE',  ( 0.000000000000000000, 11.42999999999999972, 0.000000000000000000 ) ) ;
#51927=LINE ( 'NONE', #71971, #14488 ) ;
#51931=AXIS2_PLACEMENT_3D ( 'NONE', #41966, #76961, #48322 ) ;
#52014=AXIS2_PLACEMENT_3D ( 'NONE', #68962, #5395, #7187 ) ;
#52020=VERTEX_POINT ( 'NONE', #72682 ) ;
#52024=DIRECTION ( 'NONE',  ( 0.000000000000000000, 1.000000000000000000, 0.000000000000000000 ) ) ;
#52028=ADVANCED_FACE ( 'NONE', ( #30007 ), #23218, .T. ) ;
#52046=VECTOR ( 'NONE', #12761, 1000.000000000000000 ) ;
#52055=AXIS2_PLACEMENT_3D ( 'NONE', #34844, #5810, #88481 ) ;
#52085=CARTESIAN_POINT ( 'NONE',  ( -179.8898777604655095, 20.32000000000000028, -12.69999999999999929 ) ) ;
#52093=ADVANCED_FACE ( 'NONE', ( #30453 ), #16378, .F. ) ;
#52101=VECTOR ( 'NONE', #48624, 1000.000000000000000 ) ;
#52124=CARTESIAN_POINT ( 'NONE',  ( 196.2150000000000034, 37.33800000000000097, 60.32499999999999574 ) ) ;
#52135=CARTESIAN_POINT ( 'NONE',  ( 120.5286047550879260, 58.23918486294396502, -50.17733349311141211 ) ) ;
#52170=DIRECTION ( 'NONE',  ( 0.000000000000000000, 0.000000000000000000, 1.000000000000000000 ) ) ;
#52177=CARTESIAN_POINT ( 'NONE',  ( 117.7358725014768481, 73.84217107435090099, 56.42336322934903592 ) ) ;
#52184=CARTESIAN_POINT ( 'NONE',  ( 131.3179999999999836, 37.33800000000000097, 50.79999999999999716 ) ) ;
#52262=CARTESIAN_POINT ( 'NONE',  ( -3.174999999999644995, 24.56180297284579694, 33.98325472291465132 ) ) ;
#52281=ORIENTED_EDGE ( 'NONE', *, *, #69624, .T. ) ;
#52282=VECTOR ( 'NONE', #38606, 1000.000000000000114 ) ;
#52302=EDGE_CURVE ( 'NONE', #23986, #19042, #64860, .T. ) ;
#52309=EDGE_CURVE ( 'NONE', #17548, #5232, #29448, .T. ) ;
#52340=EDGE_CURVE ( 'NONE', #11616, #21936, #3517, .T. ) ;
#52381=CIRCLE ( 'NONE', #88746, 8.636000000000004562 ) ;
#52403=LINE ( 'NONE', #78394, #61331 ) ;
#52404=DIRECTION ( 'NONE',  ( 0.7071067811865604513, 0.000000000000000000, -0.7071067811865345831 ) ) ;
#52433=EDGE_LOOP ( 'NONE', ( #85793, #74666, #44728, #51061 ) ) ;
#52435=EDGE_CURVE ( 'NONE', #85180, #21659, #33009, .T. ) ;
#52436=DIRECTION ( 'NONE',  ( 1.000000000000000000, 0.000000000000000000, 2.108231265501709878E-16 ) ) ;
#52452=VECTOR ( 'NONE', #3424, 1000.000000000000000 ) ;
#52463=CARTESIAN_POINT ( 'NONE',  ( 126.8161134320454977, 48.06767884207233976, 31.02493203361878926 ) ) ;
#52489=LINE ( 'NONE', #45245, #80534 ) ;
#52506=DIRECTION ( 'NONE',  ( 1.000000000000000000, 0.000000000000000000, 0.000000000000000000 ) ) ;
#52538=VERTEX_POINT ( 'NONE', #13471 ) ;
#52563=EDGE_LOOP ( 'NONE', ( #64407, #44384, #50796, #309 ) ) ;
#52564=EDGE_CURVE ( 'NONE', #35850, #6945, #17005, .T. ) ;
#52575=CARTESIAN_POINT ( 'NONE',  ( 124.2933722748468028, 59.28198175267112191, -39.95096659757145829 ) ) ;
#52620=CARTESIAN_POINT ( 'NONE',  ( 110.4077240393726527, 62.31375596498891412, 69.67785885149439196 ) ) ;
#52633=VERTEX_POINT ( 'NONE', #57028 ) ;
#52634=DIRECTION ( 'NONE',  ( 0.000000000000000000, -1.000000000000000000, 0.000000000000000000 ) ) ;
#52645=EDGE_CURVE ( 'NONE', #20262, #74824, #64315, .T. ) ;
#52649=DIRECTION ( 'NONE',  ( 0.000000000000000000, 1.000000000000000000, 0.000000000000000000 ) ) ;
#52651=DIRECTION ( 'NONE',  ( 0.000000000000000000, -1.000000000000000000, 0.000000000000000000 ) ) ;
#52655=ORIENTED_EDGE ( 'NONE', *, *, #8074, .F. ) ;
#52690=CARTESIAN_POINT ( 'NONE',  ( 0.000000000000000000, 95.00619999999999266, 0.000000000000000000 ) ) ;
#52692=ADVANCED_FACE ( 'NONE', ( #24314 ), #2975, .T. ) ;
#52722=DIRECTION ( 'NONE',  ( -2.671820169801660301E-13, 0.000000000000000000, 1.000000000000000000 ) ) ;
#52768=ORIENTED_EDGE ( 'NONE', *, *, #27130, .F. ) ;
#52794=ORIENTED_EDGE ( 'NONE', *, *, #9622, .T. ) ;
#52795=ORIENTED_EDGE ( 'NONE', *, *, #68415, .T. ) ;
#52832=CARTESIAN_POINT ( 'NONE',  ( -17.75984020069129343, 65.55676468737539153, 33.71262514113522712 ) ) ;
#52861=ORIENTED_EDGE ( 'NONE', *, *, #28563, .F. ) ;
#52885=AXIS2_PLACEMENT_3D ( 'NONE', #60395, #61296, #89017 ) ;
#52893=LINE ( 'NONE', #88825, #84446 ) ;
#52913=CARTESIAN_POINT ( 'NONE',  ( -110.5312426757802626, 62.76878794380225202, 69.48247424316639353 ) ) ;
#52984=DIRECTION ( 'NONE',  ( 0.000000000000000000, 0.000000000000000000, 1.000000000000000000 ) ) ;
#53014=CARTESIAN_POINT ( 'NONE',  ( 122.6405678466407352, 60.67261296635635404, -44.76865280868378250 ) ) ;
#53038=VERTEX_POINT ( 'NONE', #15045 ) ;
#53048=VECTOR ( 'NONE', #27707, 1000.000000000000000 ) ;
#53060=CARTESIAN_POINT ( 'NONE',  ( 114.1934708208216307, 70.42029666602465454, 63.28548749111810423 ) ) ;
#53073=DIRECTION ( 'NONE',  ( 0.000000000000000000, 0.000000000000000000, 1.000000000000000000 ) ) ;
#53078=CIRCLE ( 'NONE', #31327, 9.525000000000000355 ) ;
#53081=VECTOR ( 'NONE', #86195, 1000.000000000000000 ) ;
#53083=CIRCLE ( 'NONE', #74917, 34.13125000000000142 ) ;
#53107=DIRECTION ( 'NONE',  ( -1.000000000000000000, 0.000000000000000000, 0.000000000000000000 ) ) ;
#53110=DIRECTION ( 'NONE',  ( 1.000000000000000000, 0.000000000000000000, 1.472650733923983947E-14 ) ) ;
#53118=ADVANCED_FACE ( 'NONE', ( #70008 ), #86323, .F. ) ;
#53137=CIRCLE ( 'NONE', #25614, 218.1859999999999786 ) ;
#53155=EDGE_CURVE ( 'NONE', #86605, #58432, #45402, .T. ) ;
#53159=AXIS2_PLACEMENT_3D ( 'NONE', #59217, #86947, #87836 ) ;
#53178=LINE ( 'NONE', #31873, #76982 ) ;
#53188=( NAMED_UNIT ( * ) SI_UNIT ( $, .STERADIAN. ) SOLID_ANGLE_UNIT ( ) );
#53196=ORIENTED_EDGE ( 'NONE', *, *, #86918, .T. ) ;
#53212=CARTESIAN_POINT ( 'NONE',  ( 10.18556280471778486, 90.13775373083149134, 130.1582303542269017 ) ) ;
#53244=EDGE_CURVE ( 'NONE', #61695, #47090, #3209, .T. ) ;
#53298=EDGE_CURVE ( 'NONE', #72757, #43367, #83170, .T. ) ;
#53304=DIRECTION ( 'NONE',  ( -0.7071067811865739960, 0.000000000000000000, -0.7071067811865210384 ) ) ;
#53320=AXIS2_PLACEMENT_3D ( 'NONE', #43128, #1374, #29526 ) ;
#53326=LINE ( 'NONE', #75608, #57494 ) ;
#53338=EDGE_LOOP ( 'NONE', ( #73380, #9647, #73764, #40523 ) ) ;
#53340=AXIS2_PLACEMENT_3D ( 'NONE', #56238, #76259, #14037 ) ;
#53345=DIRECTION ( 'NONE',  ( 0.000000000000000000, 1.000000000000000000, 0.000000000000000000 ) ) ;
#53378=CARTESIAN_POINT ( 'NONE',  ( -110.7180744603615352, 63.37589224994205495, 69.18472289323493385 ) ) ;
#53407=CYLINDRICAL_SURFACE ( 'NONE', #36058, 6.349999999999997868 ) ;
#53410=FACE_OUTER_BOUND ( 'NONE', #18527, .T. ) ;
#53433=VECTOR ( 'NONE', #62586, 1000.000000000000000 ) ;
#53442=DIRECTION ( 'NONE',  ( 0.000000000000000000, 1.000000000000000000, 0.000000000000000000 ) ) ;
#53447=ORIENTED_EDGE ( 'NONE', *, *, #83652, .F. ) ;
#53463=VECTOR ( 'NONE', #44078, 1000.000000000000000 ) ;
#53472=CARTESIAN_POINT ( 'NONE',  ( 123.0934642905847198, 60.63545122801047427, -43.51030618446090870 ) ) ;
#53492=EDGE_LOOP ( 'NONE', ( #49517, #22461, #6727, #67148 ) ) ;
#53518=CARTESIAN_POINT ( 'NONE',  ( 173.9900000000000091, 37.33800000000000097, 50.79999999999999716 ) ) ;
#53557=EDGE_CURVE ( 'NONE', #89203, #16001, #10354, .T. ) ;
#53568=CARTESIAN_POINT ( 'NONE',  ( 173.9900000000000091, 101.5999999999999943, -71.37400000000000944 ) ) ;
#53617=DIRECTION ( 'NONE',  ( 0.000000000000000000, -1.000000000000000000, 0.000000000000000000 ) ) ;
#53623=VECTOR ( 'NONE', #8437, 1000.000000000000000 ) ;
#53635=VECTOR ( 'NONE', #41306, 1000.000000000000000 ) ;
#53643=CARTESIAN_POINT ( 'NONE',  ( 183.5150000000000148, 21.46300000000000097, 41.63456447661474868 ) ) ;
#53677=VECTOR ( 'NONE', #85871, 1000.000000000000000 ) ;
#53688=CARTESIAN_POINT ( 'NONE',  ( 55.48342271751659638, 20.32000000000000028, 171.1197181046785261 ) ) ;
#53695=B_SPLINE_CURVE_WITH_KNOTS ( 'NONE', 3,
 ( #83590, #7283, #56295, #54940, #56756, #8176, #456, #14549, #75427, #62683, #35869, #63586, #48136, #69507, #68613, #13201, #20907, #910, #13641, #1365, #6374, #27717, #47692, #34969, #42226, #75870, #62231, #48580, #76314, #28150, #76764, #69956, #28609, #34065, #29069, #84040, #21816, #30850, #15448, #85838, #50843, #43119, #57653, #58105, #36777, #44011 ),
 .UNSPECIFIED., .F., .F.,
 ( 4, 2, 2, 2, 2, 2, 2, 2, 2, 2, 2, 2, 2, 2, 2, 2, 2, 2, 2, 2, 2, 2, 4 ),
 ( 1.387778780781445676E-17, 0.001601640810786372163, 0.003203281621572730449, 0.004804922432359089168, 0.005605742837752265492, 0.006406563243145441816, 0.007207383648538618140, 0.008008204053931794464, 0.009609844864718143642, 0.01121148567550449282, 0.01281312648629084373, 0.01361394689168402700, 0.01441476729707721373, 0.01601640810786359934, 0.01681722851325679127, 0.01761804891864998668, 0.01921968972943637402, 0.02002051013482955902, 0.02082133054022275095, 0.02162215094561594289, 0.02242297135100913136, 0.02402461216179551870, 0.02562625297258190604 ),
 .UNSPECIFIED. ) ;
#53779=CARTESIAN_POINT ( 'NONE',  ( 22.90438369314431100, 50.44815651554718983, 30.44723272559076221 ) ) ;
#53809=EDGE_CURVE ( 'NONE', #73841, #58184, #28090, .T. ) ;
#53814=CARTESIAN_POINT ( 'NONE',  ( 3.175000000000334666, 17.78000000000000114, 31.75000000000000000 ) ) ;
#53819=CYLINDRICAL_SURFACE ( 'NONE', #82647, 7.937500000000000000 ) ;
#53827=VECTOR ( 'NONE', #30417, 1000.000000000000000 ) ;
#53851=CARTESIAN_POINT ( 'NONE',  ( -12.69999999999999929, 82.54999999999999716, 129.9368274816650057 ) ) ;
#53858=ADVANCED_FACE ( 'NONE', ( #35258 ), #8472, .T. ) ;
#53868=AXIS2_PLACEMENT_3D ( 'NONE', #5303, #19823, #20719 ) ;
#53888=CARTESIAN_POINT ( 'NONE',  ( -126.7857788319987407, 47.45011355129853570, 31.15124566716904653 ) ) ;
#53895=AXIS2_PLACEMENT_3D ( 'NONE', #1300, #84434, #2198 ) ;
#53925=CARTESIAN_POINT ( 'NONE',  ( 125.3463460965256786, 53.27927791669488755, -36.51250000000000284 ) ) ;
#53926=EDGE_LOOP ( 'NONE', ( #8813, #40635, #51627, #679 ) ) ;
#53967=PLANE ( 'NONE',  #20451 ) ;
#54012=ORIENTED_EDGE ( 'NONE', *, *, #31173, .F. ) ;
#54030=AXIS2_PLACEMENT_3D ( 'NONE', #51047, #66005, #36977 ) ;
#54035=CARTESIAN_POINT ( 'NONE',  ( -194.1576000000000022, 20.32000000000000028, -213.9117947927954901 ) ) ;
#54040=VECTOR ( 'NONE', #47827, 1000.000000000000000 ) ;
#54048=CIRCLE ( 'NONE', #1842, 8.636000000000004562 ) ;
#54095=LINE ( 'NONE', #40495, #43838 ) ;
#54166=VERTEX_POINT ( 'NONE', #11128 ) ;
#54171=ORIENTED_EDGE ( 'NONE', *, *, #20971, .F. ) ;
#54197=CARTESIAN_POINT ( 'NONE',  ( 0.000000000000000000, 0.000000000000000000, 0.000000000000000000 ) ) ;
#54221=CYLINDRICAL_SURFACE ( 'NONE', #28290, 9.425000000000000711 ) ;
#54222=VERTEX_POINT ( 'NONE', #66991 ) ;
#54247=ORIENTED_EDGE ( 'NONE', *, *, #45957, .F. ) ;
#54262=AXIS2_PLACEMENT_3D ( 'NONE', #46607, #75686, #26187 ) ;
#54273=CARTESIAN_POINT ( 'NONE',  ( -109.3008916335299716, 55.38362039756903954, 71.40162167859008946 ) ) ;
#54276=ADVANCED_FACE ( 'NONE', ( #47426 ), #12939, .T. ) ;
#54295=CIRCLE ( 'NONE', #6417, 8.636000000000004562 ) ;
#54297=CARTESIAN_POINT ( 'NONE',  ( 0.000000000000000000, 0.000000000000000000, -161.5439999999999827 ) ) ;
#54325=EDGE_LOOP ( 'NONE', ( #81229, #65471, #16520, #52795 ) ) ;
#54335=CARTESIAN_POINT ( 'NONE',  ( -126.9767693855287405, 51.08807848479448666, 30.36069443887403096 ) ) ;
#54354=EDGE_LOOP ( 'NONE', ( #56791, #19171, #32278, #77683 ) ) ;
#54365=CARTESIAN_POINT ( 'NONE',  ( 0.000000000000000000, 1.270000000000000018, 0.000000000000000000 ) ) ;
#54431=SHAPE_DEFINITION_REPRESENTATION ( #46997, #48599 ) ;
#54456=AXIS2_PLACEMENT_3D ( 'NONE', #37049, #64755, #59699 ) ;
#54464=ORIENTED_EDGE ( 'NONE', *, *, #70161, .F. ) ;
#54472=EDGE_CURVE ( 'NONE', #59655, #66001, #65100, .T. ) ;
#54479=ORIENTED_EDGE ( 'NONE', *, *, #53809, .F. ) ;
#54484=DIRECTION ( 'NONE',  ( 0.000000000000000000, 0.000000000000000000, -1.000000000000000000 ) ) ;
#54519=VECTOR ( 'NONE', #12388, 1000.000000000000000 ) ;
#54555=VERTEX_POINT ( 'NONE', #57833 ) ;
#54557=CARTESIAN_POINT ( 'NONE',  ( -33.98325472291465132, 24.56180297284579694, -3.174999999999764899 ) ) ;
#54574=VECTOR ( 'NONE', #47895, 1000.000000000000000 ) ;
#54618=ORIENTED_EDGE ( 'NONE', *, *, #63536, .F. ) ;
#54626=CYLINDRICAL_SURFACE ( 'NONE', #50677, 6.349999999999994316 ) ;
#54665=EDGE_CURVE ( 'NONE', #43971, #21656, #83179, .T. ) ;
#54668=ORIENTED_EDGE ( 'NONE', *, *, #53155, .T. ) ;
#54684=AXIS2_PLACEMENT_3D ( 'NONE', #35348, #76249, #63063 ) ;
#54687=FACE_OUTER_BOUND ( 'NONE', #52563, .T. ) ;
#54706=CIRCLE ( 'NONE', #86655, 12.69999999999998863 ) ;
#54716=ORIENTED_EDGE ( 'NONE', *, *, #365, .T. ) ;
#54717=CARTESIAN_POINT ( 'NONE',  ( 131.3179999999999836, 37.33800000000000097, 58.73749999999999716 ) ) ;
#54725=CARTESIAN_POINT ( 'NONE',  ( -125.5854312618940867, 68.04355014475468977, 35.68462287192087956 ) ) ;
#54726=ORIENTED_EDGE ( 'NONE', *, *, #20174, .F. ) ;
#54749=CARTESIAN_POINT ( 'NONE',  ( -8.063121854991559090, 72.73576936706652418, 130.3067131650634565 ) ) ;
#54786=CARTESIAN_POINT ( 'NONE',  ( -127.0239848601435995, 53.97500000000000142, 30.16249999999999787 ) ) ;
#54819=DIRECTION ( 'NONE',  ( 0.000000000000000000, -1.000000000000000000, 0.000000000000000000 ) ) ;
#54848=EDGE_CURVE ( 'NONE', #82011, #36180, #51236, .T. ) ;
#54884=ADVANCED_FACE ( 'NONE', ( #7348 ), #27782, .F. ) ;
#54886=ADVANCED_FACE ( 'NONE', ( #523 ), #12088, .T. ) ;
#54891=VECTOR ( 'NONE', #63393, 1000.000000000000000 ) ;
#54904=DIRECTION ( 'NONE',  ( 0.000000000000000000, 3.785359618865284342E-16, 1.000000000000000000 ) ) ;
#54919=AXIS2_PLACEMENT_3D ( 'NONE', #43470, #69860, #58011 ) ;
#54930=DIRECTION ( 'NONE',  ( 0.000000000000000000, -1.000000000000000000, 0.000000000000000000 ) ) ;
#54933=CARTESIAN_POINT ( 'NONE',  ( 7.736379116599698236, 72.47620246569817937, 130.3265317108386512 ) ) ;
#54940=CARTESIAN_POINT ( 'NONE',  ( 119.7018510303924756, 50.62094380000917937, -52.11861110539391717 ) ) ;
#54947=DIRECTION ( 'NONE',  ( 0.000000000000000000, 1.000000000000000000, 0.000000000000000000 ) ) ;
#54956=VERTEX_POINT ( 'NONE', #77741 ) ;
#55017=CARTESIAN_POINT ( 'NONE',  ( 1.166476076187854022E-15, 95.00619999999999266, 9.525000000000000355 ) ) ;
#55023=VECTOR ( 'NONE', #27486, 1000.000000000000000 ) ;
#55094=CYLINDRICAL_SURFACE ( 'NONE', #88917, 218.1859999999999786 ) ;
#55108=AXIS2_PLACEMENT_3D ( 'NONE', #52184, #19485, #47168 ) ;
#55111=CARTESIAN_POINT ( 'NONE',  ( -110.7653435595065901, 44.45000000000000284, 69.10794311903988785 ) ) ;
#55115=ORIENTED_EDGE ( 'NONE', *, *, #13693, .T. ) ;
#55127=CARTESIAN_POINT ( 'NONE',  ( -44.45000000000000284, 101.5999999999999943, 206.3750000000000000 ) ) ;
#55143=ORIENTED_EDGE ( 'NONE', *, *, #31574, .F. ) ;
#55166=CARTESIAN_POINT ( 'NONE',  ( -119.0649508995676626, 74.44429733102370506, 53.56549206838347743 ) ) ;
#55193=ORIENTED_EDGE ( 'NONE', *, *, #34695, .T. ) ;
#55198=CARTESIAN_POINT ( 'NONE',  ( -5.566352093571659942, 71.12725780905140027, 130.4377547077455688 ) ) ;
#55241=EDGE_CURVE ( 'NONE', #12149, #23464, #33931, .T. ) ;
#55258=LINE ( 'NONE', #76174, #39071 ) ;
#55269=ORIENTED_EDGE ( 'NONE', *, *, #55917, .F. ) ;
#55272=ORIENTED_EDGE ( 'NONE', *, *, #20945, .F. ) ;
#55275=VECTOR ( 'NONE', #36532, 1000.000000000000114 ) ;
#55299=ORIENTED_EDGE ( 'NONE', *, *, #53298, .T. ) ;
#55303=ORIENTED_EDGE ( 'NONE', *, *, #68926, .T. ) ;
#55313=LINE ( 'NONE', #60801, #66656 ) ;
#55349=DIRECTION ( 'NONE',  ( 1.000000000000000000, 0.000000000000000000, -1.224646799147355919E-16 ) ) ;
#55364=VERTEX_POINT ( 'NONE', #50695 ) ;
#55366=LINE ( 'NONE', #89476, #23493 ) ;
#55369=FACE_OUTER_BOUND ( 'NONE', #64821, .T. ) ;
#55386=CARTESIAN_POINT ( 'NONE',  ( 4.049920669541869245, 70.48119388710848909, 130.4956849816146871 ) ) ;
#55390=VECTOR ( 'NONE', #86070, 1000.000000000000000 ) ;
#55403=DIRECTION ( 'NONE',  ( 0.000000000000000000, -1.000000000000000000, 0.000000000000000000 ) ) ;
#55407=VECTOR ( 'NONE', #39750, 1000.000000000000000 ) ;
#55410=LINE ( 'NONE', #83165, #73247 ) ;
#55421=LINE ( 'NONE', #29092, #33239 ) ;
#55425=CIRCLE ( 'NONE', #40915, 179.8898777604655095 ) ;
#55433=VERTEX_POINT ( 'NONE', #30269 ) ;
#55447=DIRECTION ( 'NONE',  ( 1.000000000000000000, 0.000000000000000000, -6.982966722218760189E-15 ) ) ;
#55460=ORIENTED_EDGE ( 'NONE', *, *, #46365, .T. ) ;
#55462=DIRECTION ( 'NONE',  ( 1.000000000000000000, 0.000000000000000000, 1.472650733923983947E-14 ) ) ;
#55530=ORIENTED_EDGE ( 'NONE', *, *, #65769, .T. ) ;
#55532=DIRECTION ( 'NONE',  ( 0.000000000000000000, 0.000000000000000000, -1.000000000000000000 ) ) ;
#55535=FACE_OUTER_BOUND ( 'NONE', #12840, .T. ) ;
#55539=DIRECTION ( 'NONE',  ( 0.000000000000000000, -1.000000000000000000, 0.000000000000000000 ) ) ;
#55575=ORIENTED_EDGE ( 'NONE', *, *, #69162, .F. ) ;
#55583=DIRECTION ( 'NONE',  ( -1.000000000000000000, 0.000000000000000000, 0.000000000000000000 ) ) ;
#55587=CARTESIAN_POINT ( 'NONE',  ( 3.063943826786764771E-15, 1.270000000000000018, -24.63800000000000168 ) ) ;
#55601=VECTOR ( 'NONE', #84064, 1000.000000000000000 ) ;
#55612=ORIENTED_EDGE ( 'NONE', *, *, #69602, .F. ) ;
#55614=CARTESIAN_POINT ( 'NONE',  ( -125.8688597900877397, 66.85668029895285258, 34.66965736785963514 ) ) ;
#55638=AXIS2_PLACEMENT_3D ( 'NONE', #30181, #24259, #86052 ) ;
#55641=CARTESIAN_POINT ( 'NONE',  ( -10.81204423530230585, 75.87175144098965518, 130.1077780123643208 ) ) ;
#55693=ADVANCED_FACE ( 'NONE', ( #13014 ), #61147, .F. ) ;
#55695=CARTESIAN_POINT ( 'NONE',  ( -12.69999999999999929, 83.33535579944408767, 129.9368274816650057 ) ) ;
#55740=LINE ( 'NONE', #62138, #36095 ) ;
#55762=ORIENTED_EDGE ( 'NONE', *, *, #10019, .F. ) ;
#55813=VECTOR ( 'NONE', #35523, 1000.000000000000000 ) ;
#55832=CARTESIAN_POINT ( 'NONE',  ( 9.432210905596992490, 74.04481405089026680, 130.2149380284310212 ) ) ;
#55885=( NAMED_UNIT ( * ) SI_UNIT ( $, .STERADIAN. ) SOLID_ANGLE_UNIT ( ) );
#55912=CARTESIAN_POINT ( 'NONE',  ( 0.000000000000000000, 17.78000000000000114, 0.000000000000000000 ) ) ;
#55917=EDGE_CURVE ( 'NONE', #57180, #19136, #67316, .T. ) ;
#55968=EDGE_LOOP ( 'NONE', ( #32352, #54171 ) ) ;
#55989=CARTESIAN_POINT ( 'NONE',  ( 10.57409824832103418, 75.51590200896762894, 130.1270826008356778 ) ) ;
#56015=DIRECTION ( 'NONE',  ( 0.000000000000000000, -1.000000000000000000, 0.000000000000000000 ) ) ;
#56022=EDGE_CURVE ( 'NONE', #28034, #34082, #73151, .T. ) ;
#56072=CARTESIAN_POINT ( 'NONE',  ( -124.4872849904342189, 71.15633340822272146, 39.34666567088954992 ) ) ;
#56100=PLANE ( 'NONE',  #39190 ) ;
#56122=CARTESIAN_POINT ( 'NONE',  ( -215.9000000000000057, 101.5999999999999943, -45.33899999999999864 ) ) ;
#56145=AXIS2_PLACEMENT_3D ( 'NONE', #24917, #88499, #82141 ) ;
#56156=CARTESIAN_POINT ( 'NONE',  ( -11.73779877120047743, 87.39914602784801900, 130.0272786502210067 ) ) ;
#56170=ORIENTED_EDGE ( 'NONE', *, *, #37826, .T. ) ;
#56194=PLANE ( 'NONE',  #1772 ) ;
#56204=CARTESIAN_POINT ( 'NONE',  ( 19.18896583590734650, 64.29237593614118396, 32.91936650831844702 ) ) ;
#56217=CIRCLE ( 'NONE', #15670, 6.349999999999994316 ) ;
#56219=LINE ( 'NONE', #83970, #7110 ) ;
#56227=AXIS2_PLACEMENT_3D ( 'NONE', #87738, #74553, #60462 ) ;
#56238=CARTESIAN_POINT ( 'NONE',  ( -71.09939861440099662, 101.5999999999999943, 177.8662485265279827 ) ) ;
#56281=CARTESIAN_POINT ( 'NONE',  ( -3.174999999999664979, 17.78000000000000114, 31.75000000000000000 ) ) ;
#56295=CARTESIAN_POINT ( 'NONE',  ( 119.6084552581333469, 51.66411822165594003, -52.33259208581855404 ) ) ;
#56299=ORIENTED_EDGE ( 'NONE', *, *, #29743, .T. ) ;
#56376=DIRECTION ( 'NONE',  ( 0.000000000000000000, 1.000000000000000000, 0.000000000000000000 ) ) ;
#56379=CARTESIAN_POINT ( 'NONE',  ( 173.9900000000000091, 21.46300000000000097, 41.63456447661474868 ) ) ;
#56454=EDGE_CURVE ( 'NONE', #17490, #2213, #24627, .T. ) ;
#56510=ADVANCED_FACE ( 'NONE', ( #4634 ), #73669, .T. ) ;
#56514=CYLINDRICAL_SURFACE ( 'NONE', #87400, 20.63750000000000284 ) ;
#56533=CARTESIAN_POINT ( 'NONE',  ( -119.5597780469935145, 74.55132283206019395, 52.44562168052537743 ) ) ;
#56575=LINE ( 'NONE', #43386, #7977 ) ;
#56595=ORIENTED_EDGE ( 'NONE', *, *, #59929, .F. ) ;
#56606=VERTEX_POINT ( 'NONE', #53643 ) ;
#56615=CARTESIAN_POINT ( 'NONE',  ( 135.2444258376730204, 20.32000000000000028, -147.4575741623271767 ) ) ;
#56633=EDGE_LOOP ( 'NONE', ( #56987, #40441, #493, #73925 ) ) ;
#56651=EDGE_CURVE ( 'NONE', #48373, #47090, #59573, .T. ) ;
#56667=CARTESIAN_POINT ( 'NONE',  ( 19.63602930441068750, 63.82048847602042940, 32.65376468583215086 ) ) ;
#56719=VECTOR ( 'NONE', #17084, 1000.000000000000114 ) ;
#56724=ORIENTED_EDGE ( 'NONE', *, *, #15951, .T. ) ;
#56733=CIRCLE ( 'NONE', #19069, 9.425000000000000711 ) ;
#56756=CARTESIAN_POINT ( 'NONE',  ( 119.7724476469521449, 50.10406306454358827, -51.95653040766548258 ) ) ;
#56769=CARTESIAN_POINT ( 'NONE',  ( -179.8898777604655095, 101.5999999999999943, 114.2999999999999972 ) ) ;
#56791=ORIENTED_EDGE ( 'NONE', *, *, #75206, .F. ) ;
#56793=DIRECTION ( 'NONE',  ( 0.000000000000000000, -1.000000000000000000, 0.000000000000000000 ) ) ;
#56798=PRESENTATION_STYLE_ASSIGNMENT (( #43166 ) ) ;
#56802=DIRECTION ( 'NONE',  ( 0.000000000000000000, 0.000000000000000000, -1.000000000000000000 ) ) ;
#56809=DIRECTION ( 'NONE',  ( 0.000000000000000000, -1.000000000000000000, 0.000000000000000000 ) ) ;
#56810=CARTESIAN_POINT ( 'NONE',  ( 0.000000000000000000, 20.32000000000000028, 0.000000000000000000 ) ) ;
#56823=CARTESIAN_POINT ( 'NONE',  ( -33.98325472291465132, 17.78000000000000114, -3.174999999999764899 ) ) ;
#56845=ADVANCED_FACE ( 'NONE', ( #45721, #73450 ), #38479, .F. ) ;
#56863=CIRCLE ( 'NONE', #62708, 9.525000000000000355 ) ;
#56877=ORIENTED_EDGE ( 'NONE', *, *, #75353, .T. ) ;
#56905=CARTESIAN_POINT ( 'NONE',  ( 11.92955753101793626, 78.19254692348476965, 130.0098836371429627 ) ) ;
#56910=DIRECTION ( 'NONE',  ( 0.000000000000000000, 0.000000000000000000, -1.000000000000000000 ) ) ;
#56917=ORIENTED_EDGE ( 'NONE', *, *, #72694, .T. ) ;
#56938=DIRECTION ( 'NONE',  ( 0.000000000000000000, -1.000000000000000000, 0.000000000000000000 ) ) ;
#56942=ORIENTED_EDGE ( 'NONE', *, *, #32889, .F. ) ;
#56957=VERTEX_POINT ( 'NONE', #69337 ) ;
#56987=ORIENTED_EDGE ( 'NONE', *, *, #62520, .F. ) ;
#57010=DIRECTION ( 'NONE',  ( 0.7071067811865330288, 0.000000000000000000, 0.7071067811865621167 ) ) ;
#57017=DIRECTION ( 'NONE',  ( 0.000000000000000000, -1.000000000000000000, 0.000000000000000000 ) ) ;
#57028=CARTESIAN_POINT ( 'NONE',  ( -194.1576000000000022, 0.000000000000000000, 114.2999999999999972 ) ) ;
#57047=EDGE_LOOP ( 'NONE', ( #80767, #47949 ) ) ;
#57062=EDGE_CURVE ( 'NONE', #43158, #16965, #41378, .T. ) ;
#57070=EDGE_CURVE ( 'NONE', #43122, #17548, #2541, .T. ) ;
#57082=DIRECTION ( 'NONE',  ( 0.000000000000000000, 1.000000000000000000, 0.000000000000000000 ) ) ;
#57125=VERTEX_POINT ( 'NONE', #22538 ) ;
#57131=CARTESIAN_POINT ( 'NONE',  ( 0.000000000000000000, 152.3879256507328250, 0.000000000000000000 ) ) ;
#57148=FACE_OUTER_BOUND ( 'NONE', #5154, .T. ) ;
#57167=VERTEX_POINT ( 'NONE', #35699 ) ;
#57173=CIRCLE ( 'NONE', #68804, 34.13125000000000142 ) ;
#57175=ADVANCED_FACE ( 'NONE', ( #71586 ), #9346, .T. ) ;
#57180=VERTEX_POINT ( 'NONE', #66528 ) ;
#57186=CARTESIAN_POINT ( 'NONE',  ( -23.27731929905162289, 53.97500000000000142, 30.16249999999999076 ) ) ;
#57188=FACE_OUTER_BOUND ( 'NONE', #60902, .T. ) ;
#57221=EDGE_CURVE ( 'NONE', #6370, #18422, #31112, .T. ) ;
#57235=DIRECTION ( 'NONE',  ( 7.980413499659429724E-32, 1.000000000000000000, -3.785359618865284342E-16 ) ) ;
#57254=CYLINDRICAL_SURFACE ( 'NONE', #17515, 8.636000000000004562 ) ;
#57267=VECTOR ( 'NONE', #79613, 1000.000000000000000 ) ;
#57272=PLANE ( 'NONE',  #2310 ) ;
#57278=VERTEX_POINT ( 'NONE', #86553 ) ;
#57287=ORIENTED_EDGE ( 'NONE', *, *, #32327, .T. ) ;
#57318=VECTOR ( 'NONE', #70939, 1000.000000000000000 ) ;
#57321=AXIS2_PLACEMENT_3D ( 'NONE', #61080, #88365, #82895 ) ;
#57333=AXIS2_PLACEMENT_3D ( 'NONE', #16730, #78078, #29919 ) ;
#57348=CARTESIAN_POINT ( 'NONE',  ( 10.86079732252673580, 75.96631587555827991, 130.1035022676263679 ) ) ;
#57356=DIRECTION ( 'NONE',  ( 0.000000000000000000, 1.000000000000000000, 0.000000000000000000 ) ) ;
#57362=ADVANCED_FACE ( 'NONE', ( #46960 ), #67877, .T. ) ;
#57386=FACE_OUTER_BOUND ( 'NONE', #65042, .T. ) ;
#57389=ORIENTED_EDGE ( 'NONE', *, *, #21042, .F. ) ;
#57409=ADVANCED_FACE ( 'NONE', ( #88341 ), #77724, .F. ) ;
#57463=DIRECTION ( 'NONE',  ( 0.000000000000000000, 0.000000000000000000, 1.000000000000000000 ) ) ;
#57464=CARTESIAN_POINT ( 'NONE',  ( 173.9900000000000091, 37.33800000000000097, 32.46912895322940074 ) ) ;
#57471=DIRECTION ( 'NONE',  ( 0.000000000000000000, 0.000000000000000000, 1.000000000000000000 ) ) ;
#57478=ORIENTED_EDGE ( 'NONE', *, *, #75444, .F. ) ;
#57487=DIRECTION ( 'NONE',  ( 0.000000000000000000, -1.000000000000000000, 0.000000000000000000 ) ) ;
#57494=VECTOR ( 'NONE', #81544, 1000.000000000000114 ) ;
#57516=CARTESIAN_POINT ( 'NONE',  ( -8.224930598656271741, 92.23576600848676321, 130.2969003264876449 ) ) ;
#57522=AXIS2_PLACEMENT_3D ( 'NONE', #39875, #18097, #88054 ) ;
#57537=DIRECTION ( 'NONE',  ( 1.000000000000000000, 0.000000000000000000, 0.000000000000000000 ) ) ;
#57554=LINE ( 'NONE', #22612, #14805 ) ;
#57559=VERTEX_POINT ( 'NONE', #78743 ) ;
#57560=CIRCLE ( 'NONE', #15508, 8.636000000000004562 ) ;
#57567=LINE ( 'NONE', #22625, #4950 ) ;
#57570=DIRECTION ( 'NONE',  ( 0.000000000000000000, 1.000000000000000000, 0.000000000000000000 ) ) ;
#57574=VERTEX_POINT ( 'NONE', #11003 ) ;
#57653=CARTESIAN_POINT ( 'NONE',  ( 125.2667151975434479, 50.60771645571414723, -36.78494105014318194 ) ) ;
#57684=FACE_OUTER_BOUND ( 'NONE', #69849, .T. ) ;
#57686=CARTESIAN_POINT ( 'NONE',  ( 125.4480236541915019, 68.52740834580446005, 36.16247866844641123 ) ) ;
#57688=EDGE_LOOP ( 'NONE', ( #59624, #72425 ) ) ;
#57718=ORIENTED_EDGE ( 'NONE', *, *, #29878, .T. ) ;
#57811=CIRCLE ( 'NONE', #2714, 38.10000000000000142 ) ;
#57821=CARTESIAN_POINT ( 'NONE',  ( -160.2664750769284865, 20.32000000000000028, 148.0533267522753818 ) ) ;
#57833=CARTESIAN_POINT ( 'NONE',  ( 71.09939861440099662, 0.000000000000000000, 177.8662485265279827 ) ) ;
#57866=CARTESIAN_POINT ( 'NONE',  ( 127.0239848601435995, 53.97500000000000142, 30.16249999999999787 ) ) ;
#57869=DIRECTION ( 'NONE',  ( 1.000000000000000000, 0.000000000000000000, 0.000000000000000000 ) ) ;
#57873=ORIENTED_EDGE ( 'NONE', *, *, #7221, .T. ) ;
#57887=CARTESIAN_POINT ( 'NONE',  ( -126.9019698816670711, 58.54574603448291725, 30.67188900999152423 ) ) ;
#57925=ORIENTED_EDGE ( 'NONE', *, *, #78560, .F. ) ;
#57990=EDGE_CURVE ( 'NONE', #12239, #89203, #49997, .T. ) ;
#57992=ORIENTED_EDGE ( 'NONE', *, *, #26526, .F. ) ;
#58011=DIRECTION ( 'NONE',  ( 0.000000000000000000, 0.000000000000000000, 1.000000000000000000 ) ) ;
#58041=B_SPLINE_CURVE_WITH_KNOTS ( 'NONE', 3,
 ( #57186, #29503, #64469, #73055, #64028, #84933, #78118, #15881, #43559, #9067, #47464, #20679 ),
 .UNSPECIFIED., .F., .F.,
 ( 4, 2, 2, 2, 2, 4 ),
 ( 0.08510440135476479706, 0.08774507987650315144, 0.09038575839824151970, 0.09302643691997988795, 0.09434677618084906514, 0.09566711544171824233 ),
 .UNSPECIFIED. ) ;
#58045=FACE_OUTER_BOUND ( 'NONE', #29531, .T. ) ;
#58067=AXIS2_PLACEMENT_3D ( 'NONE', #42448, #47914, #34300 ) ;
#58083=DIRECTION ( 'NONE',  ( 0.000000000000000000, 0.000000000000000000, 1.000000000000000000 ) ) ;
#58105=CARTESIAN_POINT ( 'NONE',  ( 125.3300043389053684, 51.65368650150782770, -36.56872758047426686 ) ) ;
#58123=ORIENTED_EDGE ( 'NONE', *, *, #35021, .F. ) ;
#58143=EDGE_CURVE ( 'NONE', #23113, #25704, #79524, .T. ) ;
#58170=CARTESIAN_POINT ( 'NONE',  ( -3.175000000000120171, 8.255000000000000782, -33.98325472291460159 ) ) ;
#58184=VERTEX_POINT ( 'NONE', #59486 ) ;
#58197=CARTESIAN_POINT ( 'NONE',  ( 0.000000000000000000, 20.32000000000000028, 0.000000000000000000 ) ) ;
#58214=CARTESIAN_POINT ( 'NONE',  ( -75.61066417432020614, 20.32000000000000028, 177.0380000000000109 ) ) ;
#58226=ORIENTED_EDGE ( 'NONE', *, *, #64289, .T. ) ;
#58230=VERTEX_POINT ( 'NONE', #81320 ) ;
#58231=DIRECTION ( 'NONE',  ( 0.000000000000000000, 0.000000000000000000, 1.000000000000000000 ) ) ;
#58232=ORIENTED_EDGE ( 'NONE', *, *, #43016, .T. ) ;
#58249=ORIENTED_EDGE ( 'NONE', *, *, #12476, .T. ) ;
#58331=CARTESIAN_POINT ( 'NONE',  ( -126.6753767262755446, 61.56490666960836222, 31.59592044441793135 ) ) ;
#58334=VECTOR ( 'NONE', #28722, 1000.000000000000000 ) ;
#58341=CARTESIAN_POINT ( 'NONE',  ( -33.98325472291465132, 8.255000000000000782, -3.174999999999764899 ) ) ;
#58394=ORIENTED_EDGE ( 'NONE', *, *, #50901, .F. ) ;
#58407=EDGE_CURVE ( 'NONE', #45672, #19975, #82659, .T. ) ;
#58411=CARTESIAN_POINT ( 'NONE',  ( 126.8302186627767725, 48.26449426118261243, 30.96720769570602627 ) ) ;
#58432=VERTEX_POINT ( 'NONE', #48087 ) ;
#58447=EDGE_LOOP ( 'NONE', ( #57718, #37273 ) ) ;
#58468=ORIENTED_EDGE ( 'NONE', *, *, #52645, .F. ) ;
#58557=LINE ( 'NONE', #59447, #49848 ) ;
#58564=CARTESIAN_POINT ( 'NONE',  ( 110.5173296318792069, 62.69970716989340076, 69.50396515567824451 ) ) ;
#58566=ORIENTED_EDGE ( 'NONE', *, *, #53557, .T. ) ;
#58581=EDGE_CURVE ( 'NONE', #43342, #19136, #78077, .T. ) ;
#58598=B_SPLINE_CURVE_WITH_KNOTS ( 'NONE', 3,
 ( #54786, #13484, #40281, #54335, #68452, #34360, #60717, #53888, #47081, #82991 ),
 .UNSPECIFIED., .F., .F.,
 ( 4, 2, 2, 2, 4 ),
 ( 0.000000000000000000, 0.2500000000000008327, 0.3750000000000011102, 0.5000000000000014433, 1.000000000000000000 ),
 .UNSPECIFIED. ) ;
#58601=ADVANCED_FACE ( 'NONE', ( #81655 ), #60722, .T. ) ;
#58607=CARTESIAN_POINT ( 'NONE',  ( 110.7653435595065901, 44.45000000000000284, 69.10794311903988785 ) ) ;
#58646=LINE ( 'NONE', #1925, #43679 ) ;
#58681=DIRECTION ( 'NONE',  ( -0.000000000000000000, 0.000000000000000000, 1.000000000000000000 ) ) ;
#58692=DIRECTION ( 'NONE',  ( 0.000000000000000000, 0.000000000000000000, 1.000000000000000000 ) ) ;
#58707=CARTESIAN_POINT ( 'NONE',  ( 4.506942778454146037, 94.42426803962317194, 130.4782289187788251 ) ) ;
#58713=DIRECTION ( 'NONE',  ( 0.000000000000000000, 0.000000000000000000, 1.000000000000000000 ) ) ;
#58744=VECTOR ( 'NONE', #87272, 1000.000000000000000 ) ;
#58752=CARTESIAN_POINT ( 'NONE',  ( 135.2444258376725941, 101.5999999999999943, 147.4575741623265799 ) ) ;
#58783=CARTESIAN_POINT ( 'NONE',  ( 1.166476076187854022E-15, 2.269999999999994245, 9.525000000000000355 ) ) ;
#58843=CARTESIAN_POINT ( 'NONE',  ( -7.370840183531916168, 92.89254840543441105, 130.3477230843911059 ) ) ;
#58846=EDGE_LOOP ( 'NONE', ( #75904, #4034, #31617, #15683 ) ) ;
#58859=ORIENTED_EDGE ( 'NONE', *, *, #83344, .F. ) ;
#58916=CARTESIAN_POINT ( 'NONE',  ( 3.174999999999889688, 8.255000000000000782, -31.75000000000000000 ) ) ;
#58950=FACE_OUTER_BOUND ( 'NONE', #50822, .T. ) ;
#58959=CARTESIAN_POINT ( 'NONE',  ( 121.4418839049407097, 59.87844259738950825, -47.92489995295673566 ) ) ;
#58989=DIRECTION ( 'NONE',  ( 0.000000000000000000, 1.000000000000000000, 0.000000000000000000 ) ) ;
#58992=DIRECTION ( 'NONE',  ( 0.000000000000000000, 0.000000000000000000, 1.000000000000000000 ) ) ;
#59004=CARTESIAN_POINT ( 'NONE',  ( 109.5833183008944474, 58.35583844470681214, 70.96735860772342619 ) ) ;
#59009=FACE_OUTER_BOUND ( 'NONE', #17846, .T. ) ;
#59013=EDGE_CURVE ( 'NONE', #32410, #74769, #83470, .T. ) ;
#59061=EDGE_CURVE ( 'NONE', #23464, #71527, #47194, .T. ) ;
#59086=EDGE_CURVE ( 'NONE', #88388, #121, #45760, .T. ) ;
#59088=EDGE_CURVE ( 'NONE', #65725, #45672, #28341, .T. ) ;
#59099=ORIENTED_EDGE ( 'NONE', *, *, #14538, .T. ) ;
#59185=CARTESIAN_POINT ( 'NONE',  ( 0.000000000000000000, 114.2999999999999972, 0.000000000000000000 ) ) ;
#59190=AXIS2_PLACEMENT_3D ( 'NONE', #48758, #56015, #87553 ) ;
#59217=CARTESIAN_POINT ( 'NONE',  ( 0.000000000000000000, 1.270000000000000018, 0.000000000000000000 ) ) ;
#59232=CIRCLE ( 'NONE', #82485, 38.10000000000000142 ) ;
#59237=ORIENTED_EDGE ( 'NONE', *, *, #29177, .T. ) ;
#59240=CARTESIAN_POINT ( 'NONE',  ( -14.47561641184040226, 67.58393596072598086, 35.26458586194669920 ) ) ;
#59247=DIRECTION ( 'NONE',  ( 0.000000000000000000, 0.000000000000000000, -1.000000000000000000 ) ) ;
#59248=DIRECTION ( 'NONE',  ( 0.000000000000000000, 0.000000000000000000, -1.000000000000000000 ) ) ;
#59292=CARTESIAN_POINT ( 'NONE',  ( -9.373716445341450765, 91.13655357722605288, 130.2196449801177209 ) ) ;
#59293=CARTESIAN_POINT ( 'NONE',  ( -33.98325472291465132, 8.255000000000000782, -3.174999999999764899 ) ) ;
#59302=ADVANCED_FACE ( 'NONE', ( #70936, #28224 ), #57272, .F. ) ;
#59320=AXIS2_PLACEMENT_3D ( 'NONE', #72948, #43561, #32058 ) ;
#59334=FACE_OUTER_BOUND ( 'NONE', #49468, .T. ) ;
#59347=PLANE ( 'NONE',  #70720 ) ;
#59363=CARTESIAN_POINT ( 'NONE',  ( -75.61066417432020614, 0.000000000000000000, 177.0380000000000109 ) ) ;
#59379=VECTOR ( 'NONE', #13473, 1000.000000000000000 ) ;
#59389=DIRECTION ( 'NONE',  ( 0.000000000000000000, 0.000000000000000000, 1.000000000000000000 ) ) ;
#59391=LINE ( 'NONE', #87120, #78068 ) ;
#59397=VERTEX_POINT ( 'NONE', #58607 ) ;
#59411=CARTESIAN_POINT ( 'NONE',  ( 119.9073604651600249, 56.10210383135144241, -51.64404161576485564 ) ) ;
#59431=ORIENTED_EDGE ( 'NONE', *, *, #25426, .T. ) ;
#59447=CARTESIAN_POINT ( 'NONE',  ( -71.09939861440099662, 20.32000000000000028, 177.8662485265279827 ) ) ;
#59455=CARTESIAN_POINT ( 'NONE',  ( 120.1783960690039095, 74.61161073219626871, 51.01009929557958600 ) ) ;
#59479=ORIENTED_EDGE ( 'NONE', *, *, #75078, .T. ) ;
#59486=CARTESIAN_POINT ( 'NONE',  ( 75.61066417432020614, 20.32000000000000028, 177.0380000000000109 ) ) ;
#59504=ORIENTED_EDGE ( 'NONE', *, *, #53155, .F. ) ;
#59533=VECTOR ( 'NONE', #14783, 1000.000000000000000 ) ;
#59538=ADVANCED_FACE ( 'NONE', ( #18628 ), #6339, .F. ) ;
#59542=CARTESIAN_POINT ( 'NONE',  ( 208.9149999999999920, 43.68799999999999528, 44.45000000000000284 ) ) ;
#59546=ORIENTED_EDGE ( 'NONE', *, *, #70408, .F. ) ;
#59550=ORIENTED_EDGE ( 'NONE', *, *, #73899, .F. ) ;
#59568=FACE_OUTER_BOUND ( 'NONE', #31729, .T. ) ;
#59573=LINE ( 'NONE', #87309, #77646 ) ;
#59612=VECTOR ( 'NONE', #55403, 1000.000000000000000 ) ;
#59624=ORIENTED_EDGE ( 'NONE', *, *, #74411, .T. ) ;
#59652=CARTESIAN_POINT ( 'NONE',  ( 57.91199999999999903, 101.5999999999999943, 191.3008000794699797 ) ) ;
#59655=VERTEX_POINT ( 'NONE', #28567 ) ;
#59681=CARTESIAN_POINT ( 'NONE',  ( -186.2398777604655038, 20.32000000000000028, -12.69999999999999929 ) ) ;
#59699=DIRECTION ( 'NONE',  ( 0.000000000000000000, 0.000000000000000000, -1.000000000000000000 ) ) ;
#59710=ORIENTED_EDGE ( 'NONE', *, *, #39871, .F. ) ;
#59717=EDGE_CURVE ( 'NONE', #84162, #52633, #18248, .T. ) ;
#59722=ORIENTED_EDGE ( 'NONE', *, *, #32955, .F. ) ;
#59747=ORIENTED_EDGE ( 'NONE', *, *, #20701, .T. ) ;
#59748=DIRECTION ( 'NONE',  ( 0.000000000000000000, -1.000000000000000000, 0.000000000000000000 ) ) ;
#59777=EDGE_LOOP ( 'NONE', ( #40690, #2508 ) ) ;
#59780=DIRECTION ( 'NONE',  ( 0.000000000000000000, -1.000000000000000000, 0.000000000000000000 ) ) ;
#59787=FACE_OUTER_BOUND ( 'NONE', #76888, .T. ) ;
#59793=CARTESIAN_POINT ( 'NONE',  ( 147.4575741623265799, 0.000000000000000000, 135.2444258376725941 ) ) ;
#59811=AXIS2_PLACEMENT_3D ( 'NONE', #74299, #59748, #72520 ) ;
#59816=EDGE_CURVE ( 'NONE', #32634, #79978, #41363, .T. ) ;
#59836=ADVANCED_FACE ( 'NONE', ( #20052 ), #48175, .F. ) ;
#59852=CARTESIAN_POINT ( 'NONE',  ( 125.2636845449844287, 54.85408740538772321, -36.79518296114878240 ) ) ;
#59898=CARTESIAN_POINT ( 'NONE',  ( 120.0727942879283745, 74.60757107455795278, 51.25817907159669318 ) ) ;
#59913=DIRECTION ( 'NONE',  ( 0.000000000000000000, 1.000000000000000000, 0.000000000000000000 ) ) ;
#59929=EDGE_CURVE ( 'NONE', #25704, #67615, #49524, .T. ) ;
#59946=ORIENTED_EDGE ( 'NONE', *, *, #5381, .T. ) ;
#59977=ORIENTED_EDGE ( 'NONE', *, *, #20318, .T. ) ;
#60012=VERTEX_POINT ( 'NONE', #67078 ) ;
#60025=EDGE_CURVE ( 'NONE', #77712, #46235, #73441, .T. ) ;
#60037=VECTOR ( 'NONE', #84857, 1000.000000000000000 ) ;
#60043=CARTESIAN_POINT ( 'NONE',  ( 12.30956025940465537, 85.78406842316067582, 129.9748705538268325 ) ) ;
#60076=AXIS2_PLACEMENT_3D ( 'NONE', #25870, #45836, #39041 ) ;
#60160=CARTESIAN_POINT ( 'NONE',  ( 208.9149999999999920, 37.33800000000000097, 50.79999999999999716 ) ) ;
#60184=DIRECTION ( 'NONE',  ( -1.000000000000000000, 0.000000000000000000, -2.108231265501709878E-16 ) ) ;
#60185=CARTESIAN_POINT ( 'NONE',  ( 131.3179999999999836, 44.45000000000000284, 69.10794311903988785 ) ) ;
#60216=PLANE ( 'NONE',  #17529 ) ;
#60220=ORIENTED_EDGE ( 'NONE', *, *, #6824, .F. ) ;
#60234=CARTESIAN_POINT ( 'NONE',  ( -4.352199961275779572, 70.61852695876001462, 130.4834258897450923 ) ) ;
#60250=CIRCLE ( 'NONE', #38469, 6.349999999999994316 ) ;
#60296=AXIS2_PLACEMENT_3D ( 'NONE', #20433, #14056, #83556 ) ;
#60303=CARTESIAN_POINT ( 'NONE',  ( 124.8813761161696476, 57.47090627086830494, -38.07277077706557833 ) ) ;
#60315=VERTEX_POINT ( 'NONE', #8906 ) ;
#60316=PLANE ( 'NONE',  #57522 ) ;
#60331=CARTESIAN_POINT ( 'NONE',  ( 0.000000000000000000, 101.5999999999999943, 0.000000000000000000 ) ) ;
#60348=CARTESIAN_POINT ( 'NONE',  ( 118.0314967278394533, 74.00740537028835320, 55.80249333958784774 ) ) ;
#60395=CARTESIAN_POINT ( 'NONE',  ( -185.9961463128564958, 20.32000000000000028, -9.525000000000000355 ) ) ;
#60404=LINE ( 'NONE', #5009, #34247 ) ;
#60409=DIRECTION ( 'NONE',  ( 0.000000000000000000, 0.000000000000000000, 1.000000000000000000 ) ) ;
#60429=EDGE_LOOP ( 'NONE', ( #70303, #10546, #55303, #80352 ) ) ;
#60450=ORIENTED_EDGE ( 'NONE', *, *, #18090, .T. ) ;
#60459=ORIENTED_EDGE ( 'NONE', *, *, #991, .T. ) ;
#60462=DIRECTION ( 'NONE',  ( 0.000000000000000000, 0.000000000000000000, -1.000000000000000000 ) ) ;
#60494=CARTESIAN_POINT ( 'NONE',  ( 11.66424111575752320, 87.57388405225547956, 130.0339036534010120 ) ) ;
#60495=ORIENTED_EDGE ( 'NONE', *, *, #22276, .F. ) ;
#60514=CYLINDRICAL_SURFACE ( 'NONE', #21638, 7.937500000000000000 ) ;
#60526=CARTESIAN_POINT ( 'NONE',  ( 131.3179999999999836, 37.33800000000000097, 50.79999999999999716 ) ) ;
#60527=CARTESIAN_POINT ( 'NONE',  ( -55.48342271751670296, 20.32000000000000028, 171.1197181046785261 ) ) ;
#60608=CARTESIAN_POINT ( 'NONE',  ( 22.09100578693153594, 47.99823937963132892, 31.04264637510191349 ) ) ;
#60628=CARTESIAN_POINT ( 'NONE',  ( 0.000000000000000000, 2.269999999999994245, 0.000000000000000000 ) ) ;
#60645=AXIS2_PLACEMENT_3D ( 'NONE', #74089, #66821, #72753 ) ;
#60648=VERTEX_POINT ( 'NONE', #26089 ) ;
#60656=CARTESIAN_POINT ( 'NONE',  ( -110.2860940435973873, 61.86465508475756536, 69.87023241873045265 ) ) ;
#60684=CARTESIAN_POINT ( 'NONE',  ( -11.72824152711724288, 77.67777890152783016, 130.0281412439851465 ) ) ;
#60704=DIRECTION ( 'NONE',  ( 0.000000000000000000, -1.000000000000000000, 0.000000000000000000 ) ) ;
#60713=ORIENTED_EDGE ( 'NONE', *, *, #85042, .T. ) ;
#60717=CARTESIAN_POINT ( 'NONE',  ( -126.9052826151614823, 49.45974035476580610, 30.65825619889020004 ) ) ;
#60722=CYLINDRICAL_SURFACE ( 'NONE', #61659, 179.8898777604655095 ) ;
#60724=VERTEX_POINT ( 'NONE', #20618 ) ;
#60752=DIRECTION ( 'NONE',  ( 0.000000000000000000, 1.000000000000000000, 0.000000000000000000 ) ) ;
#60757=CARTESIAN_POINT ( 'NONE',  ( 123.4412257795802645, 60.45185376280554834, -42.51366219649503364 ) ) ;
#60771=FACE_OUTER_BOUND ( 'NONE', #14570, .T. ) ;
#60801=CARTESIAN_POINT ( 'NONE',  ( -3.174999999999644995, 8.255000000000000782, 33.98325472291465132 ) ) ;
#60803=DIRECTION ( 'NONE',  ( -1.000000000000000000, 0.000000000000000000, -8.503806984168940141E-16 ) ) ;
#60819=CIRCLE ( 'NONE', #4286, 9.524999999999998579 ) ;
#60880=CARTESIAN_POINT ( 'NONE',  ( 9.073998176338214705, 73.66341487109981756, 130.2403208068726030 ) ) ;
#60902=EDGE_LOOP ( 'NONE', ( #29572, #34731, #73024, #36047 ) ) ;
#60904=CIRCLE ( 'NONE', #30452, 6.349999999999994316 ) ;
#60919=CARTESIAN_POINT ( 'NONE',  ( 0.000000000000000000, 1.270000000000000018, 0.000000000000000000 ) ) ;
#60923=CYLINDRICAL_SURFACE ( 'NONE', #56227, 6.349999999999997868 ) ;
#60928=AXIS2_PLACEMENT_3D ( 'NONE', #27696, #20887, #13619 ) ;
#60956=AXIS2_PLACEMENT_3D ( 'NONE', #60331, #39893, #32633 ) ;
#60963=DIRECTION ( 'NONE',  ( 0.000000000000000000, 0.000000000000000000, 1.000000000000000000 ) ) ;
#60981=LINE ( 'NONE', #53688, #54519 ) ;
#60990=DIRECTION ( 'NONE',  ( 1.000000000000000000, 0.000000000000000000, 0.000000000000000000 ) ) ;
#60997=LINE ( 'NONE', #88726, #76728 ) ;
#61011=EDGE_LOOP ( 'NONE', ( #54479, #77284, #51280, #38787 ) ) ;
#61025=EDGE_CURVE ( 'NONE', #13532, #18491, #1051, .T. ) ;
#61042=AXIS2_PLACEMENT_3D ( 'NONE', #1196, #36621, #64321 ) ;
#61058=VECTOR ( 'NONE', #54947, 1000.000000000000000 ) ;
#61079=ORIENTED_EDGE ( 'NONE', *, *, #71034, .T. ) ;
#61080=CARTESIAN_POINT ( 'NONE',  ( -187.8075999999999794, 0.000000000000000000, -12.69999999999999929 ) ) ;
#61087=DIRECTION ( 'NONE',  ( 0.000000000000000000, 0.000000000000000000, 1.000000000000000000 ) ) ;
#61131=ORIENTED_EDGE ( 'NONE', *, *, #44415, .T. ) ;
#61147=CYLINDRICAL_SURFACE ( 'NONE', #54262, 7.874000000000005883 ) ;
#61152=VECTOR ( 'NONE', #68640, 1000.000000000000000 ) ;
#61172=EDGE_CURVE ( 'NONE', #16001, #65247, #54706, .T. ) ;
#61229=EDGE_LOOP ( 'NONE', ( #23503, #82771, #31226, #87492 ) ) ;
#61233=DIRECTION ( 'NONE',  ( 0.000000000000000000, 1.000000000000000000, 0.000000000000000000 ) ) ;
#61247=DIRECTION ( 'NONE',  ( 0.000000000000000000, 0.000000000000000000, -1.000000000000000000 ) ) ;
#61252=DIRECTION ( 'NONE',  ( 6.982966722218760189E-15, 0.000000000000000000, 1.000000000000000000 ) ) ;
#61254=ORIENTED_EDGE ( 'NONE', *, *, #32946, .F. ) ;
#61274=VERTEX_POINT ( 'NONE', #49084 ) ;
#61281=CARTESIAN_POINT ( 'NONE',  ( -148.0533267522752112, 0.000000000000000000, 160.2664750769289697 ) ) ;
#61296=DIRECTION ( 'NONE',  ( 0.000000000000000000, 1.000000000000000000, 0.000000000000000000 ) ) ;
#61313=ORIENTED_EDGE ( 'NONE', *, *, #38700, .T. ) ;
#61317=DIRECTION ( 'NONE',  ( 0.000000000000000000, -1.000000000000000000, 0.000000000000000000 ) ) ;
#61322=CARTESIAN_POINT ( 'NONE',  ( 9.818283287276351246, 74.49179306748567342, 130.1865249340722812 ) ) ;
#61331=VECTOR ( 'NONE', #37034, 1000.000000000000000 ) ;
#61343=ORIENTED_EDGE ( 'NONE', *, *, #15771, .F. ) ;
#61396=CARTESIAN_POINT ( 'NONE',  ( 10.80657803997667443, 89.23705086585235335, 130.1082320863853568 ) ) ;
#61414=VECTOR ( 'NONE', #17284, 1000.000000000000000 ) ;
#61429=CIRCLE ( 'NONE', #55638, 130.5560000000000116 ) ;
#61435=CARTESIAN_POINT ( 'NONE',  ( 170.2205283966864897, 20.32000000000000028, -71.37400000000000944 ) ) ;
#61437=DIRECTION ( 'NONE',  ( 0.000000000000000000, 1.000000000000000000, 0.000000000000000000 ) ) ;
#61441=ORIENTED_EDGE ( 'NONE', *, *, #3798, .T. ) ;
#61446=ORIENTED_EDGE ( 'NONE', *, *, #80736, .F. ) ;
#61457=EDGE_CURVE ( 'NONE', #19136, #57180, #2617, .T. ) ;
#61469=VECTOR ( 'NONE', #15984, 1000.000000000000000 ) ;
#61497=CARTESIAN_POINT ( 'NONE',  ( 0.000000000000000000, 8.255000000000000782, 0.000000000000000000 ) ) ;
#61504=ORIENTED_EDGE ( 'NONE', *, *, #75766, .F. ) ;
#61505=CARTESIAN_POINT ( 'NONE',  ( -31.75000000000000000, 17.78000000000000114, -3.174999999999779998 ) ) ;
#61515=ORIENTED_EDGE ( 'NONE', *, *, #52340, .T. ) ;
#61524=CARTESIAN_POINT ( 'NONE',  ( 31.75000000000000000, 17.78000000000000114, -3.174999999999999822 ) ) ;
#61550=DIRECTION ( 'NONE',  ( 0.000000000000000000, -1.000000000000000000, 0.000000000000000000 ) ) ;
#61553=CARTESIAN_POINT ( 'NONE',  ( -122.6777674792067643, 73.68547069920268200, 44.66800687705570994 ) ) ;
#61572=ADVANCED_FACE ( 'NONE', ( #21300 ), #62628, .F. ) ;
#61579=CARTESIAN_POINT ( 'NONE',  ( -4.848965775826784785, 70.81212673990701489, 130.4659219253704237 ) ) ;
#61586=CARTESIAN_POINT ( 'NONE',  ( 0.000000000000000000, 2.031999999999865025, 25.39999999999999858 ) ) ;
#61601=CARTESIAN_POINT ( 'NONE',  ( 3.174999999999889688, 24.56180297284579694, -31.75000000000000000 ) ) ;
#61606=AXIS2_PLACEMENT_3D ( 'NONE', #25027, #3256, #16435 ) ;
#61608=AXIS2_PLACEMENT_3D ( 'NONE', #80755, #31692, #59389 ) ;
#61628=CARTESIAN_POINT ( 'NONE',  ( -186.2398777604659870, 101.5999999999999943, 107.9500000000000028 ) ) ;
#61634=LINE ( 'NONE', #42093, #34248 ) ;
#61642=CYLINDRICAL_SURFACE ( 'NONE', #1214, 130.5560000000000116 ) ;
#61659=AXIS2_PLACEMENT_3D ( 'NONE', #40289, #53442, #52984 ) ;
#61677=LINE ( 'NONE', #19463, #80098 ) ;
#61679=CARTESIAN_POINT ( 'NONE',  ( -194.1576000000000022, 20.32000000000000028, -9.525000000000000355 ) ) ;
#61687=DIRECTION ( 'NONE',  ( -0.000000000000000000, 1.000000000000000000, 0.000000000000000000 ) ) ;
#61693=CARTESIAN_POINT ( 'NONE',  ( 3.174999999999889688, 17.78000000000000114, -31.75000000000000000 ) ) ;
#61695=VERTEX_POINT ( 'NONE', #34918 ) ;
#61749=ORIENTED_EDGE ( 'NONE', *, *, #58407, .F. ) ;
#61750=CARTESIAN_POINT ( 'NONE',  ( 3.175000000000334666, 8.255000000000000782, 31.75000000000000000 ) ) ;
#61774=CARTESIAN_POINT ( 'NONE',  ( 163.0822201311030142, 20.32000000000000028, 75.92468371870748456 ) ) ;
#61786=EDGE_LOOP ( 'NONE', ( #412, #45953, #12099, #63704 ) ) ;
#61793=ORIENTED_EDGE ( 'NONE', *, *, #6030, .T. ) ;
#61811=EDGE_CURVE ( 'NONE', #21770, #84402, #38843, .T. ) ;
#61845=VECTOR ( 'NONE', #68939, 1000.000000000000000 ) ;
#61875=CIRCLE ( 'NONE', #50265, 6.349999999999999645 ) ;
#61895=DIRECTION ( 'NONE',  ( -1.047445008332813989E-14, 0.000000000000000000, -1.000000000000000000 ) ) ;
#61901=ORIENTED_EDGE ( 'NONE', *, *, #64375, .T. ) ;
#61903=DIRECTION ( 'NONE',  ( -1.000000000000000000, 0.000000000000000000, 1.107319919754840046E-14 ) ) ;
#61910=EDGE_CURVE ( 'NONE', #73841, #54555, #67546, .T. ) ;
#61944=CIRCLE ( 'NONE', #73558, 130.5560000000000116 ) ;
#61993=EDGE_CURVE ( 'NONE', #34396, #64746, #11355, .T. ) ;
#62001=DIRECTION ( 'NONE',  ( -1.000000000000000000, 0.000000000000000000, 0.000000000000000000 ) ) ;
#62009=CARTESIAN_POINT ( 'NONE',  ( -124.9130890353168581, 70.14308647312734024, 37.96932838610722882 ) ) ;
#62035=CARTESIAN_POINT ( 'NONE',  ( -10.34205959026443367, 75.17848243421535415, 130.1458012250857337 ) ) ;
#62064=AXIS2_PLACEMENT_3D ( 'NONE', #51666, #3534, #43962 ) ;
#62068=VECTOR ( 'NONE', #28021, 1000.000000000000000 ) ;
#62072=CARTESIAN_POINT ( 'NONE',  ( 75.61066417432020614, 20.32000000000000028, 189.7379999999999995 ) ) ;
#62077=CARTESIAN_POINT ( 'NONE',  ( -33.98325472291460159, 8.255000000000000782, 3.175000000000234746 ) ) ;
#62082=ORIENTED_EDGE ( 'NONE', *, *, #85632, .F. ) ;
#62132=FACE_OUTER_BOUND ( 'NONE', #8962, .T. ) ;
#62138=CARTESIAN_POINT ( 'NONE',  ( 160.2664750769289697, 20.32000000000000028, 148.0533267522752112 ) ) ;
#62152=DIRECTION ( 'NONE',  ( 0.000000000000000000, -1.000000000000000000, 0.000000000000000000 ) ) ;
#62179=DIRECTION ( 'NONE',  ( 0.000000000000000000, -1.000000000000000000, 0.000000000000000000 ) ) ;
#62182=VECTOR ( 'NONE', #42729, 1000.000000000000000 ) ;
#62205=DIRECTION ( 'NONE',  ( 0.000000000000000000, -1.000000000000000000, 0.000000000000000000 ) ) ;
#62223=CARTESIAN_POINT ( 'NONE',  ( 9.347434767860939075, 73.95160161085279071, 130.2210325332607113 ) ) ;
#62231=CARTESIAN_POINT ( 'NONE',  ( 123.6107665481496554, 45.16440871034607341, -42.01786438290864822 ) ) ;
#62237=LINE ( 'NONE', #20916, #61058 ) ;
#62238=DIRECTION ( 'NONE',  ( 0.000000000000000000, 0.000000000000000000, -1.000000000000000000 ) ) ;
#62267=CIRCLE ( 'NONE', #39052, 154.1697486074984909 ) ;
#62270=CARTESIAN_POINT ( 'NONE',  ( -179.6205029264235122, 20.32000000000000028, 123.8612349545196025 ) ) ;
#62279=ORIENTED_EDGE ( 'NONE', *, *, #44415, .F. ) ;
#62280=VECTOR ( 'NONE', #10868, 1000.000000000000000 ) ;
#62281=DIRECTION ( 'NONE',  ( 0.000000000000000000, 0.000000000000000000, 1.000000000000000000 ) ) ;
#62312=DIRECTION ( 'NONE',  ( -0.3552177606235690788, 0.000000000000000000, -0.9347835805883503157 ) ) ;
#62321=DIRECTION ( 'NONE',  ( 0.000000000000000000, -1.000000000000000000, 0.000000000000000000 ) ) ;
#62348=ORIENTED_EDGE ( 'NONE', *, *, #44125, .F. ) ;
#62400=EDGE_CURVE ( 'NONE', #23269, #31479, #83930, .T. ) ;
#62441=CARTESIAN_POINT ( 'NONE',  ( 0.000000000000000000, 44.45000000000000284, 130.5560000000000116 ) ) ;
#62450=ORIENTED_EDGE ( 'NONE', *, *, #3636, .F. ) ;
#62460=CARTESIAN_POINT ( 'NONE',  ( -124.6636586881827355, 70.76753038983027011, 38.78354852543069597 ) ) ;
#62482=LINE ( 'NONE', #262, #33030 ) ;
#62486=CARTESIAN_POINT ( 'NONE',  ( -5.206817487757472662, 70.96034413118437101, 130.4525921376586552 ) ) ;
#62520=EDGE_CURVE ( 'NONE', #57574, #24397, #21425, .T. ) ;
#62548=CARTESIAN_POINT ( 'NONE',  ( -160.2664750769284865, 101.5999999999999943, 148.0533267522753818 ) ) ;
#62586=DIRECTION ( 'NONE',  ( 0.000000000000000000, 1.000000000000000000, 0.000000000000000000 ) ) ;
#62590=DIRECTION ( 'NONE',  ( 1.840813417405305102E-14, 0.000000000000000000, -1.000000000000000000 ) ) ;
#62623=EDGE_CURVE ( 'NONE', #6147, #83969, #42285, .T. ) ;
#62624=ORIENTED_EDGE ( 'NONE', *, *, #40552, .T. ) ;
#62628=PLANE ( 'NONE',  #53340 ) ;
#62683=CARTESIAN_POINT ( 'NONE',  ( 120.4566699508395402, 47.42106607564514320, -50.34970303805386749 ) ) ;
#62708=AXIS2_PLACEMENT_3D ( 'NONE', #21631, #21174, #77037 ) ;
#62710=VERTEX_POINT ( 'NONE', #58170 ) ;
#62748=CARTESIAN_POINT ( 'NONE',  ( -158.9822249764580135, 101.5999999999999943, 107.9500000000000028 ) ) ;
#62751=VECTOR ( 'NONE', #46446, 1000.000000000000000 ) ;
#62767=DIRECTION ( 'NONE',  ( 0.7071067811865116015, 0.000000000000000000, -0.7071067811865835440 ) ) ;
#62771=ORIENTED_EDGE ( 'NONE', *, *, #53809, .T. ) ;
#62799=EDGE_CURVE ( 'NONE', #54222, #42800, #6334, .T. ) ;
#62810=DIRECTION ( 'NONE',  ( -0.000000000000000000, 1.000000000000000000, 0.000000000000000000 ) ) ;
#62818=DIRECTION ( 'NONE',  ( 0.000000000000000000, -1.000000000000000000, 0.000000000000000000 ) ) ;
#62859=FACE_OUTER_BOUND ( 'NONE', #9202, .T. ) ;
#62902=CARTESIAN_POINT ( 'NONE',  ( -124.1113515626113326, 71.86650245416660709, 40.51253187952720225 ) ) ;
#62936=LINE ( 'NONE', #42482, #38073 ) ;
#62938=DIRECTION ( 'NONE',  ( 0.000000000000000000, -1.000000000000000000, 0.000000000000000000 ) ) ;
#62968=DIRECTION ( 'NONE',  ( 0.000000000000000000, 0.000000000000000000, 1.000000000000000000 ) ) ;
#63006=EDGE_CURVE ( 'NONE', #64746, #12239, #43075, .T. ) ;
#63039=VECTOR ( 'NONE', #80164, 1000.000000000000000 ) ;
#63041=CARTESIAN_POINT ( 'NONE',  ( -215.9010000000000105, 52.73749999999999716, -52.38749999999999574 ) ) ;
#63063=DIRECTION ( 'NONE',  ( 0.000000000000000000, -1.000000000000000000, 0.000000000000000000 ) ) ;
#63097=PLANE ( 'NONE',  #18291 ) ;
#63102=ADVANCED_FACE ( 'NONE', ( #22673 ), #43527, .T. ) ;
#63113=VERTEX_POINT ( 'NONE', #66660 ) ;
#63138=DIRECTION ( 'NONE',  ( 0.000000000000000000, 0.000000000000000000, 1.000000000000000000 ) ) ;
#63158=CARTESIAN_POINT ( 'NONE',  ( 125.6515680309144329, 67.77259609856692180, 35.44867019240336958 ) ) ;
#63173=ORIENTED_EDGE ( 'NONE', *, *, #25426, .F. ) ;
#63182=VERTEX_POINT ( 'NONE', #85797 ) ;
#63217=LINE ( 'NONE', #42749, #14471 ) ;
#63265=DIRECTION ( 'NONE',  ( 0.7071067811865370256, 0.000000000000000000, -0.7071067811865580088 ) ) ;
#63282=FACE_BOUND ( 'NONE', #4151, .T. ) ;
#63288=DIRECTION ( 'NONE',  ( 1.047445008332813989E-14, 0.000000000000000000, 1.000000000000000000 ) ) ;
#63320=AXIS2_PLACEMENT_3D ( 'NONE', #4719, #10626, #17888 ) ;
#63323=ORIENTED_EDGE ( 'NONE', *, *, #3756, .F. ) ;
#63337=ORIENTED_EDGE ( 'NONE', *, *, #61172, .T. ) ;
#63361=CARTESIAN_POINT ( 'NONE',  ( -120.7378339438464678, 74.60054165536443804, 49.68010905324412363 ) ) ;
#63393=DIRECTION ( 'NONE',  ( 0.000000000000000000, 0.8660254037844387076, -0.4999999999999998890 ) ) ;
#63486=DIRECTION ( 'NONE',  ( 0.000000000000000000, 1.000000000000000000, 0.000000000000000000 ) ) ;
#63488=FACE_OUTER_BOUND ( 'NONE', #70592, .T. ) ;
#63490=CARTESIAN_POINT ( 'NONE',  ( 23.27731929905161934, 54.66493626280016827, 30.16249999999999076 ) ) ;
#63498=ORIENTED_EDGE ( 'NONE', *, *, #2468, .T. ) ;
#63524=CARTESIAN_POINT ( 'NONE',  ( -3.174999999999664979, 24.56180297284579694, 31.75000000000000000 ) ) ;
#63536=EDGE_CURVE ( 'NONE', #57574, #69150, #60819, .T. ) ;
#63586=CARTESIAN_POINT ( 'NONE',  ( 120.6819903923023389, 46.87498547512231539, -49.80728659620316989 ) ) ;
#63594=CARTESIAN_POINT ( 'NONE',  ( 3.174999999999879918, 24.56180297284579694, -33.98325472291465132 ) ) ;
#63612=CARTESIAN_POINT ( 'NONE',  ( 125.3763439628640128, 68.77237897621238005, 36.41030492311487166 ) ) ;
#63619=PLANE ( 'NONE',  #9958 ) ;
#63628=SHAPE_REPRESENTATION_RELATIONSHIP ( 'NONE' , 'NONE' ,  #48599, #83525 ) ;
#63643=ADVANCED_FACE ( 'NONE', ( #14686 ), #77808, .T. ) ;
#63644=CARTESIAN_POINT ( 'NONE',  ( 141.3509999999999991, 101.5999999999999943, -141.3509999999999991 ) ) ;
#63704=ORIENTED_EDGE ( 'NONE', *, *, #45957, .T. ) ;
#63708=ORIENTED_EDGE ( 'NONE', *, *, #13993, .F. ) ;
#63724=DIRECTION ( 'NONE',  ( 1.000000000000000000, 0.000000000000000000, 0.000000000000000000 ) ) ;
#63744=CARTESIAN_POINT ( 'NONE',  ( -3.174999999999644995, 17.78000000000000114, 33.98325472291465132 ) ) ;
#63758=AXIS2_PLACEMENT_3D ( 'NONE', #76450, #62810, #63724 ) ;
#63786=DIRECTION ( 'NONE',  ( 0.000000000000000000, 1.000000000000000000, 0.000000000000000000 ) ) ;
#63824=EDGE_CURVE ( 'NONE', #49608, #23986, #55313, .T. ) ;
#63827=ORIENTED_EDGE ( 'NONE', *, *, #84373, .T. ) ;
#63834=ORIENTED_EDGE ( 'NONE', *, *, #31026, .T. ) ;
#63871=VECTOR ( 'NONE', #88151, 1000.000000000000000 ) ;
#63926=EDGE_CURVE ( 'NONE', #63182, #53038, #14485, .T. ) ;
#63949=CARTESIAN_POINT ( 'NONE',  ( 13.26698260364423199, 68.06966155350374947, 35.72126630662602054 ) ) ;
#63953=DIRECTION ( 'NONE',  ( 0.000000000000000000, 0.000000000000000000, 1.000000000000000000 ) ) ;
#63956=EDGE_CURVE ( 'NONE', #8973, #43788, #73926, .T. ) ;
#64003=AXIS2_PLACEMENT_3D ( 'NONE', #41522, #21107, #34724 ) ;
#64028=CARTESIAN_POINT ( 'NONE',  ( -22.68723905695524934, 49.61528013047381336, 30.61088831204059701 ) ) ;
#64029=CARTESIAN_POINT ( 'NONE',  ( 108.8673596973266058, 37.33800000000000097, 50.79999999999999716 ) ) ;
#64054=EDGE_CURVE ( 'NONE', #23269, #31466, #11671, .T. ) ;
#64144=CARTESIAN_POINT ( 'NONE',  ( 1.971923734479900239E-14, 11.98343896644750117, 160.4955849403809793 ) ) ;
#64158=VERTEX_POINT ( 'NONE', #27083 ) ;
#64175=ORIENTED_EDGE ( 'NONE', *, *, #22398, .F. ) ;
#64181=LINE ( 'NONE', #2850, #72683 ) ;
#64186=CARTESIAN_POINT ( 'NONE',  ( 11.76728917727518464, 77.77273929673829400, 130.0246156895997274 ) ) ;
#64188=CARTESIAN_POINT ( 'NONE',  ( 131.3179999999999836, 37.33800000000000097, 42.86249999999999716 ) ) ;
#64216=DIRECTION ( 'NONE',  ( 0.000000000000000000, -1.000000000000000000, 0.000000000000000000 ) ) ;
#64218=CARTESIAN_POINT ( 'NONE',  ( 196.2150000000000034, 43.68799999999999528, 44.45000000000000284 ) ) ;
#64263=ADVANCED_FACE ( 'NONE', ( #4849 ), #53407, .F. ) ;
#64268=VERTEX_POINT ( 'NONE', #20279 ) ;
#64289=EDGE_CURVE ( 'NONE', #15997, #17885, #49067, .T. ) ;
#64311=DIRECTION ( 'NONE',  ( -1.000000000000000000, 0.000000000000000000, -2.108231265501709878E-16 ) ) ;
#64315=LINE ( 'NONE', #85663, #32935 ) ;
#64321=DIRECTION ( 'NONE',  ( 0.000000000000000000, 0.000000000000000000, -1.000000000000000000 ) ) ;
#64322=ORIENTED_EDGE ( 'NONE', *, *, #69248, .F. ) ;
#64336=VERTEX_POINT ( 'NONE', #50648 ) ;
#64355=EDGE_CURVE ( 'NONE', #56606, #18423, #43379, .T. ) ;
#64365=ORIENTED_EDGE ( 'NONE', *, *, #65376, .T. ) ;
#64368=FACE_OUTER_BOUND ( 'NONE', #83571, .T. ) ;
#64375=EDGE_CURVE ( 'NONE', #54166, #61695, #269, .T. ) ;
#64387=ORIENTED_EDGE ( 'NONE', *, *, #54472, .T. ) ;
#64395=CARTESIAN_POINT ( 'NONE',  ( 22.90570976208508824, 57.39977848847996000, 30.44578217438603218 ) ) ;
#64400=CARTESIAN_POINT ( 'NONE',  ( 170.2205283966864897, 101.5999999999999943, -79.24800000000000466 ) ) ;
#64405=DIRECTION ( 'NONE',  ( 0.000000000000000000, 1.000000000000000000, 0.000000000000000000 ) ) ;
#64407=ORIENTED_EDGE ( 'NONE', *, *, #10019, .T. ) ;
#64408=DIRECTION ( 'NONE',  ( 0.000000000000000000, 0.000000000000000000, 1.000000000000000000 ) ) ;
#64417=CARTESIAN_POINT ( 'NONE',  ( -187.8075999999999794, 101.5999999999999943, -3.174999999999999822 ) ) ;
#64420=VECTOR ( 'NONE', #22160, 1000.000000000000000 ) ;
#64427=DIRECTION ( 'NONE',  ( 0.000000000000000000, -1.000000000000000000, 0.000000000000000000 ) ) ;
#64440=CARTESIAN_POINT ( 'NONE',  ( 0.000000000000000000, 101.5999999999999943, 0.000000000000000000 ) ) ;
#64469=CARTESIAN_POINT ( 'NONE',  ( -23.20326867387899128, 52.20473367193696390, 30.22006327746032284 ) ) ;
#64579=DIRECTION ( 'NONE',  ( 1.000000000000000000, 0.000000000000000000, -6.982966722218760189E-15 ) ) ;
#64623=LINE ( 'NONE', #31429, #50638 ) ;
#64627=LINE ( 'NONE', #3743, #87417 ) ;
#64650=DIRECTION ( 'NONE',  ( 0.000000000000000000, 0.000000000000000000, 1.000000000000000000 ) ) ;
#64668=AXIS2_PLACEMENT_3D ( 'NONE', #14630, #62312, #35495 ) ;
#64675=DIRECTION ( 'NONE',  ( 0.000000000000000000, -1.000000000000000000, 0.000000000000000000 ) ) ;
#64710=CARTESIAN_POINT ( 'NONE',  ( -126.7366439761708818, 60.90736961166211216, 31.34868955532726886 ) ) ;
#64723=DIRECTION ( 'NONE',  ( 0.000000000000000000, -1.000000000000000000, 0.000000000000000000 ) ) ;
#64725=VERTEX_POINT ( 'NONE', #64188 ) ;
#64746=VERTEX_POINT ( 'NONE', #28769 ) ;
#64754=CARTESIAN_POINT ( 'NONE',  ( -135.2444258376730204, 0.000000000000000000, 147.4575741623271767 ) ) ;
#64755=DIRECTION ( 'NONE',  ( 0.000000000000000000, -1.000000000000000000, 0.000000000000000000 ) ) ;
#64793=CIRCLE ( 'NONE', #9670, 7.937500000000000000 ) ;
#64804=ORIENTED_EDGE ( 'NONE', *, *, #23192, .T. ) ;
#64821=EDGE_LOOP ( 'NONE', ( #86504, #9572, #28105, #61901 ) ) ;
#64840=CARTESIAN_POINT ( 'NONE',  ( 7.511964023296719084, 69.63594209550339542, 37.35831287037660076 ) ) ;
#64847=DIRECTION ( 'NONE',  ( -1.749395751137010036E-15, 0.000000000000000000, -1.000000000000000000 ) ) ;
#64860=LINE ( 'NONE', #37158, #76655 ) ;
#64861=CARTESIAN_POINT ( 'NONE',  ( -141.3509999999999991, 0.000000000000000000, -141.3509999999999991 ) ) ;
#64870=EDGE_CURVE ( 'NONE', #74824, #54956, #86426, .T. ) ;
#64872=EDGE_CURVE ( 'NONE', #56957, #6370, #64623, .T. ) ;
#64884=VERTEX_POINT ( 'NONE', #65073 ) ;
#64897=ORIENTED_EDGE ( 'NONE', *, *, #78560, .T. ) ;
#64938=CIRCLE ( 'NONE', #18498, 6.349999999999999645 ) ;
#64955=CARTESIAN_POINT ( 'NONE',  ( 126.9549993752607264, 57.49093265451766399, 30.45191747052217934 ) ) ;
#64961=CARTESIAN_POINT ( 'NONE',  ( 0.000000000000000000, 17.78000000000000114, 0.000000000000000000 ) ) ;
#65005=ORIENTED_EDGE ( 'NONE', *, *, #39658, .T. ) ;
#65013=DIRECTION ( 'NONE',  ( 0.000000000000000000, -1.000000000000000000, 0.000000000000000000 ) ) ;
#65031=DIRECTION ( 'NONE',  ( 1.000000000000000000, -0.000000000000000000, 2.108231265501709878E-16 ) ) ;
#65042=EDGE_LOOP ( 'NONE', ( #10850, #36360 ) ) ;
#65073=CARTESIAN_POINT ( 'NONE',  ( -215.9000000000000057, 53.97500000000000142, 30.16249999999999787 ) ) ;
#65078=CONICAL_SURFACE ( 'NONE', #54919, 25.39999999999999858, 0.7853981633974984611 ) ;
#65100=LINE ( 'NONE', #64218, #419 ) ;
#65129=DIRECTION ( 'NONE',  ( 0.000000000000000000, 0.000000000000000000, -1.000000000000000000 ) ) ;
#65132=LINE ( 'NONE', #2916, #85789 ) ;
#65141=DIRECTION ( 'NONE',  ( 0.000000000000000000, 1.000000000000000000, 0.000000000000000000 ) ) ;
#65150=ORIENTED_EDGE ( 'NONE', *, *, #59086, .F. ) ;
#65161=CARTESIAN_POINT ( 'NONE',  ( 135.2444258376730204, 101.5999999999999943, -147.4575741623271767 ) ) ;
#65167=EDGE_CURVE ( 'NONE', #37741, #75634, #22305, .T. ) ;
#65180=CARTESIAN_POINT ( 'NONE',  ( 0.000000000000000000, 2.031999999999865025, 0.000000000000000000 ) ) ;
#65188=( GEOMETRIC_REPRESENTATION_CONTEXT ( 3 ) GLOBAL_UNCERTAINTY_ASSIGNED_CONTEXT ( ( #35109 ) ) GLOBAL_UNIT_ASSIGNED_CONTEXT ( ( #20515, #76361, #55885 ) ) REPRESENTATION_CONTEXT ( 'NONE', 'WORKASPACE' ) );
#65193=ORIENTED_EDGE ( 'NONE', *, *, #50273, .F. ) ;
#65207=ORIENTED_EDGE ( 'NONE', *, *, #70625, .T. ) ;
#65217=EDGE_CURVE ( 'NONE', #81504, #10881, #76811, .T. ) ;
#65222=EDGE_LOOP ( 'NONE', ( #74311, #71867, #21, #67751 ) ) ;
#65234=CARTESIAN_POINT ( 'NONE',  ( -10.55958528308446986, 89.60586021078158581, 130.1282609435105826 ) ) ;
#65239=DIRECTION ( 'NONE',  ( 0.000000000000000000, 1.000000000000000000, 0.000000000000000000 ) ) ;
#65242=AXIS2_PLACEMENT_3D ( 'NONE', #2178, #1732, #29433 ) ;
#65247=VERTEX_POINT ( 'NONE', #89551 ) ;
#65252=MECHANICAL_DESIGN_GEOMETRIC_PRESENTATION_REPRESENTATION('',(#11570),#65188);
#65309=DIRECTION ( 'NONE',  ( 0.000000000000000000, 0.000000000000000000, 1.000000000000000000 ) ) ;
#65310=CARTESIAN_POINT ( 'NONE',  ( 0.000000000000000000, 0.000000000000000000, 0.000000000000000000 ) ) ;
#65312=VERTEX_POINT ( 'NONE', #30012 ) ;
#65320=CARTESIAN_POINT ( 'NONE',  ( -75.61066417432020614, 20.32000000000000028, 177.0380000000000109 ) ) ;
#65326=LINE ( 'NONE', #3102, #24033 ) ;
#65376=EDGE_CURVE ( 'NONE', #43971, #72757, #23223, .T. ) ;
#65401=CARTESIAN_POINT ( 'NONE',  ( 111.7869510898867276, 66.18006229446802990, 67.44307826104233072 ) ) ;
#65422=DIRECTION ( 'NONE',  ( 0.000000000000000000, -1.000000000000000000, 0.000000000000000000 ) ) ;
#65430=CARTESIAN_POINT ( 'NONE',  ( -31.75000000000000000, 24.56180297284579694, 3.175000000000219647 ) ) ;
#65449=VERTEX_POINT ( 'NONE', #74358 ) ;
#65471=ORIENTED_EDGE ( 'NONE', *, *, #69624, .F. ) ;
#65474=PLANE ( 'NONE',  #71520 ) ;
#65476=ADVANCED_FACE ( 'NONE', ( #67989 ), #82541, .F. ) ;
#65486=DIRECTION ( 'NONE',  ( -1.000000000000000000, 0.000000000000000000, 1.047445008332813989E-14 ) ) ;
#65496=CARTESIAN_POINT ( 'NONE',  ( -31.75000000000000000, 8.255000000000000782, 3.175000000000219647 ) ) ;
#65541=EDGE_LOOP ( 'NONE', ( #48242, #1331, #72299, #28534 ) ) ;
#65554=VECTOR ( 'NONE', #28545, 1000.000000000000000 ) ;
#65557=EDGE_CURVE ( 'NONE', #64158, #5232, #82983, .T. ) ;
#65581=ORIENTED_EDGE ( 'NONE', *, *, #29520, .F. ) ;
#65582=EDGE_CURVE ( 'NONE', #51180, #23464, #47969, .T. ) ;
#65621=DIRECTION ( 'NONE',  ( 0.000000000000000000, 0.000000000000000000, 1.000000000000000000 ) ) ;
#65669=VERTEX_POINT ( 'NONE', #64754 ) ;
#65673=CARTESIAN_POINT ( 'NONE',  ( 196.2150000000000034, 43.68799999999999528, 44.45000000000000284 ) ) ;
#65675=AXIS2_PLACEMENT_3D ( 'NONE', #51515, #64723, #78819 ) ;
#65698=ORIENTED_EDGE ( 'NONE', *, *, #78125, .T. ) ;
#65725=VERTEX_POINT ( 'NONE', #83413 ) ;
#65738=CARTESIAN_POINT ( 'NONE',  ( 173.9900000000000091, 20.32000000000000028, -71.37400000000000944 ) ) ;
#65740=VECTOR ( 'NONE', #64405, 1000.000000000000000 ) ;
#65753=ORIENTED_EDGE ( 'NONE', *, *, #84262, .F. ) ;
#65769=EDGE_CURVE ( 'NONE', #36938, #86605, #49765, .T. ) ;
#65772=CARTESIAN_POINT ( 'NONE',  ( -148.0533267522752112, 0.000000000000000000, 160.2664750769289697 ) ) ;
#65782=CARTESIAN_POINT ( 'NONE',  ( 124.4917145262460565, 58.80722411771389346, -39.32846460224703833 ) ) ;
#65803=CARTESIAN_POINT ( 'NONE',  ( 1.978343425214599878E-14, 0.000000000000000000, 161.5439999999999827 ) ) ;
#65812=ORIENTED_EDGE ( 'NONE', *, *, #44313, .F. ) ;
#65823=DIRECTION ( 'NONE',  ( 0.000000000000000000, 1.000000000000000000, 0.000000000000000000 ) ) ;
#65829=CARTESIAN_POINT ( 'NONE',  ( 122.2627588294752030, 73.99831669748220975, 45.79086873724280338 ) ) ;
#65841=ORIENTED_EDGE ( 'NONE', *, *, #30339, .T. ) ;
#65855=DIRECTION ( 'NONE',  ( 1.000000000000000000, 0.000000000000000000, -2.505701470911820065E-15 ) ) ;
#65902=LINE ( 'NONE', #73163, #50487 ) ;
#65930=DIRECTION ( 'NONE',  ( 0.000000000000000000, 1.000000000000000000, 0.000000000000000000 ) ) ;
#65938=ORIENTED_EDGE ( 'NONE', *, *, #41731, .T. ) ;
#65971=CARTESIAN_POINT ( 'NONE',  ( 2.820233448801842346, 94.93988138122190890, 130.5258113771150192 ) ) ;
#66001=VERTEX_POINT ( 'NONE', #76030 ) ;
#66005=DIRECTION ( 'NONE',  ( 0.000000000000000000, -1.000000000000000000, 0.000000000000000000 ) ) ;
#66023=ORIENTED_EDGE ( 'NONE', *, *, #50108, .T. ) ;
#66040=DIRECTION ( 'NONE',  ( 0.000000000000000000, 0.000000000000000000, 1.000000000000000000 ) ) ;
#66074=FACE_OUTER_BOUND ( 'NONE', #58846, .T. ) ;
#66109=CARTESIAN_POINT ( 'NONE',  ( -7.735609141604705030, 92.62441004919340060, 130.3265751744775400 ) ) ;
#66115=CARTESIAN_POINT ( 'NONE',  ( 126.7715183016628657, 47.48007084238671638, 31.20684018435030538 ) ) ;
#66205=DIRECTION ( 'NONE',  ( 0.000000000000000000, 0.000000000000000000, -1.000000000000000000 ) ) ;
#66215=AXIS2_PLACEMENT_3D ( 'NONE', #72859, #31963, #74647 ) ;
#66224=CARTESIAN_POINT ( 'NONE',  ( 120.7589990805706037, 58.78128315956222139, -49.62150920525567699 ) ) ;
#66248=DIRECTION ( 'NONE',  ( 1.000000000000000000, 0.000000000000000000, -4.277118011829300531E-15 ) ) ;
#66254=FACE_OUTER_BOUND ( 'NONE', #54325, .T. ) ;
#66264=CARTESIAN_POINT ( 'NONE',  ( 173.9900000000000091, 101.5999999999999943, 71.37400000000000944 ) ) ;
#66269=CARTESIAN_POINT ( 'NONE',  ( 115.5056795903910825, 72.00002230228413680, 60.85563221252769495 ) ) ;
#66298=ORIENTED_EDGE ( 'NONE', *, *, #52564, .F. ) ;
#66344=DIRECTION ( 'NONE',  ( -1.000000000000000000, 0.000000000000000000, 0.000000000000000000 ) ) ;
#66349=DIRECTION ( 'NONE',  ( 0.000000000000000000, 0.000000000000000000, -1.000000000000000000 ) ) ;
#66356=VERTEX_POINT ( 'NONE', #30124 ) ;
#66358=CARTESIAN_POINT ( 'NONE',  ( 1.978343425214599878E-14, 0.000000000000000000, 161.5439999999999827 ) ) ;
#66380=DIRECTION ( 'NONE',  ( 1.000000000000000000, 0.000000000000000000, 2.671820169801660301E-13 ) ) ;
#66418=ORIENTED_EDGE ( 'NONE', *, *, #25449, .F. ) ;
#66420=CARTESIAN_POINT ( 'NONE',  ( 12.69999999999999929, 82.54999999999999716, 129.9368274816650057 ) ) ;
#66446=CARTESIAN_POINT ( 'NONE',  ( -215.9000000000000057, 101.5999999999999943, -45.33899999999999864 ) ) ;
#66449=VERTEX_POINT ( 'NONE', #57821 ) ;
#66460=VERTEX_POINT ( 'NONE', #74576 ) ;
#66461=ORIENTED_EDGE ( 'NONE', *, *, #27630, .F. ) ;
#66477=VERTEX_POINT ( 'NONE', #12358 ) ;
#66504=CARTESIAN_POINT ( 'NONE',  ( -5.491540717450776654, 69.94491574763448227, 37.72695927949112615 ) ) ;
#66508=DIRECTION ( 'NONE',  ( 0.000000000000000000, -1.000000000000000000, 0.000000000000000000 ) ) ;
#66528=CARTESIAN_POINT ( 'NONE',  ( 0.000000000000000000, 2.031999999999865025, 25.39999999999999858 ) ) ;
#66539=ORIENTED_EDGE ( 'NONE', *, *, #61172, .F. ) ;
#66565=CARTESIAN_POINT ( 'NONE',  ( 183.5150000000000148, 37.33800000000000097, 69.13087104677069306 ) ) ;
#66568=CIRCLE ( 'NONE', #27399, 218.1859999999999786 ) ;
#66596=EDGE_CURVE ( 'NONE', #74769, #73841, #14152, .T. ) ;
#66625=DIRECTION ( 'NONE',  ( -1.000000000000000000, 0.000000000000000000, 0.000000000000000000 ) ) ;
#66627=DIRECTION ( 'NONE',  ( 0.000000000000000000, 1.000000000000000000, 0.000000000000000000 ) ) ;
#66638=LINE ( 'NONE', #58916, #38048 ) ;
#66654=VERTEX_POINT ( 'NONE', #28207 ) ;
#66656=VECTOR ( 'NONE', #27185, 1000.000000000000000 ) ;
#66660=CARTESIAN_POINT ( 'NONE',  ( -187.8075999999999794, 0.000000000000000000, -6.349999999999999645 ) ) ;
#66704=CARTESIAN_POINT ( 'NONE',  ( -187.8075999999999794, 20.32000000000000028, -3.174999999999999822 ) ) ;
#66728=CARTESIAN_POINT ( 'NONE',  ( 114.8489081444445645, 71.25364465473249709, 62.08545131505363202 ) ) ;
#66732=ADVANCED_FACE ( 'NONE', ( #73 ), #57254, .F. ) ;
#66777=ORIENTED_EDGE ( 'NONE', *, *, #65217, .F. ) ;
#66813=LINE ( 'NONE', #81809, #58744 ) ;
#66814=CARTESIAN_POINT ( 'NONE',  ( 0.000000000000000000, 0.000000000000000000, 0.000000000000000000 ) ) ;
#66821=DIRECTION ( 'NONE',  ( 0.000000000000000000, -1.000000000000000000, 0.000000000000000000 ) ) ;
#66825=FACE_OUTER_BOUND ( 'NONE', #77591, .T. ) ;
#66830=DIRECTION ( 'NONE',  ( 0.000000000000000000, 0.000000000000000000, 1.000000000000000000 ) ) ;
#66837=PLANE ( 'NONE',  #71665 ) ;
#66840=EDGE_CURVE ( 'NONE', #17885, #26732, #31792, .T. ) ;
#66873=CARTESIAN_POINT ( 'NONE',  ( 8.586325160335727347, 91.92393960641707906, 130.2739338507628020 ) ) ;
#66908=LINE ( 'NONE', #32831, #79336 ) ;
#66930=LINE ( 'NONE', #4711, #20330 ) ;
#66936=FACE_OUTER_BOUND ( 'NONE', #2242, .T. ) ;
#66965=DIRECTION ( 'NONE',  ( 3.213938816075602116E-15, 0.000000000000000000, 1.000000000000000000 ) ) ;
#66966=CARTESIAN_POINT ( 'NONE',  ( -186.2398777604659870, 101.5999999999999943, 107.9500000000000028 ) ) ;
#66987=CARTESIAN_POINT ( 'NONE',  ( 20.90327949605574887, 45.74637997433028858, 31.85781312205738303 ) ) ;
#66991=CARTESIAN_POINT ( 'NONE',  ( -31.75000000000000000, 17.78000000000000114, -3.174999999999779998 ) ) ;
#67006=DIRECTION ( 'NONE',  ( 0.000000000000000000, -1.000000000000000000, 0.000000000000000000 ) ) ;
#67019=DIRECTION ( 'NONE',  ( 0.000000000000000000, -1.000000000000000000, 0.000000000000000000 ) ) ;
#67021=EDGE_CURVE ( 'NONE', #34082, #75654, #81756, .T. ) ;
#67052=DIRECTION ( 'NONE',  ( 0.000000000000000000, -0.000000000000000000, -1.000000000000000000 ) ) ;
#67054=FACE_OUTER_BOUND ( 'NONE', #10967, .T. ) ;
#67062=DIRECTION ( 'NONE',  ( 0.000000000000000000, 0.000000000000000000, 1.000000000000000000 ) ) ;
#67073=CARTESIAN_POINT ( 'NONE',  ( 33.98325472291465132, 17.78000000000000114, 3.174999999999999822 ) ) ;
#67078=CARTESIAN_POINT ( 'NONE',  ( 183.5150000000000148, 37.33800000000000097, 69.13087104677069306 ) ) ;
#67131=CARTESIAN_POINT ( 'NONE',  ( 119.6090684540881171, 53.82079221388885770, -52.33119174590274270 ) ) ;
#67135=ORIENTED_EDGE ( 'NONE', *, *, #60025, .T. ) ;
#67148=ORIENTED_EDGE ( 'NONE', *, *, #51911, .F. ) ;
#67164=CARTESIAN_POINT ( 'NONE',  ( 196.2150000000000034, 30.98800000000000310, 57.14999999999999858 ) ) ;
#67169=CARTESIAN_POINT ( 'NONE',  ( -194.1576000000000022, 101.5999999999999943, -45.33899999999999864 ) ) ;
#67174=CARTESIAN_POINT ( 'NONE',  ( 115.0304089598074171, 71.47004980129892715, 61.74880860687861173 ) ) ;
#67196=DIRECTION ( 'NONE',  ( 0.000000000000000000, -1.000000000000000000, 0.000000000000000000 ) ) ;
#67199=ORIENTED_EDGE ( 'NONE', *, *, #44125, .T. ) ;
#67255=ORIENTED_EDGE ( 'NONE', *, *, #43447, .T. ) ;
#67258=LINE ( 'NONE', #5042, #71810 ) ;
#67282=ORIENTED_EDGE ( 'NONE', *, *, #88385, .T. ) ;
#67314=CARTESIAN_POINT ( 'NONE',  ( 11.32062350639499293, 88.30991999289778960, 130.0643505849274391 ) ) ;
#67316=CIRCLE ( 'NONE', #4962, 25.39999999999999858 ) ;
#67324=CARTESIAN_POINT ( 'NONE',  ( -187.8075999999999794, 101.5999999999999943, 107.9500000000000028 ) ) ;
#67342=ORIENTED_EDGE ( 'NONE', *, *, #6030, .F. ) ;
#67370=AXIS2_PLACEMENT_3D ( 'NONE', #38500, #38951, #73929 ) ;
#67371=VERTEX_POINT ( 'NONE', #23997 ) ;
#67392=CARTESIAN_POINT ( 'NONE',  ( -22.33653601812255474, 59.36077262818345446, 30.86733950792826775 ) ) ;
#67399=CARTESIAN_POINT ( 'NONE',  ( -160.2664750769284865, 0.000000000000000000, 148.0533267522753818 ) ) ;
#67400=DIRECTION ( 'NONE',  ( 0.000000000000000000, -1.000000000000000000, 0.000000000000000000 ) ) ;
#67427=DIRECTION ( 'NONE',  ( 0.000000000000000000, 0.000000000000000000, -1.000000000000000000 ) ) ;
#67443=DIRECTION ( 'NONE',  ( 0.000000000000000000, 0.000000000000000000, -1.000000000000000000 ) ) ;
#67450=AXIS2_PLACEMENT_3D ( 'NONE', #65310, #24428, #73906 ) ;
#67474=DIRECTION ( 'NONE',  ( 1.000000000000000000, 0.000000000000000000, 0.000000000000000000 ) ) ;
#67504=CARTESIAN_POINT ( 'NONE',  ( -7.017469736778876310, 71.96484654754983978, 130.3672675077506256 ) ) ;
#67527=DIRECTION ( 'NONE',  ( 0.000000000000000000, 1.000000000000000000, 0.000000000000000000 ) ) ;
#67546=LINE ( 'NONE', #41500, #48999 ) ;
#67572=EDGE_CURVE ( 'NONE', #14773, #37741, #49689, .T. ) ;
#67580=DIRECTION ( 'NONE',  ( 0.000000000000000000, 1.000000000000000000, 0.000000000000000000 ) ) ;
#67582=ORIENTED_EDGE ( 'NONE', *, *, #46067, .F. ) ;
#67584=CARTESIAN_POINT ( 'NONE',  ( 124.0808947512391711, 59.70268277206753282, -40.60803669063014354 ) ) ;
#67615=VERTEX_POINT ( 'NONE', #62077 ) ;
#67627=LINE ( 'NONE', #27634, #81420 ) ;
#67629=VERTEX_POINT ( 'NONE', #69355 ) ;
#67630=DIRECTION ( 'NONE',  ( 0.000000000000000000, 0.000000000000000000, -1.000000000000000000 ) ) ;
#67638=EDGE_CURVE ( 'NONE', #52633, #51180, #56217, .T. ) ;
#67709=AXIS2_PLACEMENT_3D ( 'NONE', #46333, #61317, #68150 ) ;
#67728=ORIENTED_EDGE ( 'NONE', *, *, #50234, .F. ) ;
#67733=CYLINDRICAL_SURFACE ( 'NONE', #30097, 7.873999999999991672 ) ;
#67751=ORIENTED_EDGE ( 'NONE', *, *, #19256, .T. ) ;
#67760=LINE ( 'NONE', #80507, #37139 ) ;
#67779=DIRECTION ( 'NONE',  ( 0.000000000000000000, 0.000000000000000000, 1.000000000000000000 ) ) ;
#67812=DIRECTION ( 'NONE',  ( -3.491483361109380094E-15, 0.000000000000000000, -1.000000000000000000 ) ) ;
#67825=CYLINDRICAL_SURFACE ( 'NONE', #72662, 7.873999999999991672 ) ;
#67832=ORIENTED_EDGE ( 'NONE', *, *, #70408, .T. ) ;
#67877=CYLINDRICAL_SURFACE ( 'NONE', #38522, 34.13125000000000142 ) ;
#67878=DIRECTION ( 'NONE',  ( 0.000000000000000000, -1.000000000000000000, 0.000000000000000000 ) ) ;
#67884=CARTESIAN_POINT ( 'NONE',  ( 23.25885318707441485, 53.08705262765686683, 30.17677895551207001 ) ) ;
#67895=ORIENTED_EDGE ( 'NONE', *, *, #55241, .T. ) ;
#67935=CARTESIAN_POINT ( 'NONE',  ( -109.2774118001976120, 53.97500000000000142, 71.43750000000000000 ) ) ;
#67963=CARTESIAN_POINT ( 'NONE',  ( -6.975949578566201126, 71.93738766389279249, 130.3694979861350873 ) ) ;
#67976=ADVANCED_FACE ( 'NONE', ( #57684 ), #9545, .F. ) ;
#67979=CIRCLE ( 'NONE', #76731, 34.13125000000000142 ) ;
#67989=FACE_OUTER_BOUND ( 'NONE', #8022, .T. ) ;
#68023=VECTOR ( 'NONE', #41730, 999.9999999999998863 ) ;
#68027=EDGE_CURVE ( 'NONE', #42257, #66654, #1137, .T. ) ;
#68094=EDGE_CURVE ( 'NONE', #75654, #63113, #11315, .T. ) ;
#68130=VECTOR ( 'NONE', #43773, 1000.000000000000000 ) ;
#68146=ORIENTED_EDGE ( 'NONE', *, *, #64289, .F. ) ;
#68150=DIRECTION ( 'NONE',  ( 0.000000000000000000, 0.000000000000000000, 1.000000000000000000 ) ) ;
#68155=CARTESIAN_POINT ( 'NONE',  ( 7.064474567469056332, 71.99617586329878804, 130.3647280704349782 ) ) ;
#68159=AXIS2_PLACEMENT_3D ( 'NONE', #29427, #43025, #14459 ) ;
#68164=ORIENTED_EDGE ( 'NONE', *, *, #38700, .F. ) ;
#68180=VECTOR ( 'NONE', #9521, 1000.000000000000114 ) ;
#68194=DIRECTION ( 'NONE',  ( 0.000000000000000000, -1.000000000000000000, 0.000000000000000000 ) ) ;
#68233=CARTESIAN_POINT ( 'NONE',  ( 11.69661972370231773, 87.49773257406484106, 130.0309910664321649 ) ) ;
#68236=DIRECTION ( 'NONE',  ( 0.000000000000000000, 1.000000000000000000, 0.000000000000000000 ) ) ;
#68291=ORIENTED_EDGE ( 'NONE', *, *, #76638, .T. ) ;
#68293=DIRECTION ( 'NONE',  ( 0.000000000000000000, 0.000000000000000000, 1.000000000000000000 ) ) ;
#68313=LINE ( 'NONE', #26978, #3210 ) ;
#68392=CARTESIAN_POINT ( 'NONE',  ( -125.0340203103765759, 69.82055466749729078, 37.56983117113036030 ) ) ;
#68415=EDGE_CURVE ( 'NONE', #7688, #72189, #16634, .T. ) ;
#68417=DIRECTION ( 'NONE',  ( 0.000000000000000000, -1.000000000000000000, 0.000000000000000000 ) ) ;
#68419=CARTESIAN_POINT ( 'NONE',  ( -6.727371441648950956, 71.77714599857043254, 130.3826064408659704 ) ) ;
#68429=AXIS2_PLACEMENT_3D ( 'NONE', #53518, #39913, #67630 ) ;
#68452=CARTESIAN_POINT ( 'NONE',  ( -126.9619601814429046, 50.67986003389061267, 30.42261724897560882 ) ) ;
#68474=CIRCLE ( 'NONE', #4664, 34.13125000000000142 ) ;
#68516=LINE ( 'NONE', #61679, #53433 ) ;
#68552=ORIENTED_EDGE ( 'NONE', *, *, #50743, .F. ) ;
#68553=AXIS2_PLACEMENT_3D ( 'NONE', #7873, #35569, #56910 ) ;
#68565=ORIENTED_EDGE ( 'NONE', *, *, #84883, .T. ) ;
#68593=EDGE_CURVE ( 'NONE', #84402, #44354, #44755, .T. ) ;
#68607=CARTESIAN_POINT ( 'NONE',  ( 4.881240125921706863, 70.82551138040557248, 130.4647181642625924 ) ) ;
#68613=CARTESIAN_POINT ( 'NONE',  ( 121.0092027855660035, 46.23352279840064938, -49.00708929922899415 ) ) ;
#68616=EDGE_LOOP ( 'NONE', ( #76164, #67832, #17335, #39771, #15734, #32564 ) ) ;
#68636=DIRECTION ( 'NONE',  ( 0.000000000000000000, -1.000000000000000000, 0.000000000000000000 ) ) ;
#68640=DIRECTION ( 'NONE',  ( 0.000000000000000000, -1.000000000000000000, 0.000000000000000000 ) ) ;
#68662=DIRECTION ( 'NONE',  ( 0.000000000000000000, 0.000000000000000000, 1.000000000000000000 ) ) ;
#68663=FACE_OUTER_BOUND ( 'NONE', #77460, .T. ) ;
#68665=ADVANCED_FACE ( 'NONE', ( #205 ), #22012, .F. ) ;
#68674=DIRECTION ( 'NONE',  ( 0.000000000000000000, 0.000000000000000000, 1.000000000000000000 ) ) ;
#68684=EDGE_CURVE ( 'NONE', #64158, #19304, #67979, .T. ) ;
#68704=ORIENTED_EDGE ( 'NONE', *, *, #89710, .T. ) ;
#68723=ORIENTED_EDGE ( 'NONE', *, *, #80865, .T. ) ;
#68725=PLANE ( 'NONE',  #26227 ) ;
#68739=CARTESIAN_POINT ( 'NONE',  ( -50.03799999999999670, 101.5999999999999943, 206.3750000000000000 ) ) ;
#68741=CARTESIAN_POINT ( 'NONE',  ( 126.8507000869722390, 59.56822751209651301, 30.88457633610675046 ) ) ;
#68745=ORIENTED_EDGE ( 'NONE', *, *, #27093, .F. ) ;
#68787=FACE_OUTER_BOUND ( 'NONE', #49354, .T. ) ;
#68804=AXIS2_PLACEMENT_3D ( 'NONE', #64961, #8212, #44048 ) ;
#68814=DIRECTION ( 'NONE',  ( 0.000000000000000000, 1.000000000000000000, 0.000000000000000000 ) ) ;
#68833=CARTESIAN_POINT ( 'NONE',  ( -215.9010000000000105, 52.73749999999999716, -44.45000000000000284 ) ) ;
#68837=CARTESIAN_POINT ( 'NONE',  ( -119.9775062457194537, 74.60142784138798788, 51.48081989348475673 ) ) ;
#68838=ORIENTED_EDGE ( 'NONE', *, *, #15951, .F. ) ;
#68856=ORIENTED_EDGE ( 'NONE', *, *, #59717, .F. ) ;
#68857=AXIS2_PLACEMENT_3D ( 'NONE', #56769, #924, #22274 ) ;
#68860=CARTESIAN_POINT ( 'NONE',  ( -11.03427668835723274, 76.24857023526358546, 130.0890678893988763 ) ) ;
#68862=DIRECTION ( 'NONE',  ( 0.000000000000000000, 0.000000000000000000, 1.000000000000000000 ) ) ;
#68874=ADVANCED_FACE ( 'NONE', ( #32818 ), #60514, .F. ) ;
#68895=ORIENTED_EDGE ( 'NONE', *, *, #39746, .F. ) ;
#68898=VECTOR ( 'NONE', #56376, 1000.000000000000000 ) ;
#68926=EDGE_CURVE ( 'NONE', #25618, #75654, #11435, .T. ) ;
#68939=DIRECTION ( 'NONE',  ( 0.000000000000000000, -1.000000000000000000, 0.000000000000000000 ) ) ;
#68960=CARTESIAN_POINT ( 'NONE',  ( 1.415352702357284018E-13, 20.32000000000000028, -179.8898777604655095 ) ) ;
#68962=CARTESIAN_POINT ( 'NONE',  ( -158.9822249764575020, 20.32000000000000028, 139.6999999999999886 ) ) ;
#68971=DIRECTION ( 'NONE',  ( 1.000000000000000000, 0.000000000000000000, 0.000000000000000000 ) ) ;
#69007=CARTESIAN_POINT ( 'NONE',  ( 1.888034891575249936E-14, 11.42999999999999972, 154.1697486074984909 ) ) ;
#69017=CARTESIAN_POINT ( 'NONE',  ( 173.9900000000000091, 53.21300000000000097, 41.63456447661469895 ) ) ;
#69047=CARTESIAN_POINT ( 'NONE',  ( 6.677588726327760682, 71.73758720873208006, 130.3856720512892764 ) ) ;
#69059=CARTESIAN_POINT ( 'NONE',  ( 0.000000000000000000, 0.000000000000000000, 0.000000000000000000 ) ) ;
#69068=CARTESIAN_POINT ( 'NONE',  ( 173.9900000000000091, 37.33800000000000097, 58.73749999999999716 ) ) ;
#69075=AXIS2_PLACEMENT_3D ( 'NONE', #88709, #33281, #11043 ) ;
#69093=CARTESIAN_POINT ( 'NONE',  ( 173.9900000000000091, 101.5999999999999943, -71.37400000000000944 ) ) ;
#69138=VECTOR ( 'NONE', #66627, 1000.000000000000000 ) ;
#69149=CARTESIAN_POINT ( 'NONE',  ( -3.175000000000109956, 17.78000000000000114, -31.75000000000000000 ) ) ;
#69150=VERTEX_POINT ( 'NONE', #52124 ) ;
#69162=EDGE_CURVE ( 'NONE', #39686, #10389, #38961, .T. ) ;
#69176=ORIENTED_EDGE ( 'NONE', *, *, #424, .F. ) ;
#69215=ORIENTED_EDGE ( 'NONE', *, *, #86750, .F. ) ;
#69223=AXIS2_PLACEMENT_3D ( 'NONE', #16798, #31296, #18569 ) ;
#69233=B_SPLINE_CURVE_WITH_KNOTS ( 'NONE', 3,
 ( #36804, #35442, #16364, #77696, #64955, #68741, #44041, #2739, #15480, #2292, #84071, #50417, #43149, #7751, #15920, #77249, #63158, #78160, #57686, #63612, #15019, #1393, #36358, #42693, #84530, #43597, #70890, #8660, #70434, #85429, #1844, #28637, #71776, #50871, #29542, #9547, #940, #65829, #4513, #72222, #87189, #10873, #37702, #73543, #4956, #32201, #59455, #45814, #59898, #79494, #73995, #86294, #45376, #60348, #52177, #3613, #44490, #38571, #88086, #66269, #87630, #67174, #24513, #66728, #11317, #9993, #53060, #86742, #11774, #16808, #80830, #39471, #32652, #25394, #73095, #4060, #24953, #65401, #51296, #18579, #46259, #17256, #79043, #3181, #30880, #44936, #58564, #24074, #52620, #31759, #39018, #79940, #72666, #51744, #31308, #10433, #38136, #59004, #17696, #80381, #18130, #76232 ),
 .UNSPECIFIED., .F., .F.,
 ( 4, 2, 2, 2, 2, 1, 2, 2, 2, 2, 2, 2, 1, 2, 2, 2, 1, 1, 2, 2, 2, 1, 2, 2, 1, 1, 1, 2, 2, 2, 2, 2, 2, 2, 1, 1, 2, 2, 2, 1, 1, 2, 2, 2, 1, 1, 1, 2, 2, 2, 1, 1, 1, 2, 2, 2, 1, 1, 2, 2, 4 ),
 ( 0.000000000000000000, 0.03124999999999782813, 0.06249999999999565625, 0.1249999999999916456, 0.1562499999999896472, 0.1718749999999886480, 0.1796874999999883982, 0.1874999999999881484, 0.2187499999999845957, 0.2343749999999827083, 0.2499999999999808209, 0.2812499999999776845, 0.2968749999999760192, 0.3046874999999750755, 0.3124999999999740763, 0.3437499999999703570, 0.3593749999999687472, 0.3671874999999680256, 0.3710937499999676925, 0.3749999999999674150, 0.4062499999999646394, 0.4218749999999635292, 0.4296874999999631961, 0.4374999999999628630, 0.4687499999999621969, 0.4843749999999618638, 0.4921874999999616973, 0.4960937499999618638, 0.4999999999999620304, 0.5312499999999621414, 0.5624999999999623634, 0.5937499999999624745, 0.6249999999999626965, 0.6562499999999628075, 0.6718749999999631406, 0.6796874999999633626, 0.6835937499999635847, 0.6874999999999639178, 0.7187499999999693578, 0.7343749999999724665, 0.7421874999999742428, 0.7460937499999750200, 0.7499999999999756861, 0.7812499999999787947, 0.7968749999999805711, 0.8046874999999814593, 0.8085937499999823475, 0.8105468749999829026, 0.8124999999999833467, 0.8437499999999903411, 0.8593749999999934497, 0.8671874999999950040, 0.8710937499999956701, 0.8730468749999957812, 0.8749999999999960032, 0.9062499999999967804, 0.9218749999999971134, 0.9296874999999972244, 0.9335937499999974465, 0.9374999999999975575, 1.000000000000000000 ),
 .UNSPECIFIED. ) ;
#69241=LINE ( 'NONE', #7461, #9924 ) ;
#69242=DIRECTION ( 'NONE',  ( 0.000000000000000000, -0.000000000000000000, 1.000000000000000000 ) ) ;
#69248=EDGE_CURVE ( 'NONE', #66449, #6147, #5352, .T. ) ;
#69259=ORIENTED_EDGE ( 'NONE', *, *, #3756, .T. ) ;
#69270=ADVANCED_FACE ( 'NONE', ( #33046 ), #34386, .F. ) ;
#69282=AXIS2_PLACEMENT_3D ( 'NONE', #17582, #45266, #38454 ) ;
#69286=DIRECTION ( 'NONE',  ( 0.000000000000000000, 0.000000000000000000, 1.000000000000000000 ) ) ;
#69287=CARTESIAN_POINT ( 'NONE',  ( -121.3915910346715492, 74.42942291849823278, 48.05185983205323907 ) ) ;
#69313=CARTESIAN_POINT ( 'NONE',  ( -8.784747902566598654, 73.37422592973923940, 130.2602619110634521 ) ) ;
#69337=CARTESIAN_POINT ( 'NONE',  ( 183.5150000000000148, 53.21300000000000097, 59.96543552338529537 ) ) ;
#69355=CARTESIAN_POINT ( 'NONE',  ( 0.000000000000000000, 8.255000000000000782, 25.39999999999999858 ) ) ;
#69359=ORIENTED_EDGE ( 'NONE', *, *, #70288, .F. ) ;
#69369=CARTESIAN_POINT ( 'NONE',  ( -12.10688491755598939, 86.39173550988738270, 129.9936122529997249 ) ) ;
#69374=TOROIDAL_SURFACE ( 'NONE', #88251, 154.1697486074984909, 6.349999999999999645 ) ;
#69431=CARTESIAN_POINT ( 'NONE',  ( 109.4488842849793997, 50.66243909899585418, 71.17456644476511940 ) ) ;
#69433=EDGE_LOOP ( 'NONE', ( #3723, #20431, #41753, #39078 ) ) ;
#69437=CARTESIAN_POINT ( 'NONE',  ( 0.000000000000000000, 44.45000000000000284, 38.10000000000000142 ) ) ;
#69444=DIRECTION ( 'NONE',  ( 1.000000000000000000, 0.000000000000000000, 0.000000000000000000 ) ) ;
#69450=DIRECTION ( 'NONE',  ( 0.000000000000000000, 0.000000000000000000, 1.000000000000000000 ) ) ;
#69461=AXIS2_PLACEMENT_3D ( 'NONE', #72733, #35973, #36872 ) ;
#69493=LINE ( 'NONE', #56281, #8321 ) ;
#69499=CARTESIAN_POINT ( 'NONE',  ( 3.226834594885171104, 70.23869239023346722, 130.5183031135091483 ) ) ;
#69507=CARTESIAN_POINT ( 'NONE',  ( 120.9243902208823584, 46.38490584264999228, -49.21592832199778655 ) ) ;
#69515=EDGE_CURVE ( 'NONE', #21770, #31466, #11550, .T. ) ;
#69520=CARTESIAN_POINT ( 'NONE',  ( 170.2205283966864897, 101.5999999999999943, 71.37400000000000944 ) ) ;
#69523=VECTOR ( 'NONE', #31335, 1000.000000000000000 ) ;
#69543=DIRECTION ( 'NONE',  ( 1.000000000000000000, 0.000000000000000000, 4.811757763307910244E-15 ) ) ;
#69582=DIRECTION ( 'NONE',  ( 0.000000000000000000, 0.8660254037844387076, -0.4999999999999998890 ) ) ;
#69602=EDGE_CURVE ( 'NONE', #60012, #18422, #78885, .T. ) ;
#69603=ORIENTED_EDGE ( 'NONE', *, *, #66596, .F. ) ;
#69610=EDGE_LOOP ( 'NONE', ( #76199, #50841, #49536 ) ) ;
#69624=EDGE_CURVE ( 'NONE', #45185, #849, #72059, .T. ) ;
#69631=DIRECTION ( 'NONE',  ( 0.000000000000000000, 0.000000000000000000, 1.000000000000000000 ) ) ;
#69638=LINE ( 'NONE', #7407, #54040 ) ;
#69651=CARTESIAN_POINT ( 'NONE',  ( 10.61518134898173216, 75.57796106687908377, 130.1237400822467407 ) ) ;
#69655=FACE_OUTER_BOUND ( 'NONE', #50161, .T. ) ;
#69659=FACE_OUTER_BOUND ( 'NONE', #52433, .T. ) ;
#69673=FACE_OUTER_BOUND ( 'NONE', #57047, .T. ) ;
#69723=ORIENTED_EDGE ( 'NONE', *, *, #27585, .F. ) ;
#69737=CARTESIAN_POINT ( 'NONE',  ( -123.8170101655531425, 72.35301567669330325, 41.40434455345861409 ) ) ;
#69794=ORIENTED_EDGE ( 'NONE', *, *, #52302, .T. ) ;
#69809=ORIENTED_EDGE ( 'NONE', *, *, #73899, .T. ) ;
#69819=CARTESIAN_POINT ( 'NONE',  ( -11.87509116337306025, 87.05477402842780066, 130.0148473914468639 ) ) ;
#69841=VECTOR ( 'NONE', #71133, 1000.000000000000000 ) ;
#69846=VERTEX_POINT ( 'NONE', #62441 ) ;
#69849=EDGE_LOOP ( 'NONE', ( #61504, #76089, #73271, #74005, #80335, #27134 ) ) ;
#69860=DIRECTION ( 'NONE',  ( 0.000000000000000000, 1.000000000000000000, 0.000000000000000000 ) ) ;
#69867=DIRECTION ( 'NONE',  ( 0.000000000000000000, -1.000000000000000000, 0.000000000000000000 ) ) ;
#69877=CARTESIAN_POINT ( 'NONE',  ( 109.6522639851457228, 49.12997694320977615, 70.86078145649237570 ) ) ;
#69889=FACE_OUTER_BOUND ( 'NONE', #26414, .T. ) ;
#69926=EDGE_LOOP ( 'NONE', ( #55, #24014, #76255, #62279, #59747 ) ) ;
#69946=CIRCLE ( 'NONE', #53895, 8.636000000000004562 ) ;
#69951=ORIENTED_EDGE ( 'NONE', *, *, #89872, .F. ) ;
#69956=CARTESIAN_POINT ( 'NONE',  ( 124.3636858901310802, 46.33258218398187722, -39.73348582418787345 ) ) ;
#70008=FACE_OUTER_BOUND ( 'NONE', #20545, .T. ) ;
#70010=LINE ( 'NONE', #7779, #82097 ) ;
#70062=CARTESIAN_POINT ( 'NONE',  ( -194.1576000000000022, 101.5999999999999943, -12.69999999999999929 ) ) ;
#70080=LINE ( 'NONE', #35549, #42639 ) ;
#70094=CIRCLE ( 'NONE', #48276, 6.350000000000659561 ) ;
#70095=CARTESIAN_POINT ( 'NONE',  ( 12.70000000000000107, 81.76374953821583347, 129.9368274816650057 ) ) ;
#70161=EDGE_CURVE ( 'NONE', #21770, #378, #2805, .T. ) ;
#70163=ORIENTED_EDGE ( 'NONE', *, *, #60025, .F. ) ;
#70174=CARTESIAN_POINT ( 'NONE',  ( -111.8086192760389679, 66.24298264774402867, 67.40841616357421628 ) ) ;
#70241=DIRECTION ( 'NONE',  ( 0.000000000000000000, 0.000000000000000000, 1.000000000000000000 ) ) ;
#70242=EDGE_CURVE ( 'NONE', #5474, #33479, #46783, .T. ) ;
#70262=CARTESIAN_POINT ( 'NONE',  ( -11.13171314038108584, 88.66704411686306742, 130.0806558683388801 ) ) ;
#70288=EDGE_CURVE ( 'NONE', #26221, #78242, #89041, .T. ) ;
#70303=ORIENTED_EDGE ( 'NONE', *, *, #56022, .F. ) ;
#70324=CARTESIAN_POINT ( 'NONE',  ( 110.2901544400639722, 45.91391880550399662, 69.86957027353565763 ) ) ;
#70350=EDGE_CURVE ( 'NONE', #72189, #849, #5604, .T. ) ;
#70372=VECTOR ( 'NONE', #5113, 1000.000000000000000 ) ;
#70391=DIRECTION ( 'NONE',  ( -1.000000000000000000, 0.000000000000000000, 0.000000000000000000 ) ) ;
#70405=ORIENTED_EDGE ( 'NONE', *, *, #45571, .F. ) ;
#70408=EDGE_CURVE ( 'NONE', #11616, #23269, #14368, .T. ) ;
#70431=EDGE_CURVE ( 'NONE', #13582, #58432, #89494, .T. ) ;
#70434=CARTESIAN_POINT ( 'NONE',  ( 123.9191631267440528, 72.20435897694871130, 41.10135031971049813 ) ) ;
#70442=ORIENTED_EDGE ( 'NONE', *, *, #50108, .F. ) ;
#70469=ORIENTED_EDGE ( 'NONE', *, *, #5216, .T. ) ;
#70481=CARTESIAN_POINT ( 'NONE',  ( 173.9900000000000091, 20.32000000000000028, -131.6533725204174061 ) ) ;
#70488=CARTESIAN_POINT ( 'NONE',  ( -186.2398777604659870, 101.5999999999999943, 107.9500000000000028 ) ) ;
#70552=CARTESIAN_POINT ( 'NONE',  ( 11.02744467571318054, 76.24661008267737827, 130.0895381633343391 ) ) ;
#70556=DIRECTION ( 'NONE',  ( 0.000000000000000000, 1.000000000000000000, 0.000000000000000000 ) ) ;
#70557=DIRECTION ( 'NONE',  ( 0.000000000000000000, 0.000000000000000000, -1.000000000000000000 ) ) ;
#70592=EDGE_LOOP ( 'NONE', ( #75889, #41646, #19016, #82934 ) ) ;
#70620=ORIENTED_EDGE ( 'NONE', *, *, #31343, .T. ) ;
#70623=ORIENTED_EDGE ( 'NONE', *, *, #48510, .T. ) ;
#70625=EDGE_CURVE ( 'NONE', #2213, #84589, #58041, .T. ) ;
#70638=LINE ( 'NONE', #23401, #82145 ) ;
#70682=DIRECTION ( 'NONE',  ( 0.000000000000000000, 1.000000000000000000, 0.000000000000000000 ) ) ;
#70715=DIRECTION ( 'NONE',  ( 0.000000000000000000, 0.000000000000000000, -1.000000000000000000 ) ) ;
#70720=AXIS2_PLACEMENT_3D ( 'NONE', #87076, #25278, #52506 ) ;
#70723=CIRCLE ( 'NONE', #14108, 218.1859999999999786 ) ;
#70738=DIRECTION ( 'NONE',  ( 0.000000000000000000, 0.000000000000000000, -1.000000000000000000 ) ) ;
#70757=FACE_OUTER_BOUND ( 'NONE', #36860, .T. ) ;
#70780=CARTESIAN_POINT ( 'NONE',  ( -20.82352280117506282, 62.28388828036364799, 31.90676034344724243 ) ) ;
#70806=CIRCLE ( 'NONE', #24372, 7.937500000000000000 ) ;
#70850=DIRECTION ( 'NONE',  ( 0.000000000000000000, 0.000000000000000000, 1.000000000000000000 ) ) ;
#70851=CARTESIAN_POINT ( 'NONE',  ( 131.3179999999999836, 44.45000000000000284, 32.49205688096009936 ) ) ;
#70864=ORIENTED_EDGE ( 'NONE', *, *, #58143, .T. ) ;
#70890=CARTESIAN_POINT ( 'NONE',  ( 124.3463864195482387, 71.42811502680554270, 39.78527854427932198 ) ) ;
#70921=DIRECTION ( 'NONE',  ( 0.000000000000000000, 0.000000000000000000, 1.000000000000000000 ) ) ;
#70936=FACE_OUTER_BOUND ( 'NONE', #31512, .T. ) ;
#70939=DIRECTION ( 'NONE',  ( 1.000000000000000000, 0.000000000000000000, 2.108231265501709878E-16 ) ) ;
#70948=DIRECTION ( 'NONE',  ( -1.000000000000000000, 0.000000000000000000, -7.867884063170659983E-16 ) ) ;
#70973=CIRCLE ( 'NONE', #31785, 218.1859999999999786 ) ;
#70988=CARTESIAN_POINT ( 'NONE',  ( -179.8898777604655095, 0.000000000000000000, -12.69999999999999929 ) ) ;
#71033=VERTEX_POINT ( 'NONE', #61435 ) ;
#71034=EDGE_CURVE ( 'NONE', #48373, #84162, #60997, .T. ) ;
#71052=ORIENTED_EDGE ( 'NONE', *, *, #59088, .F. ) ;
#71125=DIRECTION ( 'NONE',  ( 1.000000000000000000, 0.000000000000000000, 2.108231265501709878E-16 ) ) ;
#71133=DIRECTION ( 'NONE',  ( 0.000000000000000000, -1.000000000000000000, 0.000000000000000000 ) ) ;
#71144=EDGE_LOOP ( 'NONE', ( #83353, #84427, #12630, #49726 ) ) ;
#71174=CARTESIAN_POINT ( 'NONE',  ( -12.29034155828684405, 85.77798403344019107, 129.9765768215993091 ) ) ;
#71178=CARTESIAN_POINT ( 'NONE',  ( 126.4970673974017643, 44.81588728400144106, 32.30169817395221088 ) ) ;
#71181=DIRECTION ( 'NONE',  ( 1.000000000000000000, 0.000000000000000000, -6.982966722218760189E-15 ) ) ;
#71275=EDGE_CURVE ( 'NONE', #21656, #43367, #34070, .T. ) ;
#71277=CIRCLE ( 'NONE', #29184, 9.525000000000000355 ) ;
#71281=ORIENTED_EDGE ( 'NONE', *, *, #71275, .T. ) ;
#71284=VECTOR ( 'NONE', #89222, 1000.000000000000000 ) ;
#71329=CARTESIAN_POINT ( 'NONE',  ( -3.175000000000109956, 8.255000000000000782, -31.75000000000000000 ) ) ;
#71331=CARTESIAN_POINT ( 'NONE',  ( 3.175000000000355094, 8.255000000000000782, 33.98325472291460159 ) ) ;
#71340=ORIENTED_EDGE ( 'NONE', *, *, #39135, .T. ) ;
#71437=EDGE_CURVE ( 'NONE', #19975, #6147, #70973, .T. ) ;
#71455=UNCERTAINTY_MEASURE_WITH_UNIT (LENGTH_MEASURE( 1.000000000000000082E-05 ), #87751, 'distance_accuracy_value', 'NONE');
#71462=CARTESIAN_POINT ( 'NONE',  ( 173.9900000000000091, 53.21300000000000097, 59.96543552338539484 ) ) ;
#71483=AXIS2_PLACEMENT_3D ( 'NONE', #73780, #11565, #5648 ) ;
#71503=CARTESIAN_POINT ( 'NONE',  ( 0.000000000000000000, 8.255000000000000782, 0.000000000000000000 ) ) ;
#71508=CARTESIAN_POINT ( 'NONE',  ( 50.03799999999999670, 101.5999999999999943, 206.3750000000000000 ) ) ;
#71512=ORIENTED_EDGE ( 'NONE', *, *, #57062, .F. ) ;
#71520=AXIS2_PLACEMENT_3D ( 'NONE', #86821, #65031, #23282 ) ;
#71524=DIRECTION ( 'NONE',  ( -1.000000000000000000, 0.000000000000000000, -2.301579500234999682E-14 ) ) ;
#71527=VERTEX_POINT ( 'NONE', #16339 ) ;
#71586=FACE_OUTER_BOUND ( 'NONE', #77680, .T. ) ;
#71619=CARTESIAN_POINT ( 'NONE',  ( 50.03799999999999670, 101.5999999999999943, 206.3750000000000000 ) ) ;
#71652=DIRECTION ( 'NONE',  ( -0.7071067811865370256, 0.000000000000000000, 0.7071067811865580088 ) ) ;
#71664=CARTESIAN_POINT ( 'NONE',  ( 14.46226641585351835, 67.55286469922893389, 35.25428405273846266 ) ) ;
#71665=AXIS2_PLACEMENT_3D ( 'NONE', #74107, #52722, #66380 ) ;
#71698=DIRECTION ( 'NONE',  ( 1.000000000000000000, 0.000000000000000000, 4.811757763307910244E-15 ) ) ;
#71700=DIRECTION ( 'NONE',  ( 8.659560562355369197E-17, 0.7071067811865120456, -0.7071067811865829889 ) ) ;
#71713=VERTEX_POINT ( 'NONE', #16196 ) ;
#71753=DIRECTION ( 'NONE',  ( -1.000000000000000000, 0.000000000000000000, 0.000000000000000000 ) ) ;
#71776=CARTESIAN_POINT ( 'NONE',  ( 123.1816666992336167, 73.18476051486229039, 43.25682771927707648 ) ) ;
#71810=VECTOR ( 'NONE', #32740, 1000.000000000000000 ) ;
#71836=ORIENTED_EDGE ( 'NONE', *, *, #51520, .F. ) ;
#71867=ORIENTED_EDGE ( 'NONE', *, *, #51672, .F. ) ;
#71876=AXIS2_PLACEMENT_3D ( 'NONE', #88021, #81671, #24454 ) ;
#71885=AXIS2_PLACEMENT_3D ( 'NONE', #50338, #9034, #72146 ) ;
#71892=VECTOR ( 'NONE', #54904, 1000.000000000000000 ) ;
#71947=LINE ( 'NONE', #80108, #68130 ) ;
#71951=ORIENTED_EDGE ( 'NONE', *, *, #57221, .F. ) ;
#71956=DIRECTION ( 'NONE',  ( 0.000000000000000000, -1.000000000000000000, 0.000000000000000000 ) ) ;
#71971=CARTESIAN_POINT ( 'NONE',  ( 196.2150000000000034, 30.98800000000000310, 44.45000000000000284 ) ) ;
#71978=CARTESIAN_POINT ( 'NONE',  ( -126.2750494843262175, 64.71055288310594733, 33.16032879022311164 ) ) ;
#72021=DIRECTION ( 'NONE',  ( 1.000000000000000000, 0.000000000000000000, 0.000000000000000000 ) ) ;
#72045=CARTESIAN_POINT ( 'NONE',  ( -135.1318726873890341, 20.32000000000000028, 118.7423475625884066 ) ) ;
#72049=EDGE_CURVE ( 'NONE', #60012, #11178, #24703, .T. ) ;
#72054=CARTESIAN_POINT ( 'NONE',  ( -7.057748139868313508, 93.10832354271467182, 130.3650924429668407 ) ) ;
#72059=LINE ( 'NONE', #3458, #76534 ) ;
#72061=FACE_OUTER_BOUND ( 'NONE', #1099, .T. ) ;
#72065=STYLED_ITEM ( 'NONE', ( #23704 ), #50495 ) ;
#72105=CARTESIAN_POINT ( 'NONE',  ( 22.34055959819741233, 59.35018981749909983, 30.86443047836608855 ) ) ;
#72118=EDGE_CURVE ( 'NONE', #85626, #79928, #66930, .T. ) ;
#72135=ORIENTED_EDGE ( 'NONE', *, *, #61993, .T. ) ;
#72146=DIRECTION ( 'NONE',  ( 0.000000000000000000, 0.000000000000000000, -1.000000000000000000 ) ) ;
#72167=DIRECTION ( 'NONE',  ( 0.000000000000000000, 0.000000000000000000, -1.000000000000000000 ) ) ;
#72186=ORIENTED_EDGE ( 'NONE', *, *, #17626, .T. ) ;
#72189=VERTEX_POINT ( 'NONE', #46908 ) ;
#72209=DIRECTION ( 'NONE',  ( 0.000000000000000000, 0.000000000000000000, 1.000000000000000000 ) ) ;
#72222=CARTESIAN_POINT ( 'NONE',  ( 121.8942133281728957, 74.21437598052153817, 46.76216900032968482 ) ) ;
#72227=DIRECTION ( 'NONE',  ( 2.108231265501709878E-16, 0.000000000000000000, -1.000000000000000000 ) ) ;
#72299=ORIENTED_EDGE ( 'NONE', *, *, #21901, .T. ) ;
#72313=B_SPLINE_CURVE_WITH_KNOTS ( 'NONE', 3,
 ( #38526, #53925, #80782, #4912, #59852, #88492, #87585, #25343, #24912, #60303, #33057, #80334, #88037, #11730, #65782, #18989, #52575, #67584, #72621, #12179, #60757, #53472, #38975, #53014, #18530, #31264, #44892, #39863, #81240, #26247, #58959, #73953, #86696, #24470, #66224, #52135, #11271, #87143, #79895, #46217, #39426, #17651, #59411, #45327, #73047, #67131, #4013, #18082 ),
 .UNSPECIFIED., .F., .F.,
 ( 4, 2, 2, 2, 2, 2, 2, 2, 2, 2, 2, 2, 2, 2, 2, 2, 2, 2, 2, 2, 2, 2, 2, 4 ),
 ( 1.387778780781445521E-17, 0.001601933432478720850, 0.002402900148718063820, 0.003203866864957407440, 0.004805800297436112895, 0.005606767013675474295, 0.006407733729914834829, 0.007208700446154196230, 0.008009667162393556764, 0.009611600594872257014, 0.01121353402735095726, 0.01281546745982965578, 0.01361643417606901198, 0.01441740089230836991, 0.01601933432478708577, 0.01682030104102645238, 0.01762126775726581898, 0.01922320118974451750, 0.02002416790598385288, 0.02082513462222318826, 0.02162610133846252364, 0.02242706805470186249, 0.02402900148718053325, 0.02563093491965920748 ),
 .UNSPECIFIED. ) ;
#72331=EDGE_LOOP ( 'NONE', ( #50288, #56299, #42557, #66023, #7033, #65841, #87838, #57287, #84485, #30578 ) ) ;
#72383=DIRECTION ( 'NONE',  ( -6.982966722218760189E-15, 0.000000000000000000, -1.000000000000000000 ) ) ;
#72387=DIRECTION ( 'NONE',  ( 0.000000000000000000, -3.785359618865284342E-16, -1.000000000000000000 ) ) ;
#72392=DIRECTION ( 'NONE',  ( 0.000000000000000000, 0.000000000000000000, 1.000000000000000000 ) ) ;
#72397=ORIENTED_EDGE ( 'NONE', *, *, #27567, .T. ) ;
#72419=VERTEX_POINT ( 'NONE', #35528 ) ;
#72421=CARTESIAN_POINT ( 'NONE',  ( -126.5337430658103841, 62.85728282860507221, 32.15843782321050526 ) ) ;
#72425=ORIENTED_EDGE ( 'NONE', *, *, #32706, .T. ) ;
#72457=CARTESIAN_POINT ( 'NONE',  ( 0.000000000000000000, 17.78000000000000114, 0.000000000000000000 ) ) ;
#72475=ORIENTED_EDGE ( 'NONE', *, *, #20798, .T. ) ;
#72520=DIRECTION ( 'NONE',  ( 0.000000000000000000, 0.000000000000000000, -1.000000000000000000 ) ) ;
#72544=EDGE_LOOP ( 'NONE', ( #25993, #15856, #59722, #69359 ) ) ;
#72554=CARTESIAN_POINT ( 'NONE',  ( -179.6205029264235122, 0.000000000000000000, 123.8612349545196025 ) ) ;
#72600=ORIENTED_EDGE ( 'NONE', *, *, #65557, .F. ) ;
#72601=FACE_OUTER_BOUND ( 'NONE', #21141, .T. ) ;
#72619=ORIENTED_EDGE ( 'NONE', *, *, #9906, .T. ) ;
#72621=CARTESIAN_POINT ( 'NONE',  ( 123.9304707123681766, 59.93532171591466096, -41.06530013989648609 ) ) ;
#72631=DIRECTION ( 'NONE',  ( -1.000000000000000000, -8.741913579725640327E-16, -2.913971193241879977E-15 ) ) ;
#72637=ADVANCED_FACE ( 'NONE', ( #73180 ), #24599, .F. ) ;
#72639=VERTEX_POINT ( 'NONE', #59542 ) ;
#72644=FACE_OUTER_BOUND ( 'NONE', #45975, .T. ) ;
#72662=AXIS2_PLACEMENT_3D ( 'NONE', #59652, #72854, #17883 ) ;
#72666=CARTESIAN_POINT ( 'NONE',  ( 110.0341319374553706, 60.86293649591723920, 70.26678365844557561 ) ) ;
#72678=CARTESIAN_POINT ( 'NONE',  ( -194.1576000000000022, 0.000000000000000000, 114.2999999999999972 ) ) ;
#72682=CARTESIAN_POINT ( 'NONE',  ( -194.1576000000000022, 20.32000000000000028, -12.69999999999999929 ) ) ;
#72683=VECTOR ( 'NONE', #2401, 1000.000000000000000 ) ;
#72694=EDGE_CURVE ( 'NONE', #4177, #49608, #33648, .T. ) ;
#72729=ORIENTED_EDGE ( 'NONE', *, *, #5186, .F. ) ;
#72733=CARTESIAN_POINT ( 'NONE',  ( -186.2398777604655038, 101.5999999999999943, -6.349999999999999645 ) ) ;
#72744=B_SPLINE_CURVE_WITH_KNOTS ( 'NONE', 3,
 ( #76692, #42588, #48497, #82182, #69431, #41696, #49409, #42149, #83505, #69877, #14921, #48064, #70324, #19937 ),
 .UNSPECIFIED., .F., .F.,
 ( 4, 2, 2, 1, 1, 2, 2, 4 ),
 ( 0.000000000000000000, 0.2499999999999814593, 0.3749999999999724110, 0.4374999999999666933, 0.4687499999999643618, 0.4843749999999638622, 0.4999999999999633626, 1.000000000000000000 ),
 .UNSPECIFIED. ) ;
#72753=DIRECTION ( 'NONE',  ( 0.000000000000000000, 0.000000000000000000, -1.000000000000000000 ) ) ;
#72756=DIRECTION ( 'NONE',  ( 0.7071067811865604513, 0.000000000000000000, -0.7071067811865344721 ) ) ;
#72757=VERTEX_POINT ( 'NONE', #69520 ) ;
#72804=CARTESIAN_POINT ( 'NONE',  ( 6.114111144840049583, 93.68330544519889713, 130.4128344644624917 ) ) ;
#72810=CARTESIAN_POINT ( 'NONE',  ( 57.91199999999999903, 20.32000000000000028, 191.3008000794699797 ) ) ;
#72835=CYLINDRICAL_SURFACE ( 'NONE', #25554, 9.525000000000000355 ) ;
#72854=DIRECTION ( 'NONE',  ( 0.000000000000000000, -1.000000000000000000, 0.000000000000000000 ) ) ;
#72859=CARTESIAN_POINT ( 'NONE',  ( -3.174999999999664979, 24.56180297284579694, 31.75000000000000000 ) ) ;
#72887=AXIS2_PLACEMENT_3D ( 'NONE', #7094, #34788, #22521 ) ;
#72888=LINE ( 'NONE', #38360, #39733 ) ;
#72919=ORIENTED_EDGE ( 'NONE', *, *, #39135, .F. ) ;
#72928=CARTESIAN_POINT ( 'NONE',  ( -8.592341146638979410, 91.91841160240160491, 130.2735359644163395 ) ) ;
#72948=CARTESIAN_POINT ( 'NONE',  ( 0.000000000000000000, 101.5999999999999943, 0.000000000000000000 ) ) ;
#73010=CIRCLE ( 'NONE', #3442, 7.937500000000000000 ) ;
#73024=ORIENTED_EDGE ( 'NONE', *, *, #424, .T. ) ;
#73047=CARTESIAN_POINT ( 'NONE',  ( 119.7028791468282947, 54.86242404270847572, -52.11625092004412352 ) ) ;
#73053=FACE_OUTER_BOUND ( 'NONE', #48376, .T. ) ;
#73055=CARTESIAN_POINT ( 'NONE',  ( -22.91010569159546151, 50.47404986067924426, 30.44291311365987340 ) ) ;
#73070=ADVANCED_FACE ( 'NONE', ( #62132 ), #6726, .T. ) ;
#73095=CARTESIAN_POINT ( 'NONE',  ( 112.5527812704730337, 67.77553021976281400, 66.15876282107061002 ) ) ;
#73109=CARTESIAN_POINT ( 'NONE',  ( 3.174999999999879918, 8.255000000000000782, -33.98325472291465132 ) ) ;
#73120=DIRECTION ( 'NONE',  ( -0.7071067811865470176, 0.000000000000000000, -0.7071067811865480168 ) ) ;
#73121=DIRECTION ( 'NONE',  ( 0.000000000000000000, 1.000000000000000000, 0.000000000000000000 ) ) ;
#73148=ADVANCED_FACE ( 'NONE', ( #5847 ), #33536, .F. ) ;
#73151=CIRCLE ( 'NONE', #33994, 6.349999999999999645 ) ;
#73153=LINE ( 'NONE', #32261, #63871 ) ;
#73160=ORIENTED_EDGE ( 'NONE', *, *, #26429, .F. ) ;
#73162=CARTESIAN_POINT ( 'NONE',  ( 131.3179999999999836, 44.45000000000000284, 32.49205688096009936 ) ) ;
#73163=CARTESIAN_POINT ( 'NONE',  ( -31.75000000000000000, 17.78000000000000114, 3.175000000000219647 ) ) ;
#73180=FACE_OUTER_BOUND ( 'NONE', #80983, .T. ) ;
#73183=ORIENTED_EDGE ( 'NONE', *, *, #43442, .T. ) ;
#73198=FACE_OUTER_BOUND ( 'NONE', #60429, .T. ) ;
#73247=VECTOR ( 'NONE', #20923, 1000.000000000000000 ) ;
#73271=ORIENTED_EDGE ( 'NONE', *, *, #74707, .F. ) ;
#73292=DIRECTION ( 'NONE',  ( 0.000000000000000000, 0.000000000000000000, 1.000000000000000000 ) ) ;
#73294=ORIENTED_EDGE ( 'NONE', *, *, #47910, .T. ) ;
#73328=PLANE ( 'NONE',  #81844 ) ;
#73364=EDGE_LOOP ( 'NONE', ( #78518, #54247, #18395, #48028 ) ) ;
#73380=ORIENTED_EDGE ( 'NONE', *, *, #88385, .F. ) ;
#73403=ORIENTED_EDGE ( 'NONE', *, *, #75078, .F. ) ;
#73404=AXIS2_PLACEMENT_3D ( 'NONE', #34029, #89468, #27226 ) ;
#73430=ADVANCED_FACE ( 'NONE', ( #59334 ), #24390, .F. ) ;
#73441=LINE ( 'NONE', #31660, #69138 ) ;
#73450=FACE_OUTER_BOUND ( 'NONE', #30391, .T. ) ;
#73535=LINE ( 'NONE', #44930, #12439 ) ;
#73543=CARTESIAN_POINT ( 'NONE',  ( 120.9980108323096317, 74.55612360026276519, 49.04309508044801191 ) ) ;
#73549=CARTESIAN_POINT ( 'NONE',  ( -50.03799999999999670, 0.000000000000000000, 191.3008000794699797 ) ) ;
#73558=AXIS2_PLACEMENT_3D ( 'NONE', #85858, #45805, #58992 ) ;
#73567=DIRECTION ( 'NONE',  ( 0.000000000000000000, 0.000000000000000000, 1.000000000000000000 ) ) ;
#73575=ADVANCED_FACE ( 'NONE', ( #18448, #74326 ), #60216, .T. ) ;
#73595=VERTEX_POINT ( 'NONE', #20261 ) ;
#73612=EDGE_CURVE ( 'NONE', #18423, #20334, #74766, .T. ) ;
#73669=CYLINDRICAL_SURFACE ( 'NONE', #76082, 9.524999999999998579 ) ;
#73680=EDGE_LOOP ( 'NONE', ( #75006, #69809, #8067, #4968 ) ) ;
#73693=ORIENTED_EDGE ( 'NONE', *, *, #74004, .F. ) ;
#73697=CARTESIAN_POINT ( 'NONE',  ( 10.51819778680380146, 89.66744784449326744, 130.1316157236187507 ) ) ;
#73708=EDGE_LOOP ( 'NONE', ( #59479, #22174, #73160, #71281 ) ) ;
#73730=ORIENTED_EDGE ( 'NONE', *, *, #43504, .T. ) ;
#73764=ORIENTED_EDGE ( 'NONE', *, *, #31026, .F. ) ;
#73772=CARTESIAN_POINT ( 'NONE',  ( -20.24703904125878040, 63.07654896400417499, 32.27577670923775344 ) ) ;
#73780=CARTESIAN_POINT ( 'NONE',  ( 75.61066417432020614, 101.5999999999999943, 177.0380000000000109 ) ) ;
#73841=VERTEX_POINT ( 'NONE', #2506 ) ;
#73850=CARTESIAN_POINT ( 'NONE',  ( -109.9641975813423329, 60.51899751744934974, 70.37584683824053400 ) ) ;
#73880=CARTESIAN_POINT ( 'NONE',  ( -3.842181601977885830, 70.44325810012327338, 130.4994487452559611 ) ) ;
#73888=CARTESIAN_POINT ( 'NONE',  ( 50.03799999999999670, 0.000000000000000000, 206.3750000000000000 ) ) ;
#73899=EDGE_CURVE ( 'NONE', #13532, #43158, #14123, .T. ) ;
#73906=DIRECTION ( 'NONE',  ( 1.000000000000000000, 0.000000000000000000, 0.000000000000000000 ) ) ;
#73925=ORIENTED_EDGE ( 'NONE', *, *, #3859, .F. ) ;
#73926=CIRCLE ( 'NONE', #65242, 9.425000000000000711 ) ;
#73929=DIRECTION ( 'NONE',  ( 1.000000000000000000, 0.000000000000000000, 0.000000000000000000 ) ) ;
#73948=DIRECTION ( 'NONE',  ( 0.000000000000000000, 1.000000000000000000, 0.000000000000000000 ) ) ;
#73949=CIRCLE ( 'NONE', #43530, 7.873999999999991672 ) ;
#73953=CARTESIAN_POINT ( 'NONE',  ( 121.2641460698858396, 59.64250688777392639, -48.37286511902529895 ) ) ;
#73995=CARTESIAN_POINT ( 'NONE',  ( 119.4810000828223906, 74.54169681208188081, 52.62745965564226225 ) ) ;
#73997=EDGE_LOOP ( 'NONE', ( #58123, #35588, #3040, #17975 ) ) ;
#74004=EDGE_CURVE ( 'NONE', #6945, #35850, #56733, .T. ) ;
#74005=ORIENTED_EDGE ( 'NONE', *, *, #82547, .T. ) ;
#74013=CARTESIAN_POINT ( 'NONE',  ( 170.2205283966864897, 20.32000000000000028, -71.37400000000000944 ) ) ;
#74030=DIRECTION ( 'NONE',  ( 0.000000000000000000, -0.8660254037844387076, 0.4999999999999998890 ) ) ;
#74054=DIRECTION ( 'NONE',  ( 0.000000000000000000, 1.000000000000000000, 0.000000000000000000 ) ) ;
#74089=CARTESIAN_POINT ( 'NONE',  ( 141.3509999999999991, 101.5999999999999943, 141.3509999999999991 ) ) ;
#74107=CARTESIAN_POINT ( 'NONE',  ( -185.9961463128564958, 20.32000000000000028, -3.174999999999514877 ) ) ;
#74115=CARTESIAN_POINT ( 'NONE',  ( 33.98325472291465132, 8.255000000000000782, -3.174999999999999822 ) ) ;
#74116=B_SPLINE_CURVE_WITH_KNOTS ( 'NONE', 3,
 ( #13377, #82435, #66987, #12483, #4769, #60608, #6554, #26109, #53779, #20196, #40164, #67884, #28326, #49664 ),
 .UNSPECIFIED., .F., .F.,
 ( 4, 2, 2, 2, 2, 2, 4 ),
 ( 0.008390848235266742949, 0.01104543637615772525, 0.01237273044660322160, 0.01370002451704871449, 0.01635461265793970720, 0.01768190672838519661, 0.01900920079883068256 ),
 .UNSPECIFIED. ) ;
#74146=CARTESIAN_POINT ( 'NONE',  ( 9.685063450406051544, 90.77563096578916202, 130.1966975709476628 ) ) ;
#74154=CARTESIAN_POINT ( 'NONE',  ( 0.000000000000000000, 20.32000000000000028, 0.000000000000000000 ) ) ;
#74203=FACE_OUTER_BOUND ( 'NONE', #43650, .T. ) ;
#74205=ORIENTED_EDGE ( 'NONE', *, *, #36461, .F. ) ;
#74255=AXIS2_PLACEMENT_3D ( 'NONE', #402, #7226, #69450 ) ;
#74288=CYLINDRICAL_SURFACE ( 'NONE', #47327, 130.5560000000000116 ) ;
#74296=CARTESIAN_POINT ( 'NONE',  ( 1.154229608196380665E-15, 1.270000000000000018, 9.425000000000000711 ) ) ;
#74299=CARTESIAN_POINT ( 'NONE',  ( 0.000000000000000000, 12.27000000000000313, 0.000000000000000000 ) ) ;
#74303=VERTEX_POINT ( 'NONE', #61693 ) ;
#74305=AXIS2_PLACEMENT_3D ( 'NONE', #44782, #52024, #3014 ) ;
#74311=ORIENTED_EDGE ( 'NONE', *, *, #69162, .T. ) ;
#74326=FACE_OUTER_BOUND ( 'NONE', #58447, .T. ) ;
#74347=DIRECTION ( 'NONE',  ( 1.000000000000000000, 0.000000000000000000, 2.671820169801660301E-13 ) ) ;
#74358=CARTESIAN_POINT ( 'NONE',  ( 4.665904304751416087E-15, 95.00619999999999266, -38.10000000000000142 ) ) ;
#74406=ORIENTED_EDGE ( 'NONE', *, *, #76995, .F. ) ;
#74411=EDGE_CURVE ( 'NONE', #4573, #79978, #7543, .T. ) ;
#74422=EDGE_CURVE ( 'NONE', #64746, #65669, #5414, .T. ) ;
#74436=DIRECTION ( 'NONE',  ( 0.000000000000000000, 1.000000000000000000, 0.000000000000000000 ) ) ;
#74455=ORIENTED_EDGE ( 'NONE', *, *, #42203, .T. ) ;
#74456=DIRECTION ( 'NONE',  ( 0.000000000000000000, 0.000000000000000000, -1.000000000000000000 ) ) ;
#74509=EDGE_CURVE ( 'NONE', #67629, #23399, #6119, .T. ) ;
#74536=ORIENTED_EDGE ( 'NONE', *, *, #5053, .F. ) ;
#74553=DIRECTION ( 'NONE',  ( 0.000000000000000000, -1.000000000000000000, 0.000000000000000000 ) ) ;
#74559=DIRECTION ( 'NONE',  ( 0.000000000000000000, 0.000000000000000000, -1.000000000000000000 ) ) ;
#74576=CARTESIAN_POINT ( 'NONE',  ( 127.5252020268926003, 0.000000000000000000, 177.0380000000000109 ) ) ;
#74587=CARTESIAN_POINT ( 'NONE',  ( 10.55034476490975770, 89.61967029530742934, 130.1290104682496462 ) ) ;
#74644=EDGE_LOOP ( 'NONE', ( #34900, #19889, #32932, #13659 ) ) ;
#74645=AXIS2_PLACEMENT_3D ( 'NONE', #52690, #18208, #38648 ) ;
#74647=DIRECTION ( 'NONE',  ( -1.000000000000000000, 0.000000000000000000, 1.047445008332813989E-14 ) ) ;
#74666=ORIENTED_EDGE ( 'NONE', *, *, #68415, .F. ) ;
#74669=CARTESIAN_POINT ( 'NONE',  ( -22.56126763944003244, 58.71304942578738917, 30.70258120403678248 ) ) ;
#74681=CARTESIAN_POINT ( 'NONE',  ( 0.000000000000000000, 17.78000000000000114, -154.1697486074984909 ) ) ;
#74703=LINE ( 'NONE', #61505, #12662 ) ;
#74707=EDGE_CURVE ( 'NONE', #73595, #55433, #3070, .T. ) ;
#74730=ORIENTED_EDGE ( 'NONE', *, *, #43477, .F. ) ;
#74766=LINE ( 'NONE', #13440, #50905 ) ;
#74769=VERTEX_POINT ( 'NONE', #10328 ) ;
#74803=CARTESIAN_POINT ( 'NONE',  ( 33.98325472291465132, 8.255000000000000782, 3.174999999999999822 ) ) ;
#74814=ORIENTED_EDGE ( 'NONE', *, *, #6531, .F. ) ;
#74824=VERTEX_POINT ( 'NONE', #73888 ) ;
#74883=CIRCLE ( 'NONE', #9651, 9.524999999999998579 ) ;
#74903=ORIENTED_EDGE ( 'NONE', *, *, #75245, .T. ) ;
#74907=DIRECTION ( 'NONE',  ( 0.000000000000000000, 1.000000000000000000, 0.000000000000000000 ) ) ;
#74913=ORIENTED_EDGE ( 'NONE', *, *, #76995, .T. ) ;
#74917=AXIS2_PLACEMENT_3D ( 'NONE', #3676, #65013, #31370 ) ;
#74918=EDGE_CURVE ( 'NONE', #17548, #72419, #19824, .T. ) ;
#74955=ORIENTED_EDGE ( 'NONE', *, *, #54848, .T. ) ;
#74965=CARTESIAN_POINT ( 'NONE',  ( 10.20674285154820460, 74.98125221267765994, 130.1568226710593592 ) ) ;
#75006=ORIENTED_EDGE ( 'NONE', *, *, #61025, .F. ) ;
#75041=CARTESIAN_POINT ( 'NONE',  ( 11.59753438770549039, 87.72719248967439398, 130.0398859535097245 ) ) ;
#75052=VECTOR ( 'NONE', #64675, 1000.000000000000000 ) ;
#75065=LINE ( 'NONE', #66446, #26997 ) ;
#75078=EDGE_CURVE ( 'NONE', #43367, #57559, #55425, .T. ) ;
#75107=AXIS2_PLACEMENT_3D ( 'NONE', #68739, #50869, #37250 ) ;
#75118=CARTESIAN_POINT ( 'NONE',  ( -23.22008070988836792, 55.36727740576814938, 30.20659996360767252 ) ) ;
#75157=FACE_OUTER_BOUND ( 'NONE', #3011, .T. ) ;
#75178=ORIENTED_EDGE ( 'NONE', *, *, #31166, .F. ) ;
#75186=CARTESIAN_POINT ( 'NONE',  ( 0.000000000000000000, 8.255000000000000782, 0.000000000000000000 ) ) ;
#75188=EDGE_CURVE ( 'NONE', #60315, #81504, #56863, .T. ) ;
#75203=CARTESIAN_POINT ( 'NONE',  ( -121.5826742282154385, 74.35825521121780923, 47.56630412473074188 ) ) ;
#75206=EDGE_CURVE ( 'NONE', #47018, #27791, #62936, .T. ) ;
#75209=ORIENTED_EDGE ( 'NONE', *, *, #191, .F. ) ;
#75212=EDGE_CURVE ( 'NONE', #83920, #76533, #3265, .T. ) ;
#75227=DIRECTION ( 'NONE',  ( 0.000000000000000000, -1.000000000000000000, 0.000000000000000000 ) ) ;
#75234=CARTESIAN_POINT ( 'NONE',  ( -8.597104536545209896, 73.19917002513419391, 130.2727017199365775 ) ) ;
#75236=CARTESIAN_POINT ( 'NONE',  ( 0.000000000000000000, 20.32000000000000028, 0.000000000000000000 ) ) ;
#75245=EDGE_CURVE ( 'NONE', #78242, #28246, #4300, .T. ) ;
#75308=VECTOR ( 'NONE', #48738, 1000.000000000000000 ) ;
#75319=EDGE_CURVE ( 'NONE', #4943, #64884, #52403, .T. ) ;
#75353=EDGE_CURVE ( 'NONE', #3666, #47532, #40977, .T. ) ;
#75354=VECTOR ( 'NONE', #48182, 1000.000000000000000 ) ;
#75381=ORIENTED_EDGE ( 'NONE', *, *, #34304, .F. ) ;
#75400=CIRCLE ( 'NONE', #79762, 218.1859999999999786 ) ;
#75409=DIRECTION ( 'NONE',  ( 0.000000000000000000, -1.000000000000000000, 0.000000000000000000 ) ) ;
#75421=CARTESIAN_POINT ( 'NONE',  ( 7.208983637501106934, 72.09427944926730447, 130.3568028842946092 ) ) ;
#75427=CARTESIAN_POINT ( 'NONE',  ( 120.3165253744671759, 47.81691361759333603, -50.68368231966687887 ) ) ;
#75428=EDGE_LOOP ( 'NONE', ( #40126, #77003, #22475, #52655 ) ) ;
#75431=ADVANCED_FACE ( 'NONE', ( #81069 ), #19709, .F. ) ;
#75434=EDGE_CURVE ( 'NONE', #85626, #29697, #54048, .T. ) ;
#75439=FACE_OUTER_BOUND ( 'NONE', #27511, .T. ) ;
#75444=EDGE_CURVE ( 'NONE', #80913, #32309, #18817, .T. ) ;
#75484=ORIENTED_EDGE ( 'NONE', *, *, #34458, .F. ) ;
#75514=VECTOR ( 'NONE', #16771, 1000.000000000000000 ) ;
#75521=DIRECTION ( 'NONE',  ( -1.825781832977094422E-16, 0.4999999999999998890, 0.8660254037844387076 ) ) ;
#75548=FACE_OUTER_BOUND ( 'NONE', #37551, .T. ) ;
#75551=CIRCLE ( 'NONE', #88656, 9.525000000000000355 ) ;
#75565=CARTESIAN_POINT ( 'NONE',  ( -141.3509999999999991, 0.000000000000000000, 132.7150000000000034 ) ) ;
#75588=DIRECTION ( 'NONE',  ( 0.000000000000000000, 0.000000000000000000, 1.000000000000000000 ) ) ;
#75601=PLANE ( 'NONE',  #33490 ) ;
#75605=ORIENTED_EDGE ( 'NONE', *, *, #56651, .T. ) ;
#75608=CARTESIAN_POINT ( 'NONE',  ( -71.09939861440099662, 0.000000000000000000, 177.8662485265279827 ) ) ;
#75634=VERTEX_POINT ( 'NONE', #41925 ) ;
#75640=FACE_OUTER_BOUND ( 'NONE', #18790, .T. ) ;
#75652=ADVANCED_FACE ( 'NONE', ( #35117 ), #55094, .T. ) ;
#75654=VERTEX_POINT ( 'NONE', #76467 ) ;
#75657=CARTESIAN_POINT ( 'NONE',  ( -115.3679503581490309, 71.85924980799624961, 61.11881860259094879 ) ) ;
#75682=CARTESIAN_POINT ( 'NONE',  ( -10.07588608733909119, 74.81633509576083441, 130.1668266806610177 ) ) ;
#75686=DIRECTION ( 'NONE',  ( 0.000000000000000000, 1.000000000000000000, 0.000000000000000000 ) ) ;
#75705=CARTESIAN_POINT ( 'NONE',  ( -186.2398777604659870, 0.000000000000000000, 107.9500000000000028 ) ) ;
#75731=ADVANCED_FACE ( 'NONE', ( #36027 ), #30877, .F. ) ;
#75766=EDGE_CURVE ( 'NONE', #38579, #15522, #64627, .T. ) ;
#75829=AXIS2_PLACEMENT_3D ( 'NONE', #24766, #52436, #4330 ) ;
#75849=CYLINDRICAL_SURFACE ( 'NONE', #60928, 7.873999999999991672 ) ;
#75861=CARTESIAN_POINT ( 'NONE',  ( 7.161806819047721540, 72.06186804431776238, 130.3594151003946138 ) ) ;
#75870=CARTESIAN_POINT ( 'NONE',  ( 123.4442068678753799, 45.02545161509468130, -42.50497980019686395 ) ) ;
#75889=ORIENTED_EDGE ( 'NONE', *, *, #19350, .T. ) ;
#75904=ORIENTED_EDGE ( 'NONE', *, *, #1538, .T. ) ;
#75961=LINE ( 'NONE', #27801, #15950 ) ;
#76030=CARTESIAN_POINT ( 'NONE',  ( 196.2150000000000034, 43.68799999999999528, 57.14999999999999858 ) ) ;
#76031=DIRECTION ( 'NONE',  ( 0.000000000000000000, 1.000000000000000000, 0.000000000000000000 ) ) ;
#76059=CARTESIAN_POINT ( 'NONE',  ( 3.110602869834275287E-15, -71.84204896855320044, -25.39999999999999858 ) ) ;
#76071=DIRECTION ( 'NONE',  ( 0.000000000000000000, 0.000000000000000000, -1.000000000000000000 ) ) ;
#76082=AXIS2_PLACEMENT_3D ( 'NONE', #26425, #5081, #88219 ) ;
#76089=ORIENTED_EDGE ( 'NONE', *, *, #33476, .F. ) ;
#76092=CARTESIAN_POINT ( 'NONE',  ( -123.5099984066448684, 72.79992482915794483, 42.31500800594746181 ) ) ;
#76116=CARTESIAN_POINT ( 'NONE',  ( -7.038238517017752827, 71.97865724765921414, 130.3661473682803376 ) ) ;
#76142=EDGE_LOOP ( 'NONE', ( #13952, #58232, #77553, #67255 ) ) ;
#76160=DIRECTION ( 'NONE',  ( 0.000000000000000000, 0.000000000000000000, 1.000000000000000000 ) ) ;
#76164=ORIENTED_EDGE ( 'NONE', *, *, #3636, .T. ) ;
#76172=CARTESIAN_POINT ( 'NONE',  ( -135.2444258376732193, 0.000000000000000000, -147.4575741623275746 ) ) ;
#76174=CARTESIAN_POINT ( 'NONE',  ( 208.9149999999999920, 30.98800000000000310, 57.14999999999999858 ) ) ;
#76197=LINE ( 'NONE', #83041, #29978 ) ;
#76199=ORIENTED_EDGE ( 'NONE', *, *, #56454, .F. ) ;
#76212=DIRECTION ( 'NONE',  ( 0.000000000000000000, 0.000000000000000000, 1.000000000000000000 ) ) ;
#76225=DIRECTION ( 'NONE',  ( 0.000000000000000000, 1.000000000000000000, 0.000000000000000000 ) ) ;
#76232=CARTESIAN_POINT ( 'NONE',  ( 109.2774118001976120, 53.97500000000000142, 71.43750000000000000 ) ) ;
#76249=DIRECTION ( 'NONE',  ( 0.7071067811865590080, 0.000000000000000000, 0.7071067811865361374 ) ) ;
#76255=ORIENTED_EDGE ( 'NONE', *, *, #34196, .T. ) ;
#76259=DIRECTION ( 'NONE',  ( 0.3552177606235679130, 0.000000000000000000, -0.9347835805883507598 ) ) ;
#76296=CARTESIAN_POINT ( 'NONE',  ( -126.4481529151155996, 44.45000000000000284, 32.49205688096009936 ) ) ;
#76307=CARTESIAN_POINT ( 'NONE',  ( 4.872201249568272274, 70.82175023847671014, 130.4650562613408908 ) ) ;
#76314=CARTESIAN_POINT ( 'NONE',  ( 123.9297970803746267, 45.55335027554141192, -41.06498388075110739 ) ) ;
#76361=( NAMED_UNIT ( * ) PLANE_ANGLE_UNIT ( ) SI_UNIT ( $, .RADIAN. ) );
#76382=ORIENTED_EDGE ( 'NONE', *, *, #54848, .F. ) ;
#76388=EDGE_CURVE ( 'NONE', #51056, #84701, #61677, .T. ) ;
#76405=CARTESIAN_POINT ( 'NONE',  ( 0.000000000000000000, -71.84204896855320044, 0.000000000000000000 ) ) ;
#76410=ORIENTED_EDGE ( 'NONE', *, *, #78014, .T. ) ;
#76413=DIRECTION ( 'NONE',  ( 0.000000000000000000, -1.000000000000000000, 0.000000000000000000 ) ) ;
#76450=CARTESIAN_POINT ( 'NONE',  ( -187.8075999999999794, 20.32000000000000028, -9.525000000000000355 ) ) ;
#76467=CARTESIAN_POINT ( 'NONE',  ( -186.2398777604655038, 0.000000000000000000, -6.349999999999999645 ) ) ;
#76475=ORIENTED_EDGE ( 'NONE', *, *, #70431, .F. ) ;
#76514=CARTESIAN_POINT ( 'NONE',  ( 163.0822201311030142, 101.5999999999999943, 75.92468371870748456 ) ) ;
#76515=DIRECTION ( 'NONE',  ( 0.000000000000000000, 1.000000000000000000, 0.000000000000000000 ) ) ;
#76533=VERTEX_POINT ( 'NONE', #41229 ) ;
#76534=VECTOR ( 'NONE', #65239, 1000.000000000000000 ) ;
#76546=CARTESIAN_POINT ( 'NONE',  ( -123.2955287385074143, 73.06768973456320282, 42.93641881194006515 ) ) ;
#76549=CIRCLE ( 'NONE', #28698, 34.13125000000000142 ) ;
#76573=ADVANCED_FACE ( 'NONE', ( #70757 ), #56194, .F. ) ;
#76576=CARTESIAN_POINT ( 'NONE',  ( -10.55536724279236616, 75.48783127733061349, 130.1286031690422078 ) ) ;
#76591=ORIENTED_EDGE ( 'NONE', *, *, #28357, .T. ) ;
#76600=DIRECTION ( 'NONE',  ( 0.000000000000000000, 0.000000000000000000, 1.000000000000000000 ) ) ;
#76607=VERTEX_POINT ( 'NONE', #68960 ) ;
#76627=DIRECTION ( 'NONE',  ( 1.825781832977096147E-16, 0.5000000000000003331, -0.8660254037844384856 ) ) ;
#76628=DIRECTION ( 'NONE',  ( 1.000000000000000000, 0.000000000000000000, 2.671820169801660301E-13 ) ) ;
#76629=CIRCLE ( 'NONE', #12827, 8.636000000000004562 ) ;
#76638=EDGE_CURVE ( 'NONE', #38934, #7104, #57554, .T. ) ;
#76654=ORIENTED_EDGE ( 'NONE', *, *, #67021, .T. ) ;
#76655=VECTOR ( 'NONE', #16271, 1000.000000000000000 ) ;
#76692=CARTESIAN_POINT ( 'NONE',  ( 109.2774118001976120, 53.97500000000000142, 71.43750000000000000 ) ) ;
#76705=DIRECTION ( 'NONE',  ( 0.000000000000000000, 0.000000000000000000, -1.000000000000000000 ) ) ;
#76728=VECTOR ( 'NONE', #89165, 1000.000000000000000 ) ;
#76731=AXIS2_PLACEMENT_3D ( 'NONE', #71503, #23361, #10588 ) ;
#76739=CARTESIAN_POINT ( 'NONE',  ( -215.9000000000000057, 101.5999999999999943, 146.9389999999999930 ) ) ;
#76747=ORIENTED_EDGE ( 'NONE', *, *, #26265, .F. ) ;
#76749=ORIENTED_EDGE ( 'NONE', *, *, #27585, .T. ) ;
#76755=DIRECTION ( 'NONE',  ( 0.000000000000000000, 0.000000000000000000, 1.000000000000000000 ) ) ;
#76756=CARTESIAN_POINT ( 'NONE',  ( 7.108806956920044051, 72.02595942673482909, 130.3623174704088115 ) ) ;
#76764=CARTESIAN_POINT ( 'NONE',  ( 124.1536575006588379, 45.91621576730522492, -40.38304405550843512 ) ) ;
#76779=FACE_OUTER_BOUND ( 'NONE', #15664, .T. ) ;
#76785=AXIS2_PLACEMENT_3D ( 'NONE', #21807, #447, #76755 ) ;
#76811=LINE ( 'NONE', #6423, #75354 ) ;
#76845=CIRCLE ( 'NONE', #49270, 7.937500000000000000 ) ;
#76863=ADVANCED_FACE ( 'NONE', ( #67054 ), #24830, .F. ) ;
#76888=EDGE_LOOP ( 'NONE', ( #70469, #77005, #35137, #33232, #41891, #40069, #27770, #47376, #21690, #62771, #79777, #65005, #77747, #48030, #87695, #49012 ) ) ;
#76942=CIRCLE ( 'NONE', #58067, 130.5560000000000116 ) ;
#76945=EDGE_LOOP ( 'NONE', ( #59431, #55143, #48834, #88886 ) ) ;
#76961=DIRECTION ( 'NONE',  ( 0.000000000000000000, 1.000000000000000000, 0.000000000000000000 ) ) ;
#76982=VECTOR ( 'NONE', #46379, 1000.000000000000000 ) ;
#76995=EDGE_CURVE ( 'NONE', #15725, #89539, #40971, .T. ) ;
#77001=CARTESIAN_POINT ( 'NONE',  ( -116.2551261185419236, 72.73974665673414108, 59.41428421001764093 ) ) ;
#77003=ORIENTED_EDGE ( 'NONE', *, *, #32415, .T. ) ;
#77005=ORIENTED_EDGE ( 'NONE', *, *, #8690, .T. ) ;
#77031=CARTESIAN_POINT ( 'NONE',  ( 0.000000000000000000, 101.5999999999999943, 0.000000000000000000 ) ) ;
#77037=DIRECTION ( 'NONE',  ( 0.000000000000000000, 0.000000000000000000, -1.000000000000000000 ) ) ;
#77056=CIRCLE ( 'NONE', #39296, 9.425000000000000711 ) ;
#77066=VECTOR ( 'NONE', #79386, 1000.000000000000114 ) ;
#77109=AXIS2_PLACEMENT_3D ( 'NONE', #723, #27982, #49312 ) ;
#77120=CARTESIAN_POINT ( 'NONE',  ( -109.7273655885044974, 48.66981474652848050, 70.74444168010853673 ) ) ;
#77249=CARTESIAN_POINT ( 'NONE',  ( 125.8424616898026756, 66.98845471270220742, 34.76731936747097507 ) ) ;
#77253=ORIENTED_EDGE ( 'NONE', *, *, #56454, .T. ) ;
#77260=LINE ( 'NONE', #29109, #4096 ) ;
#77284=ORIENTED_EDGE ( 'NONE', *, *, #61910, .T. ) ;
#77302=CARTESIAN_POINT ( 'NONE',  ( -71.09939861440099662, 0.000000000000000000, 177.8662485265279827 ) ) ;
#77359=CARTESIAN_POINT ( 'NONE',  ( 12.03847361652802306, 78.49881328697941285, 129.9999214341232232 ) ) ;
#77400=ORIENTED_EDGE ( 'NONE', *, *, #51084, .F. ) ;
#77401=ORIENTED_EDGE ( 'NONE', *, *, #58581, .F. ) ;
#77414=EDGE_CURVE ( 'NONE', #12239, #83014, #69638, .T. ) ;
#77438=CARTESIAN_POINT ( 'NONE',  ( 0.000000000000000000, -71.84204896855320044, 25.39999999999999858 ) ) ;
#77448=VECTOR ( 'NONE', #71698, 1000.000000000000000 ) ;
#77460=EDGE_LOOP ( 'NONE', ( #4549, #70864, #28148, #50151 ) ) ;
#77470=CARTESIAN_POINT ( 'NONE',  ( -187.8075999999999794, 101.5999999999999943, 114.2999999999999972 ) ) ;
#77490=DIRECTION ( 'NONE',  ( -0.000000000000000000, 1.000000000000000000, 0.000000000000000000 ) ) ;
#77506=VERTEX_POINT ( 'NONE', #21951 ) ;
#77534=ADVANCED_FACE ( 'NONE', ( #31314, #59009, #79945 ), #86748, .T. ) ;
#77542=ORIENTED_EDGE ( 'NONE', *, *, #3393, .T. ) ;
#77553=ORIENTED_EDGE ( 'NONE', *, *, #17531, .T. ) ;
#77555=VERTEX_POINT ( 'NONE', #45819 ) ;
#77559=CARTESIAN_POINT ( 'NONE',  ( -109.9591342944440697, 47.45097955103868514, 70.38379434518259359 ) ) ;
#77572=DIRECTION ( 'NONE',  ( -0.7071067811865470176, 0.000000000000000000, -0.7071067811865480168 ) ) ;
#77574=CARTESIAN_POINT ( 'NONE',  ( 1.385076594094139635, 70.24203434096087051, 38.10000000000000142 ) ) ;
#77589=CARTESIAN_POINT ( 'NONE',  ( -11.41071036765134750, 68.71936554549954224, 36.35710361961175607 ) ) ;
#77591=EDGE_LOOP ( 'NONE', ( #1080, #18252, #21691, #5181 ) ) ;
#77646=VECTOR ( 'NONE', #58, 1000.000000000000000 ) ;
#77648=CARTESIAN_POINT ( 'NONE',  ( 0.000000000000000000, 95.00619999999999266, 0.000000000000000000 ) ) ;
#77680=EDGE_LOOP ( 'NONE', ( #71052, #80739, #89502, #61749 ) ) ;
#77683=ORIENTED_EDGE ( 'NONE', *, *, #89055, .F. ) ;
#77691=DIRECTION ( 'NONE',  ( -1.000000000000000000, 0.000000000000000000, -2.108231265501709878E-16 ) ) ;
#77696=CARTESIAN_POINT ( 'NONE',  ( 126.9809554502671887, 56.79209779858037876, 30.34323007394005600 ) ) ;
#77712=VERTEX_POINT ( 'NONE', #33993 ) ;
#77724=CONICAL_SURFACE ( 'NONE', #28350, 161.5439999999999827, 0.08726646259971625186 ) ;
#77732=CARTESIAN_POINT ( 'NONE',  ( 127.5252020268926003, 101.5999999999999943, 177.0380000000000109 ) ) ;
#77741=CARTESIAN_POINT ( 'NONE',  ( 50.03799999999999670, 0.000000000000000000, 191.3008000794699797 ) ) ;
#77747=ORIENTED_EDGE ( 'NONE', *, *, #34405, .T. ) ;
#77757=CARTESIAN_POINT ( 'NONE',  ( 170.2205283966864897, 20.32000000000000028, 71.37400000000000944 ) ) ;
#77773=VECTOR ( 'NONE', #87300, 1000.000000000000000 ) ;
#77808=PLANE ( 'NONE',  #63758 ) ;
#77813=PRODUCT_DEFINITION_CONTEXT ( 'detailed design', #30700, 'design' ) ;
#77824=CYLINDRICAL_SURFACE ( 'NONE', #5121, 179.8898777604655095 ) ;
#77839=AXIS2_PLACEMENT_3D ( 'NONE', #87742, #5984, #12336 ) ;
#77858=EDGE_LOOP ( 'NONE', ( #27661, #71340, #87634, #42511 ) ) ;
#77869=CARTESIAN_POINT ( 'NONE',  ( -215.9000000000000057, 0.000000000000000000, -45.33899999999999864 ) ) ;
#77889=ORIENTED_EDGE ( 'NONE', *, *, #65217, .T. ) ;
#77959=ORIENTED_EDGE ( 'NONE', *, *, #21042, .T. ) ;
#77997=ORIENTED_EDGE ( 'NONE', *, *, #65167, .T. ) ;
#78002=EDGE_CURVE ( 'NONE', #46484, #87166, #10331, .T. ) ;
#78014=EDGE_CURVE ( 'NONE', #64725, #4573, #86640, .T. ) ;
#78068=VECTOR ( 'NONE', #38953, 1000.000000000000000 ) ;
#78077=LINE ( 'NONE', #15838, #18101 ) ;
#78078=DIRECTION ( 'NONE',  ( -7.980413499659419871E-32, -1.000000000000000000, 3.785359618865284342E-16 ) ) ;
#78085=DIRECTION ( 'NONE',  ( 0.000000000000000000, 0.000000000000000000, -1.000000000000000000 ) ) ;
#78102=FACE_OUTER_BOUND ( 'NONE', #41104, .T. ) ;
#78114=VECTOR ( 'NONE', #20213, 1000.000000000000000 ) ;
#78118=CARTESIAN_POINT ( 'NONE',  ( -21.75527563292445521, 47.22364764115523172, 31.28221943681005257 ) ) ;
#78125=EDGE_CURVE ( 'NONE', #19557, #27791, #73010, .T. ) ;
#78147=CARTESIAN_POINT ( 'NONE',  ( 109.2774118001976120, 53.97500000000000142, 71.43750000000000000 ) ) ;
#78160=CARTESIAN_POINT ( 'NONE',  ( 125.5854509285793910, 68.02811073279640652, 35.68229276901666225 ) ) ;
#78242=VERTEX_POINT ( 'NONE', #48392 ) ;
#78305=CARTESIAN_POINT ( 'NONE',  ( 6.719641267068065638, 93.32766509845849612, 130.3830046867565500 ) ) ;
#78328=CARTESIAN_POINT ( 'NONE',  ( 0.000000000000000000, 0.000000000000000000, 0.000000000000000000 ) ) ;
#78334=VERTEX_POINT ( 'NONE', #20286 ) ;
#78348=ORIENTED_EDGE ( 'NONE', *, *, #65582, .T. ) ;
#78362=ORIENTED_EDGE ( 'NONE', *, *, #14863, .F. ) ;
#78367=ORIENTED_EDGE ( 'NONE', *, *, #86918, .F. ) ;
#78387=EDGE_CURVE ( 'NONE', #82724, #36938, #23745, .T. ) ;
#78390=CARTESIAN_POINT ( 'NONE',  ( 183.5150000000000148, 21.46300000000000097, 41.63456447661474868 ) ) ;
#78394=CARTESIAN_POINT ( 'NONE',  ( 131.3179999999999836, 53.97500000000000142, 30.16249999999999787 ) ) ;
#78401=ORIENTED_EDGE ( 'NONE', *, *, #83461, .T. ) ;
#78440=CARTESIAN_POINT ( 'NONE',  ( 31.75000000000000000, 17.78000000000000114, -3.174999999999999822 ) ) ;
#78441=CARTESIAN_POINT ( 'NONE',  ( -10.77377455544796625, 89.27589758714826473, 130.1107393577912035 ) ) ;
#78455=CARTESIAN_POINT ( 'NONE',  ( -50.03799999999999670, 101.5999999999999943, 206.3750000000000000 ) ) ;
#78475=CARTESIAN_POINT ( 'NONE',  ( -109.7874373783072457, 48.32589523802096210, 70.65122087376927595 ) ) ;
#78481=VECTOR ( 'NONE', #64427, 1000.000000000000000 ) ;
#78482=ORIENTED_EDGE ( 'NONE', *, *, #62799, .F. ) ;
#78512=DIRECTION ( 'NONE',  ( -1.000000000000000000, 0.000000000000000000, 0.000000000000000000 ) ) ;
#78518=ORIENTED_EDGE ( 'NONE', *, *, #63926, .T. ) ;
#78542=CARTESIAN_POINT ( 'NONE',  ( -19.89663890320305839, 44.45000000000000284, 32.49205688096009936 ) ) ;
#78553=VECTOR ( 'NONE', #64311, 1000.000000000000000 ) ;
#78560=EDGE_CURVE ( 'NONE', #89089, #62710, #72888, .T. ) ;
#78568=ADVANCED_FACE ( 'NONE', ( #15709 ), #43384, .F. ) ;
#78569=DIRECTION ( 'NONE',  ( 1.000000000000000000, 0.000000000000000000, -3.491483361109380094E-15 ) ) ;
#78582=ORIENTED_EDGE ( 'NONE', *, *, #29520, .T. ) ;
#78622=AXIS2_PLACEMENT_3D ( 'NONE', #8337, #83300, #50095 ) ;
#78645=ADVANCED_FACE ( 'NONE', ( #4301 ), #88327, .F. ) ;
#78648=CARTESIAN_POINT ( 'NONE',  ( 208.9149999999999920, 37.33800000000000097, 41.27499999999999858 ) ) ;
#78658=LINE ( 'NONE', #2785, #57318 ) ;
#78661=AXIS2_PLACEMENT_3D ( 'NONE', #31326, #86760, #69444 ) ;
#78682=DIRECTION ( 'NONE',  ( 0.000000000000000000, 0.000000000000000000, 1.000000000000000000 ) ) ;
#78684=ADVANCED_FACE ( 'NONE', ( #17917 ), #73328, .F. ) ;
#78708=CARTESIAN_POINT ( 'NONE',  ( -33.98325472291460159, 17.78000000000000114, 3.175000000000234746 ) ) ;
#78743=CARTESIAN_POINT ( 'NONE',  ( 55.48342271751659638, 101.5999999999999943, 171.1197181046785261 ) ) ;
#78753=CARTESIAN_POINT ( 'NONE',  ( 3.944304526105059924E-28, 95.25000000000000000, 130.5560000000000116 ) ) ;
#78762=DIRECTION ( 'NONE',  ( -0.000000000000000000, 1.000000000000000000, 0.000000000000000000 ) ) ;
#78819=DIRECTION ( 'NONE',  ( 0.000000000000000000, 0.000000000000000000, 1.000000000000000000 ) ) ;
#78876=DIRECTION ( 'NONE',  ( 0.000000000000000000, 0.000000000000000000, -1.000000000000000000 ) ) ;
#78882=CARTESIAN_POINT ( 'NONE',  ( -6.301391689584750821, 93.58422381887211827, 130.4043053684175106 ) ) ;
#78885=LINE ( 'NONE', #66565, #28681 ) ;
#78953=ORIENTED_EDGE ( 'NONE', *, *, #28288, .F. ) ;
#78993=CYLINDRICAL_SURFACE ( 'NONE', #42113, 9.525000000000000355 ) ;
#79018=DIRECTION ( 'NONE',  ( 0.000000000000000000, 0.000000000000000000, -1.000000000000000000 ) ) ;
#79043=CARTESIAN_POINT ( 'NONE',  ( 111.3497592566078964, 65.14957505911826274, 68.16382463248645251 ) ) ;
#79073=CARTESIAN_POINT ( 'NONE',  ( 0.000000000000000000, 0.000000000000000000, -161.5439999999999827 ) ) ;
#79195=CARTESIAN_POINT ( 'NONE',  ( 4.684674336965106711, 94.35461990771972296, 130.4719347088314123 ) ) ;
#79203=LINE ( 'NONE', #30142, #20156 ) ;
#79207=ORIENTED_EDGE ( 'NONE', *, *, #61811, .T. ) ;
#79224=FACE_OUTER_BOUND ( 'NONE', #255, .T. ) ;
#79243=ADVANCED_FACE ( 'NONE', ( #9126 ), #15941, .T. ) ;
#79260=CARTESIAN_POINT ( 'NONE',  ( 0.000000000000000000, 82.54999999999999716, -179.8908777604655143 ) ) ;
#79318=EDGE_CURVE ( 'NONE', #45792, #34396, #54295, .T. ) ;
#79326=CARTESIAN_POINT ( 'NONE',  ( -7.206242203287891002, 93.00761057503720508, 130.3569541155684988 ) ) ;
#79333=DIRECTION ( 'NONE',  ( -0.000000000000000000, 1.000000000000000000, 0.000000000000000000 ) ) ;
#79336=VECTOR ( 'NONE', #26030, 1000.000000000000000 ) ;
#79360=EDGE_CURVE ( 'NONE', #21659, #51663, #42706, .T. ) ;
#79370=ORIENTED_EDGE ( 'NONE', *, *, #75434, .F. ) ;
#79386=DIRECTION ( 'NONE',  ( 0.9347835805883503157, 0.000000000000000000, -0.3552177606235690788 ) ) ;
#79402=PLANE ( 'NONE',  #51775 ) ;
#79458=CARTESIAN_POINT ( 'NONE',  ( 31.75000000000000000, 24.56180297284579694, -3.174999999999999822 ) ) ;
#79466=ORIENTED_EDGE ( 'NONE', *, *, #37990, .T. ) ;
#79494=CARTESIAN_POINT ( 'NONE',  ( 119.7619606472514135, 74.58858857478185200, 51.98495555578256955 ) ) ;
#79498=ORIENTED_EDGE ( 'NONE', *, *, #32243, .F. ) ;
#79509=CIRCLE ( 'NONE', #53320, 7.874000000000186184 ) ;
#79520=CARTESIAN_POINT ( 'NONE',  ( -160.2664750769294812, 0.000000000000000000, -148.0533267522755807 ) ) ;
#79521=CARTESIAN_POINT ( 'NONE',  ( -135.2444258376732193, 20.32000000000000028, -147.4575741623275746 ) ) ;
#79524=LINE ( 'NONE', #65430, #28270 ) ;
#79571=FACE_OUTER_BOUND ( 'NONE', #57688, .T. ) ;
#79600=AXIS2_PLACEMENT_3D ( 'NONE', #27905, #55583, #49684 ) ;
#79613=DIRECTION ( 'NONE',  ( -1.000000000000000000, 0.000000000000000000, 0.000000000000000000 ) ) ;
#79614=ADVANCED_FACE ( 'NONE', ( #49325 ), #26316, .F. ) ;
#79636=CARTESIAN_POINT ( 'NONE',  ( 4.851269734593515182, 94.28692116364298670, 130.4658362704004730 ) ) ;
#79650=EDGE_LOOP ( 'NONE', ( #8116, #74814, #48077, #74903 ) ) ;
#79696=CARTESIAN_POINT ( 'NONE',  ( 131.3179999999999836, 37.33800000000000097, 50.79999999999999716 ) ) ;
#79722=DIRECTION ( 'NONE',  ( 0.000000000000000000, 0.000000000000000000, 1.000000000000000000 ) ) ;
#79762=AXIS2_PLACEMENT_3D ( 'NONE', #78328, #2458, #30602 ) ;
#79775=CARTESIAN_POINT ( 'NONE',  ( -5.017381069699506924, 94.21703938470614048, 130.4595628991474143 ) ) ;
#79777=ORIENTED_EDGE ( 'NONE', *, *, #41869, .T. ) ;
#79866=ADVANCED_FACE ( 'NONE', ( #69673 ), #48299, .F. ) ;
#79888=LINE ( 'NONE', #43984, #24897 ) ;
#79893=VERTEX_POINT ( 'NONE', #7446 ) ;
#79895=CARTESIAN_POINT ( 'NONE',  ( 120.2489068914665182, 57.44811514648141326, -50.84382873326221386 ) ) ;
#79928=VERTEX_POINT ( 'NONE', #13370 ) ;
#79940=CARTESIAN_POINT ( 'NONE',  ( 110.1894008633096149, 61.51549208609898045, 70.02337478721381103 ) ) ;
#79945=FACE_BOUND ( 'NONE', #1984, .T. ) ;
#79978=VERTEX_POINT ( 'NONE', #69068 ) ;
#79983=CARTESIAN_POINT ( 'NONE',  ( -194.1576000000000022, 101.5999999999999943, 114.2999999999999972 ) ) ;
#80007=SURFACE_STYLE_USAGE ( .BOTH. , #85934 ) ;
#80012=ADVANCED_FACE ( 'NONE', ( #76779 ), #29083, .F. ) ;
#80028=DIRECTION ( 'NONE',  ( 0.000000000000000000, 1.000000000000000000, 0.000000000000000000 ) ) ;
#80061=EDGE_CURVE ( 'NONE', #51500, #80913, #55410, .T. ) ;
#80098=VECTOR ( 'NONE', #11301, 1000.000000000000114 ) ;
#80108=CARTESIAN_POINT ( 'NONE',  ( 208.9149999999999920, 43.68799999999999528, 44.45000000000000284 ) ) ;
#80130=CARTESIAN_POINT ( 'NONE',  ( 183.5150000000000148, 37.33800000000000097, 69.13087104677069306 ) ) ;
#80164=DIRECTION ( 'NONE',  ( -1.000000000000000000, 0.000000000000000000, -2.108231265501709878E-16 ) ) ;
#80198=EDGE_CURVE ( 'NONE', #13914, #51337, #52489, .T. ) ;
#80215=CARTESIAN_POINT ( 'NONE',  ( -4.887181091293991031, 94.27201341476896346, 130.4644959256346795 ) ) ;
#80237=CARTESIAN_POINT ( 'NONE',  ( -110.0726456481004050, 61.01229592318024686, 70.20625887764980178 ) ) ;
#80260=ORIENTED_EDGE ( 'NONE', *, *, #32946, .T. ) ;
#80272=CARTESIAN_POINT ( 'NONE',  ( 1.925672578516905147E-22, 69.84999999999999432, 130.5560000000000116 ) ) ;
#80328=VECTOR ( 'NONE', #49598, 1000.000000000000000 ) ;
#80334=CARTESIAN_POINT ( 'NONE',  ( 124.7264490944447175, 58.08405409534557151, -38.57737657011050914 ) ) ;
#80335=ORIENTED_EDGE ( 'NONE', *, *, #32889, .T. ) ;
#80352=ORIENTED_EDGE ( 'NONE', *, *, #67021, .F. ) ;
#80375=CARTESIAN_POINT ( 'NONE',  ( -185.9961463128564958, 20.32000000000000028, -9.525000000000000355 ) ) ;
#80381=CARTESIAN_POINT ( 'NONE',  ( 109.3721747360122691, 56.79532162893549696, 71.29316779583847108 ) ) ;
#80395=DIRECTION ( 'NONE',  ( 0.000000000000000000, 0.000000000000000000, -1.000000000000000000 ) ) ;
#80397=LINE ( 'NONE', #74013, #30783 ) ;
#80438=VECTOR ( 'NONE', #2945, 1000.000000000000000 ) ;
#80468=CYLINDRICAL_SURFACE ( 'NONE', #60645, 8.636000000000004562 ) ;
#80507=CARTESIAN_POINT ( 'NONE',  ( 173.9900000000000091, 20.32000000000000028, 71.37400000000000944 ) ) ;
#80534=VECTOR ( 'NONE', #23941, 1000.000000000000000 ) ;
#80551=PRODUCT_DEFINITION ( 'UNKNOWN', '', #34839, #77813 ) ;
#80558=AXIS2_PLACEMENT_3D ( 'NONE', #88, #26002, #60963 ) ;
#80564=ORIENTED_EDGE ( 'NONE', *, *, #43669, .F. ) ;
#80583=DIRECTION ( 'NONE',  ( 0.000000000000000000, -1.000000000000000000, 0.000000000000000000 ) ) ;
#80592=EDGE_CURVE ( 'NONE', #57125, #62710, #36798, .T. ) ;
#80595=CARTESIAN_POINT ( 'NONE',  ( -187.8075999999999794, 101.5999999999999943, 114.2999999999999972 ) ) ;
#80600=LINE ( 'NONE', #39246, #879 ) ;
#80606=CARTESIAN_POINT ( 'NONE',  ( -19.19064667470416197, 64.29050366814337281, 32.91834566403962015 ) ) ;
#80655=CIRCLE ( 'NONE', #51576, 218.1859999999999786 ) ;
#80657=DIRECTION ( 'NONE',  ( 0.000000000000000000, 0.000000000000000000, -1.000000000000000000 ) ) ;
#80682=CARTESIAN_POINT ( 'NONE',  ( -111.5220324117239556, 65.55856874647801646, 67.88008701381139076 ) ) ;
#80701=DIRECTION ( 'NONE',  ( -1.531877379624855416E-14, 0.000000000000000000, 1.000000000000000000 ) ) ;
#80708=CARTESIAN_POINT ( 'NONE',  ( -147.4575741623271767, 0.000000000000000000, -135.2444258376735888 ) ) ;
#80712=CARTESIAN_POINT ( 'NONE',  ( -1.594871763261194175, 69.92315485616694559, 130.5484598327008712 ) ) ;
#80736=EDGE_CURVE ( 'NONE', #85960, #44232, #4053, .T. ) ;
#80739=ORIENTED_EDGE ( 'NONE', *, *, #33616, .T. ) ;
#80755=CARTESIAN_POINT ( 'NONE',  ( 141.3509999999999991, 0.000000000000000000, 141.3509999999999991 ) ) ;
#80762=EDGE_CURVE ( 'NONE', #18491, #16965, #73535, .T. ) ;
#80767=ORIENTED_EDGE ( 'NONE', *, *, #81168, .T. ) ;
#80770=AXIS2_PLACEMENT_3D ( 'NONE', #3276, #53617, #25048 ) ;
#80782=CARTESIAN_POINT ( 'NONE',  ( 125.3303947399734568, 53.81125057877675744, -36.56738695590195931 ) ) ;
#80784=ORIENTED_EDGE ( 'NONE', *, *, #11675, .F. ) ;
#80794=AXIS2_PLACEMENT_3D ( 'NONE', #84195, #36023, #58681 ) ;
#80820=PLANE ( 'NONE',  #69223 ) ;
#80825=PLANE ( 'NONE',  #20216 ) ;
#80828=CARTESIAN_POINT ( 'NONE',  ( 0.000000000000000000, 20.32000000000000028, 0.000000000000000000 ) ) ;
#80830=CARTESIAN_POINT ( 'NONE',  ( 113.2217361175605532, 68.94557673950741616, 65.00547801876621179 ) ) ;
#80843=DIRECTION ( 'NONE',  ( -0.000000000000000000, -1.000000000000000000, -0.000000000000000000 ) ) ;
#80863=CARTESIAN_POINT ( 'NONE',  ( 183.5150000000000148, 53.21300000000000097, 59.96543552338529537 ) ) ;
#80865=EDGE_CURVE ( 'NONE', #61274, #47365, #64938, .T. ) ;
#80882=ORIENTED_EDGE ( 'NONE', *, *, #43757, .F. ) ;
#80893=EDGE_LOOP ( 'NONE', ( #9951, #77997, #73294, #51350 ) ) ;
#80913=VERTEX_POINT ( 'NONE', #48052 ) ;
#80956=VECTOR ( 'NONE', #1547, 1000.000000000000000 ) ;
#80983=EDGE_LOOP ( 'NONE', ( #15324, #56917, #16585, #81311 ) ) ;
#81018=PLANE ( 'NONE',  #26717 ) ;
#81024=CARTESIAN_POINT ( 'NONE',  ( 4.665904304751416087E-15, 44.45000000000000284, -38.10000000000000142 ) ) ;
#81037=EDGE_CURVE ( 'NONE', #17490, #5834, #89765, .T. ) ;
#81069=FACE_OUTER_BOUND ( 'NONE', #75428, .T. ) ;
#81125=CARTESIAN_POINT ( 'NONE',  ( 0.000000000000000000, 44.45000000000000284, 0.000000000000000000 ) ) ;
#81144=ORIENTED_EDGE ( 'NONE', *, *, #365, .F. ) ;
#81162=ORIENTED_EDGE ( 'NONE', *, *, #72049, .T. ) ;
#81166=ORIENTED_EDGE ( 'NONE', *, *, #51185, .T. ) ;
#81168=EDGE_CURVE ( 'NONE', #31479, #45956, #15604, .T. ) ;
#81180=AXIS2_PLACEMENT_3D ( 'NONE', #14462, #69867, #61247 ) ;
#81182=LINE ( 'NONE', #18930, #5058 ) ;
#81199=ORIENTED_EDGE ( 'NONE', *, *, #89384, .F. ) ;
#81229=ORIENTED_EDGE ( 'NONE', *, *, #70350, .T. ) ;
#81240=CARTESIAN_POINT ( 'NONE',  ( 121.8072289635121166, 60.27442714569195914, -46.99064742675564332 ) ) ;
#81274=ADVANCED_FACE ( 'NONE', ( #32091 ), #4846, .F. ) ;
#81295=ADVANCED_FACE ( 'NONE', ( #59787 ), #59347, .T. ) ;
#81296=EDGE_CURVE ( 'NONE', #22712, #85960, #8347, .T. ) ;
#81310=CARTESIAN_POINT ( 'NONE',  ( -141.3509999999999991, 20.32000000000000028, 141.3509999999999991 ) ) ;
#81311=ORIENTED_EDGE ( 'NONE', *, *, #29177, .F. ) ;
#81320=CARTESIAN_POINT ( 'NONE',  ( 123.4696824136382105, 0.000000000000000000, -179.8898777604649979 ) ) ;
#81344=DIRECTION ( 'NONE',  ( 0.000000000000000000, 1.000000000000000000, 0.000000000000000000 ) ) ;
#81357=CARTESIAN_POINT ( 'NONE',  ( -194.1576000000000022, 101.5999999999999943, -9.525000000000000355 ) ) ;
#81376=CARTESIAN_POINT ( 'NONE',  ( -3.174999999999644995, 24.56180297284579694, 33.98325472291465132 ) ) ;
#81419=CARTESIAN_POINT ( 'NONE',  ( -75.61066417432020614, 20.32000000000000028, 189.7379999999999995 ) ) ;
#81420=VECTOR ( 'NONE', #61252, 1000.000000000000000 ) ;
#81432=CARTESIAN_POINT ( 'NONE',  ( 7.047591375350159559, 93.11510580299035666, 130.3656419271163998 ) ) ;
#81504=VERTEX_POINT ( 'NONE', #58783 ) ;
#81544=DIRECTION ( 'NONE',  ( 0.9347835805883506488, 0.000000000000000000, 0.3552177606235679130 ) ) ;
#81591=CARTESIAN_POINT ( 'NONE',  ( -110.3182612653083794, 61.98564117580777122, 69.81941546282760669 ) ) ;
#81620=CARTESIAN_POINT ( 'NONE',  ( -4.504857172154159706, 70.67494150456570878, 130.4783009322840996 ) ) ;
#81655=FACE_OUTER_BOUND ( 'NONE', #4965, .T. ) ;
#81671=DIRECTION ( 'NONE',  ( 0.000000000000000000, 0.000000000000000000, 1.000000000000000000 ) ) ;
#81684=ORIENTED_EDGE ( 'NONE', *, *, #70350, .F. ) ;
#81727=DIRECTION ( 'NONE',  ( 0.000000000000000000, 0.000000000000000000, 1.000000000000000000 ) ) ;
#81751=ORIENTED_EDGE ( 'NONE', *, *, #38105, .T. ) ;
#81756=LINE ( 'NONE', #19507, #47957 ) ;
#81784=CARTESIAN_POINT ( 'NONE',  ( -148.0533267522759786, 20.32000000000000028, -160.2664750769289697 ) ) ;
#81794=FACE_OUTER_BOUND ( 'NONE', #4853, .T. ) ;
#81795=CARTESIAN_POINT ( 'NONE',  ( 7.584119442562257341, 72.36170844776167144, 130.3354891464173306 ) ) ;
#81803=ADVANCED_FACE ( 'NONE', ( #83284 ), #1957, .F. ) ;
#81809=CARTESIAN_POINT ( 'NONE',  ( -179.8898777604649979, 101.5999999999999943, 122.9960808104842016 ) ) ;
#81816=ORIENTED_EDGE ( 'NONE', *, *, #26112, .T. ) ;
#81844=AXIS2_PLACEMENT_3D ( 'NONE', #66966, #59248, #31992 ) ;
#81852=DIRECTION ( 'NONE',  ( 1.000000000000000000, 0.000000000000000000, 2.108231265501709878E-16 ) ) ;
#81854=DIRECTION ( 'NONE',  ( 0.000000000000000000, -1.000000000000000000, 0.000000000000000000 ) ) ;
#81871=CARTESIAN_POINT ( 'NONE',  ( 10.48278874474372380, 89.71962060600694144, 130.1344814326622554 ) ) ;
#81965=DIRECTION ( 'NONE',  ( -1.000000000000000000, 0.000000000000000000, 0.000000000000000000 ) ) ;
#81968=CARTESIAN_POINT ( 'NONE',  ( 0.000000000000000000, 114.2999999999999972, -9.525000000000000355 ) ) ;
#82011=VERTEX_POINT ( 'NONE', #74681 ) ;
#82016=FACE_OUTER_BOUND ( 'NONE', #46127, .T. ) ;
#82038=CARTESIAN_POINT ( 'NONE',  ( -109.5132684488906705, 57.82504450241307126, 71.07540765708218089 ) ) ;
#82040=ORIENTED_EDGE ( 'NONE', *, *, #30193, .T. ) ;
#82053=ORIENTED_EDGE ( 'NONE', *, *, #50743, .T. ) ;
#82097=VECTOR ( 'NONE', #67, 1000.000000000000000 ) ;
#82117=LINE ( 'NONE', #33933, #27011 ) ;
#82141=DIRECTION ( 'NONE',  ( -2.913971193241881161E-15, 0.000000000000000000, 1.000000000000000000 ) ) ;
#82145=VECTOR ( 'NONE', #8416, 1000.000000000000000 ) ;
#82182=CARTESIAN_POINT ( 'NONE',  ( 109.4081066450106619, 51.07333133673250103, 71.23720173749269691 ) ) ;
#82184=EDGE_LOOP ( 'NONE', ( #61446, #85903, #17559, #61131, #42966 ) ) ;
#82191=CARTESIAN_POINT ( 'NONE',  ( 12.69999999999999929, 82.54999999999999716, 129.9368274816650057 ) ) ;
#82231=VECTOR ( 'NONE', #3576, 1000.000000000000000 ) ;
#82250=CARTESIAN_POINT ( 'NONE',  ( 10.56149714719919075, 75.49700186538963464, 130.1281057863494652 ) ) ;
#82259=ORIENTED_EDGE ( 'NONE', *, *, #37826, .F. ) ;
#82279=ORIENTED_EDGE ( 'NONE', *, *, #72049, .F. ) ;
#82289=ORIENTED_EDGE ( 'NONE', *, *, #52340, .F. ) ;
#82294=LINE ( 'NONE', #26849, #1508 ) ;
#82298=CARTESIAN_POINT ( 'NONE',  ( -148.0533267522759786, 101.5999999999999943, -160.2664750769289697 ) ) ;
#82318=CIRCLE ( 'NONE', #56145, 9.524999999999998579 ) ;
#82323=DIRECTION ( 'NONE',  ( 0.000000000000000000, -1.000000000000000000, 0.000000000000000000 ) ) ;
#82324=ORIENTED_EDGE ( 'NONE', *, *, #84373, .F. ) ;
#82347=FACE_OUTER_BOUND ( 'NONE', #71144, .T. ) ;
#82350=DIRECTION ( 'NONE',  ( 0.000000000000000000, 0.000000000000000000, 1.000000000000000000 ) ) ;
#82393=CIRCLE ( 'NONE', #40291, 179.8898777604655095 ) ;
#82429=EDGE_CURVE ( 'NONE', #16666, #43971, #67760, .T. ) ;
#82435=CARTESIAN_POINT ( 'NONE',  ( 20.42678914444644889, 45.07398772557888122, 32.16741729433402242 ) ) ;
#82465=ORIENTED_EDGE ( 'NONE', *, *, #15464, .F. ) ;
#82485=AXIS2_PLACEMENT_3D ( 'NONE', #26365, #46784, #47235 ) ;
#82488=CARTESIAN_POINT ( 'NONE',  ( -113.3591856336701937, 69.18138141856444179, 64.76768199333514531 ) ) ;
#82513=CARTESIAN_POINT ( 'NONE',  ( -7.575738673516524635, 72.34850935353102841, 130.3362775872886061 ) ) ;
#82517=DIRECTION ( 'NONE',  ( 0.000000000000000000, 0.000000000000000000, -1.000000000000000000 ) ) ;
#82541=PLANE ( 'NONE',  #31825 ) ;
#82547=EDGE_CURVE ( 'NONE', #73595, #89539, #83644, .T. ) ;
#82553=DIRECTION ( 'NONE',  ( 0.000000000000000000, 1.000000000000000000, 0.000000000000000000 ) ) ;
#82571=CARTESIAN_POINT ( 'NONE',  ( -141.3509999999999991, 20.32000000000000028, 132.7150000000000034 ) ) ;
#82573=EDGE_CURVE ( 'NONE', #89203, #2756, #70010, .T. ) ;
#82595=ADVANCED_FACE ( 'NONE', ( #68663 ), #509, .F. ) ;
#82596=LINE ( 'NONE', #341, #61845 ) ;
#82612=DIRECTION ( 'NONE',  ( 0.7071067811865344721, 0.000000000000000000, 0.7071067811865604513 ) ) ;
#82622=LINE ( 'NONE', #63041, #83287 ) ;
#82627=DIRECTION ( 'NONE',  ( 0.000000000000000000, 1.000000000000000000, 0.000000000000000000 ) ) ;
#82641=LINE ( 'NONE', #69437, #132 ) ;
#82647=AXIS2_PLACEMENT_3D ( 'NONE', #68833, #67474, #39324 ) ;
#82659=LINE ( 'NONE', #49434, #89253 ) ;
#82698=CARTESIAN_POINT ( 'NONE',  ( 10.56818871369674717, 75.50703187974120567, 130.1275625430741627 ) ) ;
#82724=VERTEX_POINT ( 'NONE', #79521 ) ;
#82726=EDGE_LOOP ( 'NONE', ( #28573, #24938, #8662, #65812, #28285 ) ) ;
#82768=DIRECTION ( 'NONE',  ( 0.000000000000000000, -1.000000000000000000, 0.000000000000000000 ) ) ;
#82771=ORIENTED_EDGE ( 'NONE', *, *, #84262, .T. ) ;
#82779=CARTESIAN_POINT ( 'NONE',  ( -178.3658777604659917, 20.32000000000000028, 122.9960808104842016 ) ) ;
#82801=ORIENTED_EDGE ( 'NONE', *, *, #27023, .F. ) ;
#82803=CARTESIAN_POINT ( 'NONE',  ( 50.03799999999999670, 101.5999999999999943, 191.3008000794699797 ) ) ;
#82809=EDGE_CURVE ( 'NONE', #83014, #2756, #80655, .T. ) ;
#82849=CARTESIAN_POINT ( 'NONE',  ( -23.27731929905162289, 53.97500000000000142, 30.16249999999999076 ) ) ;
#82872=DIRECTION ( 'NONE',  ( 0.000000000000000000, 0.000000000000000000, 1.000000000000000000 ) ) ;
#82887=VECTOR ( 'NONE', #72387, 1000.000000000000000 ) ;
#82893=VECTOR ( 'NONE', #67527, 1000.000000000000000 ) ;
#82895=DIRECTION ( 'NONE',  ( 0.000000000000000000, 0.000000000000000000, 1.000000000000000000 ) ) ;
#82916=ORIENTED_EDGE ( 'NONE', *, *, #36415, .F. ) ;
#82929=CARTESIAN_POINT ( 'NONE',  ( -125.9554655030170949, 66.44187932044889067, 34.35260500423783725 ) ) ;
#82934=ORIENTED_EDGE ( 'NONE', *, *, #49606, .T. ) ;
#82956=CARTESIAN_POINT ( 'NONE',  ( -10.54081325544818704, 75.46611757261116793, 130.1297836194693218 ) ) ;
#82976=LINE ( 'NONE', #12123, #24836 ) ;
#82983=LINE ( 'NONE', #74803, #8647 ) ;
#82988=ORIENTED_EDGE ( 'NONE', *, *, #461, .T. ) ;
#82991=CARTESIAN_POINT ( 'NONE',  ( -126.4481529151155996, 44.45000000000000284, 32.49205688096009936 ) ) ;
#83014=VERTEX_POINT ( 'NONE', #61281 ) ;
#83041=CARTESIAN_POINT ( 'NONE',  ( -179.8898777604655095, 20.32000000000000028, 114.2999999999999972 ) ) ;
#83094=VECTOR ( 'NONE', #53304, 1000.000000000000000 ) ;
#83096=LINE ( 'NONE', #20849, #65554 ) ;
#83106=CARTESIAN_POINT ( 'NONE',  ( -33.98325472291465132, 17.78000000000000114, -3.174999999999764899 ) ) ;
#83141=CARTESIAN_POINT ( 'NONE',  ( 6.301291950802956343, 71.51565506672721995, 130.4043135987251674 ) ) ;
#83154=ORIENTED_EDGE ( 'NONE', *, *, #77414, .F. ) ;
#83165=CARTESIAN_POINT ( 'NONE',  ( 148.0533267522752112, 101.5999999999999943, 160.2664750769284865 ) ) ;
#83170=CIRCLE ( 'NONE', #3398, 7.874000000000227928 ) ;
#83179=CIRCLE ( 'NONE', #7756, 7.874000000000227928 ) ;
#83196=ORIENTED_EDGE ( 'NONE', *, *, #68094, .T. ) ;
#83240=ORIENTED_EDGE ( 'NONE', *, *, #52645, .T. ) ;
#83246=VECTOR ( 'NONE', #27154, 1000.000000000000000 ) ;
#83248=ORIENTED_EDGE ( 'NONE', *, *, #6824, .T. ) ;
#83255=LINE ( 'NONE', #70062, #80328 ) ;
#83284=FACE_OUTER_BOUND ( 'NONE', #87484, .T. ) ;
#83287=VECTOR ( 'NONE', #47607, 1000.000000000000000 ) ;
#83300=DIRECTION ( 'NONE',  ( 0.000000000000000000, -1.000000000000000000, 0.000000000000000000 ) ) ;
#83343=EDGE_LOOP ( 'NONE', ( #42885, #8516 ) ) ;
#83344=EDGE_CURVE ( 'NONE', #11013, #15725, #53326, .T. ) ;
#83353=ORIENTED_EDGE ( 'NONE', *, *, #30199, .F. ) ;
#83367=CARTESIAN_POINT ( 'NONE',  ( -119.9082588554310576, 74.59549379520217371, 51.64190430363700557 ) ) ;
#83369=ORIENTED_EDGE ( 'NONE', *, *, #39119, .T. ) ;
#83388=DIRECTION ( 'NONE',  ( 2.301579500234999682E-14, 0.000000000000000000, -1.000000000000000000 ) ) ;
#83390=CARTESIAN_POINT ( 'NONE',  ( -10.55295613787796327, 75.48422888499150929, 130.1287987652872857 ) ) ;
#83413=CARTESIAN_POINT ( 'NONE',  ( -179.8898777604649979, 20.32000000000000028, 122.9960808104842016 ) ) ;
#83457=ADVANCED_FACE ( 'NONE', ( #68787 ), #54221, .T. ) ;
#83461=EDGE_CURVE ( 'NONE', #378, #17490, #74116, .T. ) ;
#83470=CIRCLE ( 'NONE', #24018, 7.873999999999991672 ) ;
#83488=ORIENTED_EDGE ( 'NONE', *, *, #3216, .T. ) ;
#83505=CARTESIAN_POINT ( 'NONE',  ( 109.6365420697629531, 49.23178009149190615, 70.88510413816129585 ) ) ;
#83516=FACE_OUTER_BOUND ( 'NONE', #3707, .T. ) ;
#83525=ADVANCED_BREP_SHAPE_REPRESENTATION ( '', ( #50495, #50656 ), #10078 ) ;
#83556=DIRECTION ( 'NONE',  ( 0.000000000000000000, 0.000000000000000000, 1.000000000000000000 ) ) ;
#83571=EDGE_LOOP ( 'NONE', ( #65938, #44709, #65150, #55193 ) ) ;
#83590=CARTESIAN_POINT ( 'NONE',  ( 119.5843592605237120, 52.73749999999999716, -52.38749999999991758 ) ) ;
#83644=LINE ( 'NONE', #89110, #5236 ) ;
#83652=EDGE_CURVE ( 'NONE', #77712, #40497, #9139, .T. ) ;
#83654=EDGE_CURVE ( 'NONE', #42800, #13980, #18729, .T. ) ;
#83668=ORIENTED_EDGE ( 'NONE', *, *, #46792, .T. ) ;
#83688=DIRECTION ( 'NONE',  ( 0.000000000000000000, 0.000000000000000000, -1.000000000000000000 ) ) ;
#83711=ORIENTED_EDGE ( 'NONE', *, *, #28563, .T. ) ;
#83761=DIRECTION ( 'NONE',  ( -1.000000000000000000, 0.000000000000000000, 0.000000000000000000 ) ) ;
#83762=VECTOR ( 'NONE', #40085, 1000.000000000000000 ) ;
#83771=LINE ( 'NONE', #8356, #80956 ) ;
#83822=CARTESIAN_POINT ( 'NONE',  ( -117.7484220338073300, 73.87720319330706786, 56.41025224552601003 ) ) ;
#83848=CARTESIAN_POINT ( 'NONE',  ( 183.5150000000000148, 53.21300000000000097, 41.63456447661469895 ) ) ;
#83849=CARTESIAN_POINT ( 'NONE',  ( 50.03799999999999670, 101.5999999999999943, 178.6098374884404905 ) ) ;
#83907=CARTESIAN_POINT ( 'NONE',  ( -11.58988490044493957, 87.75625135835190349, 130.0406260143446673 ) ) ;
#83909=DIRECTION ( 'NONE',  ( 2.505701470911820065E-15, 0.000000000000000000, 1.000000000000000000 ) ) ;
#83920=VERTEX_POINT ( 'NONE', #13265 ) ;
#83930=CIRCLE ( 'NONE', #46209, 20.63750000000000284 ) ;
#83955=CARTESIAN_POINT ( 'NONE',  ( 17.77918093722091442, 65.59530694298135245, 33.71461300154621910 ) ) ;
#83969=VERTEX_POINT ( 'NONE', #15957 ) ;
#83970=CARTESIAN_POINT ( 'NONE',  ( -215.9000000000000057, 0.000000000000000000, -45.33899999999999864 ) ) ;
#84040=CARTESIAN_POINT ( 'NONE',  ( 124.8317794719591802, 47.79294463634281698, -38.23516268198856949 ) ) ;
#84064=DIRECTION ( 'NONE',  ( 2.108231265501709878E-16, 0.000000000000000000, -1.000000000000000000 ) ) ;
#84071=CARTESIAN_POINT ( 'NONE',  ( 126.2502385374383636, 64.84973863628553659, 33.25376590429844725 ) ) ;
#84147=EDGE_LOOP ( 'NONE', ( #14321, #17104, #7465, #37299 ) ) ;
#84162=VERTEX_POINT ( 'NONE', #79983 ) ;
#84195=CARTESIAN_POINT ( 'NONE',  ( -215.9000000000000057, 101.5999999999999943, -41.27499999999999858 ) ) ;
#84205=CARTESIAN_POINT ( 'NONE',  ( 50.03799999999999670, 20.32000000000000028, 206.3750000000000000 ) ) ;
#84238=ORIENTED_EDGE ( 'NONE', *, *, #14332, .T. ) ;
#84262=EDGE_CURVE ( 'NONE', #65247, #11013, #5450, .T. ) ;
#84264=DIRECTION ( 'NONE',  ( -2.301579500234999682E-14, 0.000000000000000000, 1.000000000000000000 ) ) ;
#84279=CARTESIAN_POINT ( 'NONE',  ( -124.2065287780126965, 71.69490183950009055, 40.21978412304718375 ) ) ;
#84310=DIRECTION ( 'NONE',  ( 0.000000000000000000, 1.000000000000000000, 0.000000000000000000 ) ) ;
#84373=EDGE_CURVE ( 'NONE', #10389, #6370, #418, .T. ) ;
#84394=VERTEX_POINT ( 'NONE', #49445 ) ;
#84402=VERTEX_POINT ( 'NONE', #34027 ) ;
#84411=CARTESIAN_POINT ( 'NONE',  ( 10.79358099957683237, 68.92650925838135834, 36.56259317987532143 ) ) ;
#84413=CARTESIAN_POINT ( 'NONE',  ( 131.3179999999999836, 53.97500000000000142, 71.43750000000000000 ) ) ;
#84427=ORIENTED_EDGE ( 'NONE', *, *, #45571, .T. ) ;
#84434=DIRECTION ( 'NONE',  ( 0.000000000000000000, -1.000000000000000000, 0.000000000000000000 ) ) ;
#84446=VECTOR ( 'NONE', #67019, 1000.000000000000000 ) ;
#84485=ORIENTED_EDGE ( 'NONE', *, *, #44068, .T. ) ;
#84495=LINE ( 'NONE', #49925, #85709 ) ;
#84530=CARTESIAN_POINT ( 'NONE',  ( 124.4845670069425836, 71.14632460481045939, 39.35078757465099386 ) ) ;
#84557=DIRECTION ( 'NONE',  ( 0.000000000000000000, 0.000000000000000000, -1.000000000000000000 ) ) ;
#84589=VERTEX_POINT ( 'NONE', #78542 ) ;
#84601=AXIS2_PLACEMENT_3D ( 'NONE', #31342, #65855, #51770 ) ;
#84617=EDGE_LOOP ( 'NONE', ( #9679, #59546, #61515, #74536 ) ) ;
#84619=AXIS2_PLACEMENT_3D ( 'NONE', #55127, #69242, #635 ) ;
#84648=LINE ( 'NONE', #63744, #50103 ) ;
#84701=VERTEX_POINT ( 'NONE', #76172 ) ;
#84728=CARTESIAN_POINT ( 'NONE',  ( -126.1761431753821370, 65.30360745155232394, 33.53545494772723146 ) ) ;
#84747=ORIENTED_EDGE ( 'NONE', *, *, #74422, .F. ) ;
#84752=DIRECTION ( 'NONE',  ( 0.000000000000000000, -1.000000000000000000, 0.000000000000000000 ) ) ;
#84781=EDGE_CURVE ( 'NONE', #47365, #57167, #82117, .T. ) ;
#84804=LINE ( 'NONE', #37084, #56719 ) ;
#84823=CARTESIAN_POINT ( 'NONE',  ( 108.8673596973266058, 37.33800000000000097, 50.79999999999999716 ) ) ;
#84837=CARTESIAN_POINT ( 'NONE',  ( -110.3179153611602032, 45.92529307294462626, 69.82078934106453971 ) ) ;
#84857=DIRECTION ( 'NONE',  ( -1.000000000000000000, 0.000000000000000000, 0.000000000000000000 ) ) ;
#84880=AXIS2_PLACEMENT_3D ( 'NONE', #21511, #62818, #55532 ) ;
#84883=EDGE_CURVE ( 'NONE', #8973, #35850, #80600, .T. ) ;
#84885=EDGE_CURVE ( 'NONE', #52538, #51892, #31348, .T. ) ;
#84931=PLANE ( 'NONE',  #34431 ) ;
#84933=CARTESIAN_POINT ( 'NONE',  ( -22.10999473297549045, 47.99418752069149008, 31.03039529537862506 ) ) ;
#84972=DIRECTION ( 'NONE',  ( 8.881784197001251337E-16, 0.000000000000000000, 1.000000000000000000 ) ) ;
#84974=ORIENTED_EDGE ( 'NONE', *, *, #68593, .T. ) ;
#85000=CIRCLE ( 'NONE', #8077, 7.937500000000000000 ) ;
#85017=DIRECTION ( 'NONE',  ( -1.514143847546115117E-15, 0.000000000000000000, 1.000000000000000000 ) ) ;
#85018=LINE ( 'NONE', #8709, #68898 ) ;
#85042=EDGE_CURVE ( 'NONE', #36552, #57278, #70638, .T. ) ;
#85066=EDGE_CURVE ( 'NONE', #55433, #6845, #25574, .T. ) ;
#85089=CARTESIAN_POINT ( 'NONE',  ( 10.77469451420456359, 75.82559005915315709, 130.1106627578315340 ) ) ;
#85120=CARTESIAN_POINT ( 'NONE',  ( 6.299229072587491096, 93.57981503384465327, 130.4040377106156257 ) ) ;
#85129=PLANE ( 'NONE',  #33183 ) ;
#85141=CARTESIAN_POINT ( 'NONE',  ( 183.5150000000000148, 21.46300000000000097, 59.96543552338529537 ) ) ;
#85148=EDGE_LOOP ( 'NONE', ( #36230, #45467, #33864, #83154 ) ) ;
#85155=ADVANCED_FACE ( 'NONE', ( #66936 ), #38775, .F. ) ;
#85177=EDGE_CURVE ( 'NONE', #10881, #7937, #40092, .T. ) ;
#85180=VERTEX_POINT ( 'NONE', #24711 ) ;
#85204=EDGE_CURVE ( 'NONE', #76607, #66477, #12551, .T. ) ;
#85219=LINE ( 'NONE', #8450, #69841 ) ;
#85260=CARTESIAN_POINT ( 'NONE',  ( -4.908820038593109558, 94.26296816967553127, 130.4636833037901340 ) ) ;
#85292=CARTESIAN_POINT ( 'NONE',  ( -109.7026200886537879, 48.81775394257228839, 70.78279810002825911 ) ) ;
#85312=DIRECTION ( 'NONE',  ( 1.000000000000000000, 0.000000000000000000, 0.000000000000000000 ) ) ;
#85326=ORIENTED_EDGE ( 'NONE', *, *, #51911, .T. ) ;
#85346=EDGE_CURVE ( 'NONE', #88226, #52020, #61875, .T. ) ;
#85375=CARTESIAN_POINT ( 'NONE',  ( 0.000000000000000000, 114.2999999999999972, 0.000000000000000000 ) ) ;
#85383=DIRECTION ( 'NONE',  ( 0.000000000000000000, 0.000000000000000000, -1.000000000000000000 ) ) ;
#85429=CARTESIAN_POINT ( 'NONE',  ( 123.6120034158685286, 72.65141698275766657, 42.01243221415964513 ) ) ;
#85457=DIRECTION ( 'NONE',  ( 0.000000000000000000, -1.000000000000000000, 0.000000000000000000 ) ) ;
#85463=AXIS2_PLACEMENT_3D ( 'NONE', #9542, #85861, #1839 ) ;
#85535=DIRECTION ( 'NONE',  ( -1.000000000000000000, 0.000000000000000000, -2.108231265501709878E-16 ) ) ;
#85565=VECTOR ( 'NONE', #10183, 1000.000000000000000 ) ;
#85605=ADVANCED_FACE ( 'NONE', ( #66825 ), #24605, .F. ) ;
#85620=CARTESIAN_POINT ( 'NONE',  ( -126.9896596436628755, 56.80590851577779432, 30.30816834133878146 ) ) ;
#85626=VERTEX_POINT ( 'NONE', #86391 ) ;
#85632=EDGE_CURVE ( 'NONE', #34694, #34850, #25493, .T. ) ;
#85646=DIRECTION ( 'NONE',  ( 0.000000000000000000, 0.000000000000000000, 1.000000000000000000 ) ) ;
#85652=AXIS2_PLACEMENT_3D ( 'NONE', #77031, #30219, #57463 ) ;
#85663=CARTESIAN_POINT ( 'NONE',  ( 50.03799999999999670, 0.000000000000000000, 206.3750000000000000 ) ) ;
#85665=CIRCLE ( 'NONE', #18855, 20.63750000000000284 ) ;
#85709=VECTOR ( 'NONE', #50375, 1000.000000000000000 ) ;
#85736=CARTESIAN_POINT ( 'NONE',  ( 183.5150000000000148, 37.33800000000000097, 32.46912895322940074 ) ) ;
#85754=CARTESIAN_POINT ( 'NONE',  ( 15.05032694871533927, 67.26578276466975126, 35.00684828750966204 ) ) ;
#85776=CARTESIAN_POINT ( 'NONE',  ( 196.2150000000000034, 43.68799999999999528, 57.14999999999999858 ) ) ;
#85781=ORIENTED_EDGE ( 'NONE', *, *, #51084, .T. ) ;
#85789=VECTOR ( 'NONE', #67812, 1000.000000000000000 ) ;
#85793=ORIENTED_EDGE ( 'NONE', *, *, #86750, .T. ) ;
#85797=CARTESIAN_POINT ( 'NONE',  ( 163.0822201311030142, 101.5999999999999943, -75.92468371870729982 ) ) ;
#85806=ORIENTED_EDGE ( 'NONE', *, *, #59061, .T. ) ;
#85820=FACE_OUTER_BOUND ( 'NONE', #41961, .T. ) ;
#85822=EDGE_LOOP ( 'NONE', ( #70442, #44976, #51661, #38019 ) ) ;
#85838=CARTESIAN_POINT ( 'NONE',  ( 125.0906544762830066, 49.12084779284757019, -37.37934391051621219 ) ) ;
#85842=CARTESIAN_POINT ( 'NONE',  ( -141.3509999999999991, 101.5999999999999943, -141.3509999999999991 ) ) ;
#85858=CARTESIAN_POINT ( 'NONE',  ( 0.000000000000000000, 44.45000000000000284, 0.000000000000000000 ) ) ;
#85861=DIRECTION ( 'NONE',  ( -1.000000000000000000, 0.000000000000000000, 0.000000000000000000 ) ) ;
#85871=DIRECTION ( 'NONE',  ( 0.000000000000000000, -1.000000000000000000, 0.000000000000000000 ) ) ;
#85903=ORIENTED_EDGE ( 'NONE', *, *, #43090, .T. ) ;
#85925=ORIENTED_EDGE ( 'NONE', *, *, #5216, .F. ) ;
#85934=SURFACE_SIDE_STYLE ('',( #30501 ) ) ;
#85960=VERTEX_POINT ( 'NONE', #2281 ) ;
#85968=ORIENTED_EDGE ( 'NONE', *, *, #63926, .F. ) ;
#86007=CARTESIAN_POINT ( 'NONE',  ( 3.230156947913894072, 94.83977257127416749, 130.5163774324635142 ) ) ;
#86028=LINE ( 'NONE', #85141, #82887 ) ;
#86052=DIRECTION ( 'NONE',  ( 0.000000000000000000, 0.000000000000000000, 1.000000000000000000 ) ) ;
#86063=ORIENTED_EDGE ( 'NONE', *, *, #31166, .T. ) ;
#86065=AXIS2_PLACEMENT_3D ( 'NONE', #48708, #89185, #69631 ) ;
#86070=DIRECTION ( 'NONE',  ( 1.000000000000000000, 0.000000000000000000, -6.982966722218760189E-15 ) ) ;
#86133=ADVANCED_FACE ( 'NONE', ( #3603, #87617 ), #80820, .T. ) ;
#86135=CARTESIAN_POINT ( 'NONE',  ( -10.56631526105568142, 89.59577849103433778, 130.1277146807724421 ) ) ;
#86139=CARTESIAN_POINT ( 'NONE',  ( 126.8569334184371797, 48.66001727116653086, 30.85758840523601876 ) ) ;
#86150=ORIENTED_EDGE ( 'NONE', *, *, #39746, .T. ) ;
#86155=EDGE_CURVE ( 'NONE', #7552, #69846, #61944, .T. ) ;
#86173=DIRECTION ( 'NONE',  ( -1.000000000000000000, 0.000000000000000000, -1.531877379624855416E-14 ) ) ;
#86188=CARTESIAN_POINT ( 'NONE',  ( 131.3179999999999836, 53.97500000000000142, 30.16249999999999787 ) ) ;
#86195=DIRECTION ( 'NONE',  ( -1.000000000000000000, 0.000000000000000000, 6.982966722218760189E-15 ) ) ;
#86203=CARTESIAN_POINT ( 'NONE',  ( 31.75000000000000000, 24.56180297284579694, 3.174999999999999822 ) ) ;
#86209=VECTOR ( 'NONE', #26703, 1000.000000000000000 ) ;
#86238=CYLINDRICAL_SURFACE ( 'NONE', #3190, 218.1859999999999786 ) ;
#86294=CARTESIAN_POINT ( 'NONE',  ( 118.9099480661945165, 74.38787642755048068, 53.90531644923896692 ) ) ;
#86296=ORIENTED_EDGE ( 'NONE', *, *, #68684, .T. ) ;
#86304=EDGE_CURVE ( 'NONE', #28720, #19975, #50402, .T. ) ;
#86308=LINE ( 'NONE', #73109, #16032 ) ;
#86323=PLANE ( 'NONE',  #84601 ) ;
#86370=PLANE ( 'NONE',  #69461 ) ;
#86391=CARTESIAN_POINT ( 'NONE',  ( 147.4575741623270062, 20.32000000000000028, -135.2444258376734183 ) ) ;
#86398=ADVANCED_FACE ( 'NONE', ( #1273 ), #22176, .T. ) ;
#86426=LINE ( 'NONE', #29658, #31770 ) ;
#86428=CARTESIAN_POINT ( 'NONE',  ( 147.4575741623265799, 20.32000000000000028, 135.2444258376725941 ) ) ;
#86448=CARTESIAN_POINT ( 'NONE',  ( 3.843954637141310471, 94.65618101170012721, 130.4993963320906403 ) ) ;
#86504=ORIENTED_EDGE ( 'NONE', *, *, #53244, .T. ) ;
#86529=CARTESIAN_POINT ( 'NONE',  ( -1.389269728106021784, 70.22718948829736973, 38.08091836535547969 ) ) ;
#86553=CARTESIAN_POINT ( 'NONE',  ( -194.1576000000000022, 0.000000000000000000, -45.33899999999999864 ) ) ;
#86570=ORIENTED_EDGE ( 'NONE', *, *, #14538, .F. ) ;
#86571=CARTESIAN_POINT ( 'NONE',  ( -194.1576000000000022, 101.5999999999999943, 146.9389999999999930 ) ) ;
#86592=EDGE_LOOP ( 'NONE', ( #16331, #68856, #48676, #75605 ) ) ;
#86594=DIRECTION ( 'NONE',  ( 0.000000000000000000, -1.000000000000000000, 0.000000000000000000 ) ) ;
#86605=VERTEX_POINT ( 'NONE', #80708 ) ;
#86606=ORIENTED_EDGE ( 'NONE', *, *, #70625, .F. ) ;
#86618=ORIENTED_EDGE ( 'NONE', *, *, #12504, .F. ) ;
#86640=LINE ( 'NONE', #87085, #33844 ) ;
#86653=PLANE ( 'NONE',  #13409 ) ;
#86655=AXIS2_PLACEMENT_3D ( 'NONE', #81419, #81854, #68662 ) ;
#86696=CARTESIAN_POINT ( 'NONE',  ( 121.1771017092910796, 59.51425790832627172, -48.59044173555516011 ) ) ;
#86704=FACE_OUTER_BOUND ( 'NONE', #40094, .T. ) ;
#86742=CARTESIAN_POINT ( 'NONE',  ( 113.7708228275151470, 69.80903686419651422, 64.04023853347004547 ) ) ;
#86748=PLANE ( 'NONE',  #26580 ) ;
#86750=EDGE_CURVE ( 'NONE', #88991, #72189, #82393, .T. ) ;
#86756=LINE ( 'NONE', #46275, #1579 ) ;
#86760=DIRECTION ( 'NONE',  ( 0.000000000000000000, 0.000000000000000000, 1.000000000000000000 ) ) ;
#86802=ORIENTED_EDGE ( 'NONE', *, *, #10397, .F. ) ;
#86815=AXIS2_PLACEMENT_3D ( 'NONE', #45440, #66344, #78682 ) ;
#86821=CARTESIAN_POINT ( 'NONE',  ( 173.9900000000000091, 20.32000000000000028, -71.37400000000000944 ) ) ;
#86848=AXIS2_PLACEMENT_3D ( 'NONE', #1354, #49921, #70850 ) ;
#86861=PLANE ( 'NONE',  #33498 ) ;
#86892=CARTESIAN_POINT ( 'NONE',  ( 131.3179999999999836, 37.33800000000000097, 50.79999999999999716 ) ) ;
#86913=DIRECTION ( 'NONE',  ( 1.000000000000000000, 0.000000000000000000, 0.000000000000000000 ) ) ;
#86916=ORIENTED_EDGE ( 'NONE', *, *, #61811, .F. ) ;
#86918=EDGE_CURVE ( 'NONE', #30970, #39820, #62482, .T. ) ;
#86922=AXIS2_PLACEMENT_3D ( 'NONE', #37375, #30999, #58692 ) ;
#86947=DIRECTION ( 'NONE',  ( 0.000000000000000000, -1.000000000000000000, 0.000000000000000000 ) ) ;
#86956=DIRECTION ( 'NONE',  ( 1.000000000000000000, 0.000000000000000000, 0.000000000000000000 ) ) ;
#86962=ADVANCED_FACE ( 'NONE', ( #73198 ), #60923, .F. ) ;
#87001=ORIENTED_EDGE ( 'NONE', *, *, #43757, .T. ) ;
#87022=CARTESIAN_POINT ( 'NONE',  ( -10.20556736627216843, 90.12022208354639474, 130.1569092081103349 ) ) ;
#87033=VECTOR ( 'NONE', #77572, 1000.000000000000000 ) ;
#87038=ORIENTED_EDGE ( 'NONE', *, *, #76638, .F. ) ;
#87076=CARTESIAN_POINT ( 'NONE',  ( 57.91199999999999903, 20.32000000000000028, 178.6098374884404905 ) ) ;
#87085=CARTESIAN_POINT ( 'NONE',  ( 108.8673596973266058, 37.33800000000000097, 42.86249999999999716 ) ) ;
#87100=ORIENTED_EDGE ( 'NONE', *, *, #27130, .T. ) ;
#87101=VECTOR ( 'NONE', #69543, 1000.000000000000000 ) ;
#87120=CARTESIAN_POINT ( 'NONE',  ( -194.1576000000000022, 101.5999999999999943, -45.33899999999999864 ) ) ;
#87141=ORIENTED_EDGE ( 'NONE', *, *, #32645, .T. ) ;
#87143=CARTESIAN_POINT ( 'NONE',  ( 120.3150230176155020, 57.65353451050373934, -50.68724638474388655 ) ) ;
#87144=ORIENTED_EDGE ( 'NONE', *, *, #80198, .F. ) ;
#87164=ORIENTED_EDGE ( 'NONE', *, *, #3859, .T. ) ;
#87166=VERTEX_POINT ( 'NONE', #69093 ) ;
#87179=DIRECTION ( 'NONE',  ( 0.9347835805883506488, 0.000000000000000000, 0.3552177606235679130 ) ) ;
#87183=FACE_OUTER_BOUND ( 'NONE', #44210, .T. ) ;
#87189=CARTESIAN_POINT ( 'NONE',  ( 121.7685547874556420, 74.27669327741411109, 47.08841425960243754 ) ) ;
#87257=( NAMED_UNIT ( * ) PLANE_ANGLE_UNIT ( ) SI_UNIT ( $, .RADIAN. ) );
#87264=ORIENTED_EDGE ( 'NONE', *, *, #77414, .T. ) ;
#87270=ORIENTED_EDGE ( 'NONE', *, *, #88763, .F. ) ;
#87272=DIRECTION ( 'NONE',  ( 0.000000000000000000, -1.000000000000000000, 0.000000000000000000 ) ) ;
#87279=ADVANCED_FACE ( 'NONE', ( #49521 ), #63619, .F. ) ;
#87300=DIRECTION ( 'NONE',  ( 0.000000000000000000, -1.000000000000000000, 0.000000000000000000 ) ) ;
#87301=CARTESIAN_POINT ( 'NONE',  ( 183.5150000000000148, 53.21300000000000097, 41.63456447661469895 ) ) ;
#87309=CARTESIAN_POINT ( 'NONE',  ( -194.1576000000000022, 101.5999999999999943, 146.9389999999999930 ) ) ;
#87357=DIRECTION ( 'NONE',  ( 0.000000000000000000, -1.000000000000000000, 0.000000000000000000 ) ) ;
#87382=ORIENTED_EDGE ( 'NONE', *, *, #42373, .F. ) ;
#87400=AXIS2_PLACEMENT_3D ( 'NONE', #42433, #36088, #13410 ) ;
#87402=DIRECTION ( 'NONE',  ( 0.000000000000000000, -1.000000000000000000, 0.000000000000000000 ) ) ;
#87408=CARTESIAN_POINT ( 'NONE',  ( -9.469228445121002480, 69.24107684194999024, 36.91068001385391995 ) ) ;
#87417=VECTOR ( 'NONE', #37822, 1000.000000000000000 ) ;
#87425=ORIENTED_EDGE ( 'NONE', *, *, #20202, .T. ) ;
#87439=EDGE_CURVE ( 'NONE', #47090, #52633, #31320, .T. ) ;
#87483=CARTESIAN_POINT ( 'NONE',  ( -55.11501535285000131, 0.000000000000000000, 183.9403141659174992 ) ) ;
#87484=EDGE_LOOP ( 'NONE', ( #39211, #67895, #85806, #35532 ) ) ;
#87492=ORIENTED_EDGE ( 'NONE', *, *, #34080, .F. ) ;
#87494=ORIENTED_EDGE ( 'NONE', *, *, #87865, .T. ) ;
#87506=DIRECTION ( 'NONE',  ( 1.000000000000000000, 0.000000000000000000, 1.531877379624855416E-14 ) ) ;
#87553=DIRECTION ( 'NONE',  ( 0.000000000000000000, 0.000000000000000000, 1.000000000000000000 ) ) ;
#87585=CARTESIAN_POINT ( 'NONE',  ( 125.1886942929311743, 55.61998119543657282, -37.04958746976185324 ) ) ;
#87617=FACE_BOUND ( 'NONE', #5360, .T. ) ;
#87630=CARTESIAN_POINT ( 'NONE',  ( 115.2855339205388532, 71.76331869045601763, 61.27220515712456006 ) ) ;
#87634=ORIENTED_EDGE ( 'NONE', *, *, #68684, .F. ) ;
#87674=ORIENTED_EDGE ( 'NONE', *, *, #42373, .T. ) ;
#87678=ADVANCED_FACE ( 'NONE', ( #22639 ), #1291, .T. ) ;
#87695=ORIENTED_EDGE ( 'NONE', *, *, #21931, .T. ) ;
#87738=CARTESIAN_POINT ( 'NONE',  ( -186.2398777604655038, 101.5999999999999943, -12.69999999999999929 ) ) ;
#87742=CARTESIAN_POINT ( 'NONE',  ( 148.0533267522749838, 101.5999999999999943, -160.2664750769289697 ) ) ;
#87751=( LENGTH_UNIT ( ) NAMED_UNIT ( * ) SI_UNIT ( .MILLI., .METRE. ) );
#87759=AXIS2_PLACEMENT_3D ( 'NONE', #730, #70682, #76600 ) ;
#87836=DIRECTION ( 'NONE',  ( 0.000000000000000000, 0.000000000000000000, -1.000000000000000000 ) ) ;
#87838=ORIENTED_EDGE ( 'NONE', *, *, #85204, .T. ) ;
#87852=DIRECTION ( 'NONE',  ( 0.000000000000000000, -1.000000000000000000, 0.000000000000000000 ) ) ;
#87865=EDGE_CURVE ( 'NONE', #57278, #65312, #56219, .T. ) ;
#87901=ORIENTED_EDGE ( 'NONE', *, *, #55241, .F. ) ;
#87998=ORIENTED_EDGE ( 'NONE', *, *, #18090, .F. ) ;
#88021=CARTESIAN_POINT ( 'NONE',  ( 0.000000000000000000, 82.54999999999999716, 206.3750000000000000 ) ) ;
#88027=VECTOR ( 'NONE', #59780, 1000.000000000000000 ) ;
#88037=CARTESIAN_POINT ( 'NONE',  ( 124.6708304737691719, 58.27461704503507889, -38.75682993913466134 ) ) ;
#88054=DIRECTION ( 'NONE',  ( 1.000000000000000000, 0.000000000000000000, 0.000000000000000000 ) ) ;
#88061=ORIENTED_EDGE ( 'NONE', *, *, #8475, .F. ) ;
#88064=CARTESIAN_POINT ( 'NONE',  ( 75.61066417432020614, 20.32000000000000028, 177.0380000000000109 ) ) ;
#88084=DIRECTION ( 'NONE',  ( -1.000000000000000000, 0.000000000000000000, 0.000000000000000000 ) ) ;
#88086=CARTESIAN_POINT ( 'NONE',  ( 115.9477166093867595, 72.45386989696044111, 60.01166189639659621 ) ) ;
#88129=DIRECTION ( 'NONE',  ( 0.000000000000000000, -1.000000000000000000, 0.000000000000000000 ) ) ;
#88151=DIRECTION ( 'NONE',  ( 1.000000000000000000, 0.000000000000000000, 1.472650733923983947E-14 ) ) ;
#88167=AXIS2_PLACEMENT_3D ( 'NONE', #28507, #63486, #34881 ) ;
#88219=DIRECTION ( 'NONE',  ( 0.000000000000000000, 0.000000000000000000, 1.000000000000000000 ) ) ;
#88226=VERTEX_POINT ( 'NONE', #49309 ) ;
#88238=ORIENTED_EDGE ( 'NONE', *, *, #24595, .F. ) ;
#88246=DIRECTION ( 'NONE',  ( 0.000000000000000000, 0.000000000000000000, 1.000000000000000000 ) ) ;
#88251=AXIS2_PLACEMENT_3D ( 'NONE', #51915, #71956, #65129 ) ;
#88267=DIRECTION ( 'NONE',  ( 1.000000000000000000, 3.651563665954189830E-16, 0.000000000000000000 ) ) ;
#88274=DIRECTION ( 'NONE',  ( 0.000000000000000000, 0.000000000000000000, 1.000000000000000000 ) ) ;
#88301=ORIENTED_EDGE ( 'NONE', *, *, #1538, .F. ) ;
#88308=FACE_OUTER_BOUND ( 'NONE', #89198, .T. ) ;
#88311=EDGE_LOOP ( 'NONE', ( #82465, #47183, #55269, #20235 ) ) ;
#88327=PLANE ( 'NONE',  #32468 ) ;
#88341=FACE_OUTER_BOUND ( 'NONE', #47341, .T. ) ;
#88342=FACE_OUTER_BOUND ( 'NONE', #69433, .T. ) ;
#88365=DIRECTION ( 'NONE',  ( 0.000000000000000000, -1.000000000000000000, 0.000000000000000000 ) ) ;
#88383=ORIENTED_EDGE ( 'NONE', *, *, #37374, .F. ) ;
#88385=EDGE_CURVE ( 'NONE', #36180, #82011, #62267, .T. ) ;
#88388=VERTEX_POINT ( 'NONE', #18366 ) ;
#88421=CARTESIAN_POINT ( 'NONE',  ( -11.32599464014776558, 76.80063784493215451, 130.0638828588391220 ) ) ;
#88448=ORIENTED_EDGE ( 'NONE', *, *, #4980, .F. ) ;
#88481=DIRECTION ( 'NONE',  ( 0.000000000000000000, 0.000000000000000000, -1.000000000000000000 ) ) ;
#88492=CARTESIAN_POINT ( 'NONE',  ( 125.2163577468151914, 55.36712120389123015, -36.95591843739485682 ) ) ;
#88499=DIRECTION ( 'NONE',  ( -1.000000000000000000, -8.741913579725640327E-16, -2.913971193241879977E-15 ) ) ;
#88574=ADVANCED_FACE ( 'NONE', ( #19276 ), #26090, .F. ) ;
#88619=ORIENTED_EDGE ( 'NONE', *, *, #44132, .F. ) ;
#88656=AXIS2_PLACEMENT_3D ( 'NONE', #17711, #52634, #80395 ) ;
#88670=CIRCLE ( 'NONE', #1665, 179.8898777604655095 ) ;
#88709=CARTESIAN_POINT ( 'NONE',  ( 0.000000000000000000, 152.3879256507328250, 0.000000000000000000 ) ) ;
#88726=CARTESIAN_POINT ( 'NONE',  ( -194.1576000000000022, 101.5999999999999943, 114.2999999999999972 ) ) ;
#88738=ORIENTED_EDGE ( 'NONE', *, *, #43669, .T. ) ;
#88746=AXIS2_PLACEMENT_3D ( 'NONE', #16387, #65422, #22763 ) ;
#88763=EDGE_CURVE ( 'NONE', #121, #32410, #35573, .T. ) ;
#88825=CARTESIAN_POINT ( 'NONE',  ( -147.4575741623270062, 101.5999999999999943, 135.2444258376732193 ) ) ;
#88847=CARTESIAN_POINT ( 'NONE',  ( 0.000000000000000000, 11.42999999999999972, -154.1697486074984909 ) ) ;
#88868=CARTESIAN_POINT ( 'NONE',  ( -4.682505845377153975, 70.74451999347890307, 130.4720125505715487 ) ) ;
#88875=ADVANCED_FACE ( 'NONE', ( #23327 ), #9664, .T. ) ;
#88886=ORIENTED_EDGE ( 'NONE', *, *, #33476, .T. ) ;
#88899=ORIENTED_EDGE ( 'NONE', *, *, #74707, .T. ) ;
#88917=AXIS2_PLACEMENT_3D ( 'NONE', #13794, #55539, #70557 ) ;
#88919=FACE_OUTER_BOUND ( 'NONE', #35215, .T. ) ;
#88949=ORIENTED_EDGE ( 'NONE', *, *, #53298, .F. ) ;
#88950=CARTESIAN_POINT ( 'NONE',  ( 33.98325472291465132, 24.56180297284579694, 3.174999999999999822 ) ) ;
#88983=ORIENTED_EDGE ( 'NONE', *, *, #15771, .T. ) ;
#88991=VERTEX_POINT ( 'NONE', #9082 ) ;
#89017=DIRECTION ( 'NONE',  ( 0.000000000000000000, 0.000000000000000000, 1.000000000000000000 ) ) ;
#89032=EDGE_LOOP ( 'NONE', ( #12972, #86916, #40377, #45184, #68704, #50405, #29318, #34022, #53447, #67135, #77959 ) ) ;
#89033=LINE ( 'NONE', #7263, #42057 ) ;
#89041=LINE ( 'NONE', #19098, #44749 ) ;
#89044=CARTESIAN_POINT ( 'NONE',  ( 7.060824191845354036, 71.99373330411334848, 130.3649258744253245 ) ) ;
#89054=ORIENTED_EDGE ( 'NONE', *, *, #3523, .F. ) ;
#89055=EDGE_CURVE ( 'NONE', #27791, #19557, #1408, .T. ) ;
#89065=EDGE_CURVE ( 'NONE', #15997, #33670, #17672, .T. ) ;
#89079=EDGE_CURVE ( 'NONE', #82011, #17885, #60904, .T. ) ;
#89089=VERTEX_POINT ( 'NONE', #4035 ) ;
#89097=ORIENTED_EDGE ( 'NONE', *, *, #27474, .T. ) ;
#89109=ADVANCED_FACE ( 'NONE', ( #72644 ), #19346, .F. ) ;
#89110=CARTESIAN_POINT ( 'NONE',  ( -50.03799999999999670, 101.5999999999999943, 191.3008000794699797 ) ) ;
#89125=CARTESIAN_POINT ( 'NONE',  ( 12.62661858190509534, 84.14780334606243173, 129.9444360960973199 ) ) ;
#89128=AXIS2_PLACEMENT_3D ( 'NONE', #79260, #66040, #86956 ) ;
#89149=CARTESIAN_POINT ( 'NONE',  ( 183.5150000000000148, 21.46300000000000097, 41.63456447661474868 ) ) ;
#89165=DIRECTION ( 'NONE',  ( 0.000000000000000000, 0.000000000000000000, -1.000000000000000000 ) ) ;
#89185=DIRECTION ( 'NONE',  ( 0.000000000000000000, 1.000000000000000000, 0.000000000000000000 ) ) ;
#89198=EDGE_LOOP ( 'NONE', ( #40023, #459, #68895, #15023 ) ) ;
#89203=VERTEX_POINT ( 'NONE', #684 ) ;
#89222=DIRECTION ( 'NONE',  ( 0.000000000000000000, -1.000000000000000000, 0.000000000000000000 ) ) ;
#89247=EDGE_LOOP ( 'NONE', ( #55115, #10030, #29288, #39279, #18070, #34401, #72135, #24062, #31643, #58566, #63337, #37727, #87425, #88899, #6088, #28843, #58249, #25817 ) ) ;
#89253=VECTOR ( 'NONE', #62179, 1000.000000000000000 ) ;
#89289=CARTESIAN_POINT ( 'NONE',  ( -123.9668422125822218, 72.11824565187180269, 40.95437521977012807 ) ) ;
#89314=AXIS2_PLACEMENT_3D ( 'NONE', #51461, #72383, #51030 ) ;
#89316=CARTESIAN_POINT ( 'NONE',  ( -7.047141237186552054, 71.98459356607415316, 130.3656662584478170 ) ) ;
#89323=DIRECTION ( 'NONE',  ( 0.000000000000000000, 0.7071067811865120456, 0.7071067811865829889 ) ) ;
#89325=ORIENTED_EDGE ( 'NONE', *, *, #28156, .F. ) ;
#89338=DIRECTION ( 'NONE',  ( 0.000000000000000000, -1.000000000000000000, 0.000000000000000000 ) ) ;
#89384=EDGE_CURVE ( 'NONE', #34396, #22713, #31315, .T. ) ;
#89392=CARTESIAN_POINT ( 'NONE',  ( -3.174999999999644995, 17.78000000000000114, 33.98325472291465132 ) ) ;
#89428=CARTESIAN_POINT ( 'NONE',  ( -135.2444258376730204, 101.5999999999999943, 147.4575741623271767 ) ) ;
#89468=DIRECTION ( 'NONE',  ( 0.000000000000000000, 0.000000000000000000, 1.000000000000000000 ) ) ;
#89476=CARTESIAN_POINT ( 'NONE',  ( -123.4696824136392053, 20.32000000000000028, -179.8898777604655095 ) ) ;
#89494=LINE ( 'NONE', #21805, #18690 ) ;
#89501=DIRECTION ( 'NONE',  ( 0.000000000000000000, 0.000000000000000000, -1.000000000000000000 ) ) ;
#89502=ORIENTED_EDGE ( 'NONE', *, *, #86304, .T. ) ;
#89506=VECTOR ( 'NONE', #46887, 1000.000000000000000 ) ;
#89539=VERTEX_POINT ( 'NONE', #73549 ) ;
#89541=ORIENTED_EDGE ( 'NONE', *, *, #65557, .T. ) ;
#89551=CARTESIAN_POINT ( 'NONE',  ( -71.09939861440099662, 20.32000000000000028, 177.8662485265279827 ) ) ;
#89603=EDGE_CURVE ( 'NONE', #45956, #31479, #33412, .T. ) ;
#89635=ORIENTED_EDGE ( 'NONE', *, *, #78387, .T. ) ;
#89656=CARTESIAN_POINT ( 'NONE',  ( 0.000000000000000000, 0.000000000000000000, 0.000000000000000000 ) ) ;
#89679=DIRECTION ( 'NONE',  ( 2.108231265501709878E-16, 0.000000000000000000, -1.000000000000000000 ) ) ;
#89698=CARTESIAN_POINT ( 'NONE',  ( 160.2664750769284865, 0.000000000000000000, -148.0533267522753818 ) ) ;
#89710=EDGE_CURVE ( 'NONE', #21936, #59397, #72744, .T. ) ;
#89725=AXIS2_PLACEMENT_3D ( 'NONE', #21743, #9009, #64408 ) ;
#89744=CARTESIAN_POINT ( 'NONE',  ( -125.7768780727897564, 67.25820441060064070, 35.00145722608366583 ) ) ;
#89762=EDGE_LOOP ( 'NONE', ( #45362, #7237, #17108, #20927 ) ) ;
#89765=B_SPLINE_CURVE_WITH_KNOTS ( 'NONE', 3,
 ( #15805, #63490, #28981, #36695, #820, #64395, #44375, #28510, #72105, #15360, #35777, #23083, #43927, #36239, #51188, #56667, #56204, #83955, #21726, #85754, #71664, #63949, #49847, #84411, #37138, #64840, #9879, #1728, #30325, #50296, #77574, #49398 ),
 .UNSPECIFIED., .F., .F.,
 ( 4, 2, 2, 2, 2, 2, 2, 2, 2, 2, 2, 2, 2, 2, 2, 4 ),
 ( 0.01900920079883068256, 0.02107412302369412668, 0.02210658413612584527, 0.02313904524855756734, 0.02520396747342101146, 0.02623642858585272311, 0.02726888969828443129, 0.02933381192314784419, 0.03139873414801125362, 0.03552857859773811411, 0.03759350082260152354, 0.03965842304746493296, 0.04378826749719177958, 0.04585318972205519594, 0.04791811194691859843, 0.05204795639664543117 ),
 .UNSPECIFIED. ) ;
#89769=CARTESIAN_POINT ( 'NONE',  ( -11.41630163197954495, 76.98248777262077169, 130.0559678743007055 ) ) ;
#89872=EDGE_CURVE ( 'NONE', #5834, #2213, #35897, .T. ) ;
#89896=CARTESIAN_POINT ( 'NONE',  ( 173.9900000000000091, 52.73749999999999716, -36.51250000000000284 ) ) ;
ENDSEC;
END-ISO-10303-21;
